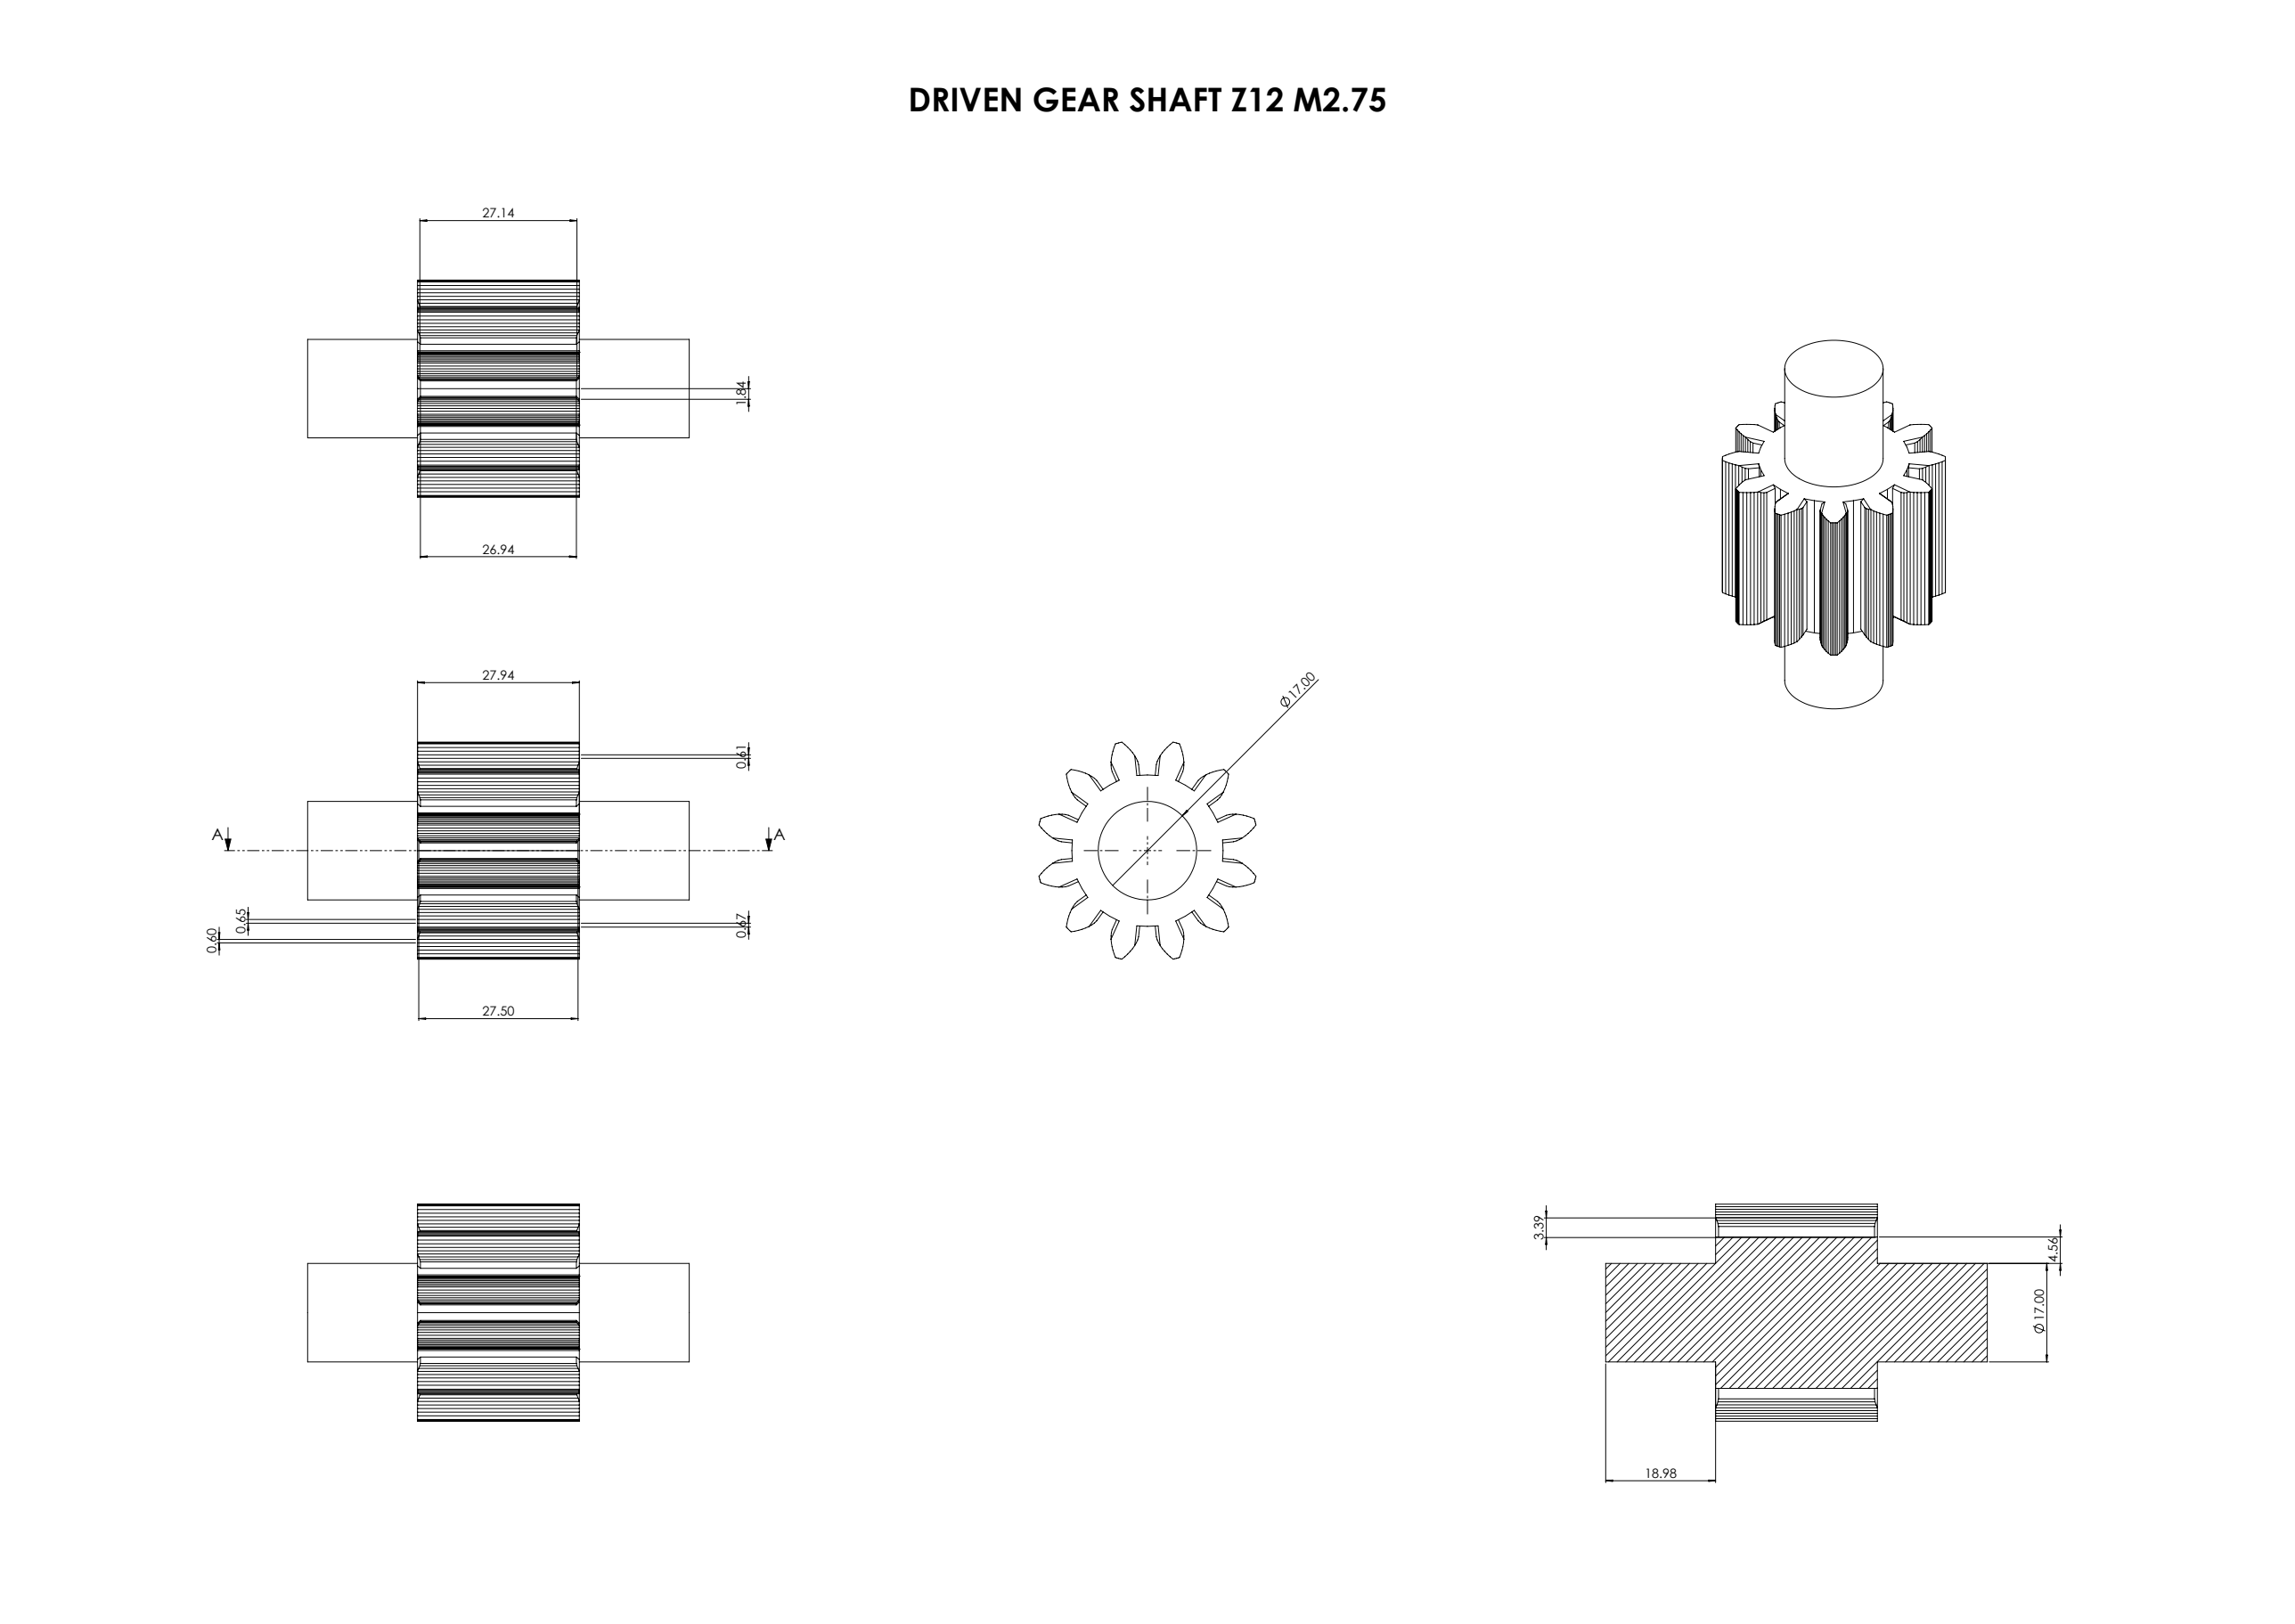
ISO-10303-21;
HEADER;
/* Generated by software containing ST-Developer
 * from STEP Tools, Inc. (www.steptools.com) 
 */

FILE_DESCRIPTION(
/* description */ (''),
/* implementation_level */ '2;1');

FILE_NAME(
/* name */ '05_Driven_Gear_Shaft_z12_m2.75.step',
/* time_stamp */ '2026-10-26T06:59:52-07:00',
/* author */ (''),
/* organization */ (''),
/* preprocessor_version */ 'ST-DEVELOPER v20.2',
/* originating_system */ 'Autodesk Translation Framework v15.15.0.0',
/* authorisation */ '');

FILE_SCHEMA (('AUTOMOTIVE_DESIGN { 1 0 10303 214 3 1 1 }'));
ENDSEC;

DATA;
#10=MECHANICAL_DESIGN_GEOMETRIC_PRESENTATION_REPRESENTATION('',(#168),#46395);
#140=SHAPE_REPRESENTATION_RELATIONSHIP('SRR','None',#46460,#154);
#154=ADVANCED_BREP_SHAPE_REPRESENTATION('',(#182),#46385);
#168=STYLED_ITEM('',(#46596),#182);
#182=MANIFOLD_SOLID_BREP('Body1',#24941);
#517=CYLINDRICAL_SURFACE('',#26404,8.5);
#518=CYLINDRICAL_SURFACE('',#26407,8.5);
#649=FACE_BOUND('',#3798,.T.);
#650=FACE_BOUND('',#3872,.T.);
#1160=PLANE('',#26064);
#1161=PLANE('',#26065);
#1162=PLANE('',#26067);
#1163=PLANE('',#26068);
#1164=PLANE('',#26069);
#1165=PLANE('',#26070);
#1166=PLANE('',#26071);
#1167=PLANE('',#26072);
#1168=PLANE('',#26073);
#1169=PLANE('',#26074);
#1170=PLANE('',#26075);
#1171=PLANE('',#26076);
#1172=PLANE('',#26077);
#1173=PLANE('',#26078);
#1174=PLANE('',#26079);
#1175=PLANE('',#26080);
#1176=PLANE('',#26081);
#1177=PLANE('',#26082);
#1178=PLANE('',#26083);
#1179=PLANE('',#26084);
#1180=PLANE('',#26085);
#1181=PLANE('',#26086);
#1182=PLANE('',#26087);
#1183=PLANE('',#26088);
#1184=PLANE('',#26089);
#1185=PLANE('',#26090);
#1186=PLANE('',#26091);
#1187=PLANE('',#26092);
#1188=PLANE('',#26093);
#1189=PLANE('',#26094);
#1190=PLANE('',#26095);
#1191=PLANE('',#26096);
#1192=PLANE('',#26097);
#1193=PLANE('',#26098);
#1194=PLANE('',#26099);
#1195=PLANE('',#26100);
#1196=PLANE('',#26101);
#1197=PLANE('',#26102);
#1198=PLANE('',#26103);
#1199=PLANE('',#26104);
#1200=PLANE('',#26105);
#1201=PLANE('',#26106);
#1202=PLANE('',#26107);
#1203=PLANE('',#26108);
#1204=PLANE('',#26109);
#1205=PLANE('',#26110);
#1206=PLANE('',#26111);
#1207=PLANE('',#26112);
#1208=PLANE('',#26113);
#1209=PLANE('',#26114);
#1210=PLANE('',#26115);
#1211=PLANE('',#26116);
#1212=PLANE('',#26117);
#1213=PLANE('',#26118);
#1214=PLANE('',#26119);
#1215=PLANE('',#26120);
#1216=PLANE('',#26121);
#1217=PLANE('',#26122);
#1218=PLANE('',#26123);
#1219=PLANE('',#26124);
#1220=PLANE('',#26125);
#1221=PLANE('',#26126);
#1222=PLANE('',#26127);
#1223=PLANE('',#26128);
#1224=PLANE('',#26129);
#1225=PLANE('',#26130);
#1226=PLANE('',#26131);
#1227=PLANE('',#26132);
#1228=PLANE('',#26133);
#1229=PLANE('',#26134);
#1230=PLANE('',#26135);
#1231=PLANE('',#26136);
#1232=PLANE('',#26137);
#1233=PLANE('',#26138);
#1234=PLANE('',#26139);
#1235=PLANE('',#26141);
#1236=PLANE('',#26142);
#1237=PLANE('',#26143);
#1238=PLANE('',#26144);
#1239=PLANE('',#26145);
#1240=PLANE('',#26146);
#1241=PLANE('',#26147);
#1242=PLANE('',#26148);
#1243=PLANE('',#26149);
#1244=PLANE('',#26150);
#1245=PLANE('',#26151);
#1246=PLANE('',#26152);
#1247=PLANE('',#26153);
#1248=PLANE('',#26154);
#1249=PLANE('',#26155);
#1250=PLANE('',#26156);
#1251=PLANE('',#26157);
#1252=PLANE('',#26158);
#1253=PLANE('',#26159);
#1254=PLANE('',#26160);
#1255=PLANE('',#26161);
#1256=PLANE('',#26162);
#1257=PLANE('',#26163);
#1258=PLANE('',#26164);
#1259=PLANE('',#26165);
#1260=PLANE('',#26166);
#1261=PLANE('',#26167);
#1262=PLANE('',#26168);
#1263=PLANE('',#26169);
#1264=PLANE('',#26170);
#1265=PLANE('',#26171);
#1266=PLANE('',#26172);
#1267=PLANE('',#26173);
#1268=PLANE('',#26174);
#1269=PLANE('',#26175);
#1270=PLANE('',#26176);
#1271=PLANE('',#26177);
#1272=PLANE('',#26178);
#1273=PLANE('',#26179);
#1274=PLANE('',#26180);
#1275=PLANE('',#26181);
#1276=PLANE('',#26182);
#1277=PLANE('',#26183);
#1278=PLANE('',#26184);
#1279=PLANE('',#26185);
#1280=PLANE('',#26186);
#1281=PLANE('',#26187);
#1282=PLANE('',#26188);
#1283=PLANE('',#26189);
#1284=PLANE('',#26190);
#1285=PLANE('',#26191);
#1286=PLANE('',#26192);
#1287=PLANE('',#26193);
#1288=PLANE('',#26194);
#1289=PLANE('',#26195);
#1290=PLANE('',#26196);
#1291=PLANE('',#26197);
#1292=PLANE('',#26198);
#1293=PLANE('',#26199);
#1294=PLANE('',#26200);
#1295=PLANE('',#26201);
#1296=PLANE('',#26202);
#1297=PLANE('',#26203);
#1298=PLANE('',#26204);
#1299=PLANE('',#26205);
#1300=PLANE('',#26206);
#1301=PLANE('',#26207);
#1302=PLANE('',#26208);
#1303=PLANE('',#26209);
#1304=PLANE('',#26210);
#1305=PLANE('',#26211);
#1306=PLANE('',#26212);
#1307=PLANE('',#26213);
#1308=PLANE('',#26214);
#1309=PLANE('',#26215);
#1310=PLANE('',#26216);
#1311=PLANE('',#26217);
#1312=PLANE('',#26218);
#1313=PLANE('',#26219);
#1314=PLANE('',#26220);
#1315=PLANE('',#26221);
#1316=PLANE('',#26222);
#1317=PLANE('',#26223);
#1318=PLANE('',#26224);
#1319=PLANE('',#26225);
#1320=PLANE('',#26226);
#1321=PLANE('',#26227);
#1322=PLANE('',#26228);
#1323=PLANE('',#26229);
#1324=PLANE('',#26230);
#1325=PLANE('',#26231);
#1326=PLANE('',#26232);
#1327=PLANE('',#26233);
#1328=PLANE('',#26234);
#1329=PLANE('',#26235);
#1330=PLANE('',#26236);
#1331=PLANE('',#26237);
#1332=PLANE('',#26238);
#1333=PLANE('',#26239);
#1334=PLANE('',#26240);
#1335=PLANE('',#26241);
#1336=PLANE('',#26242);
#1337=PLANE('',#26243);
#1338=PLANE('',#26244);
#1339=PLANE('',#26245);
#1340=PLANE('',#26246);
#1341=PLANE('',#26247);
#1342=PLANE('',#26248);
#1343=PLANE('',#26249);
#1344=PLANE('',#26250);
#1345=PLANE('',#26251);
#1346=PLANE('',#26252);
#1347=PLANE('',#26253);
#1348=PLANE('',#26254);
#1349=PLANE('',#26255);
#1350=PLANE('',#26256);
#1351=PLANE('',#26257);
#1352=PLANE('',#26258);
#1353=PLANE('',#26259);
#1354=PLANE('',#26260);
#1355=PLANE('',#26261);
#1356=PLANE('',#26262);
#1357=PLANE('',#26263);
#1358=PLANE('',#26264);
#1359=PLANE('',#26265);
#1360=PLANE('',#26266);
#1361=PLANE('',#26267);
#1362=PLANE('',#26268);
#1363=PLANE('',#26269);
#1364=PLANE('',#26270);
#1365=PLANE('',#26271);
#1366=PLANE('',#26272);
#1367=PLANE('',#26273);
#1368=PLANE('',#26274);
#1369=PLANE('',#26275);
#1370=PLANE('',#26276);
#1371=PLANE('',#26277);
#1372=PLANE('',#26278);
#1373=PLANE('',#26279);
#1374=PLANE('',#26280);
#1375=PLANE('',#26281);
#1376=PLANE('',#26282);
#1377=PLANE('',#26283);
#1378=PLANE('',#26284);
#1379=PLANE('',#26285);
#1380=PLANE('',#26286);
#1381=PLANE('',#26287);
#1382=PLANE('',#26288);
#1383=PLANE('',#26289);
#1384=PLANE('',#26290);
#1385=PLANE('',#26291);
#1386=PLANE('',#26292);
#1387=PLANE('',#26293);
#1388=PLANE('',#26294);
#1389=PLANE('',#26295);
#1390=PLANE('',#26296);
#1391=PLANE('',#26297);
#1392=PLANE('',#26298);
#1393=PLANE('',#26299);
#1394=PLANE('',#26300);
#1395=PLANE('',#26301);
#1396=PLANE('',#26302);
#1397=PLANE('',#26303);
#1398=PLANE('',#26304);
#1399=PLANE('',#26305);
#1400=PLANE('',#26306);
#1401=PLANE('',#26307);
#1402=PLANE('',#26308);
#1403=PLANE('',#26309);
#1404=PLANE('',#26310);
#1405=PLANE('',#26311);
#1406=PLANE('',#26312);
#1407=PLANE('',#26313);
#1408=PLANE('',#26314);
#1409=PLANE('',#26315);
#1410=PLANE('',#26316);
#1411=PLANE('',#26317);
#1412=PLANE('',#26318);
#1413=PLANE('',#26319);
#1414=PLANE('',#26320);
#1415=PLANE('',#26321);
#1416=PLANE('',#26322);
#1417=PLANE('',#26323);
#1418=PLANE('',#26324);
#1419=PLANE('',#26325);
#1420=PLANE('',#26326);
#1421=PLANE('',#26327);
#1422=PLANE('',#26328);
#1423=PLANE('',#26329);
#1424=PLANE('',#26330);
#1425=PLANE('',#26331);
#1426=PLANE('',#26332);
#1427=PLANE('',#26333);
#1428=PLANE('',#26334);
#1429=PLANE('',#26335);
#1430=PLANE('',#26336);
#1431=PLANE('',#26337);
#1432=PLANE('',#26338);
#1433=PLANE('',#26339);
#1434=PLANE('',#26340);
#1435=PLANE('',#26341);
#1436=PLANE('',#26342);
#1437=PLANE('',#26343);
#1438=PLANE('',#26344);
#1439=PLANE('',#26345);
#1440=PLANE('',#26346);
#1441=PLANE('',#26347);
#1442=PLANE('',#26348);
#1443=PLANE('',#26349);
#1444=PLANE('',#26350);
#1445=PLANE('',#26351);
#1446=PLANE('',#26352);
#1447=PLANE('',#26353);
#1448=PLANE('',#26354);
#1449=PLANE('',#26355);
#1450=PLANE('',#26356);
#1451=PLANE('',#26357);
#1452=PLANE('',#26358);
#1453=PLANE('',#26359);
#1454=PLANE('',#26360);
#1455=PLANE('',#26361);
#1456=PLANE('',#26362);
#1457=PLANE('',#26363);
#1458=PLANE('',#26364);
#1459=PLANE('',#26365);
#1460=PLANE('',#26366);
#1461=PLANE('',#26367);
#1462=PLANE('',#26368);
#1463=PLANE('',#26369);
#1464=PLANE('',#26370);
#1465=PLANE('',#26371);
#1466=PLANE('',#26372);
#1467=PLANE('',#26373);
#1468=PLANE('',#26374);
#1469=PLANE('',#26375);
#1470=PLANE('',#26376);
#1471=PLANE('',#26377);
#1472=PLANE('',#26378);
#1473=PLANE('',#26379);
#1474=PLANE('',#26380);
#1475=PLANE('',#26381);
#1476=PLANE('',#26382);
#1477=PLANE('',#26383);
#1478=PLANE('',#26384);
#1479=PLANE('',#26385);
#1480=PLANE('',#26386);
#1481=PLANE('',#26387);
#1482=PLANE('',#26388);
#1483=PLANE('',#26389);
#1484=PLANE('',#26390);
#1485=PLANE('',#26391);
#1486=PLANE('',#26392);
#1487=PLANE('',#26393);
#1488=PLANE('',#26394);
#1489=PLANE('',#26395);
#1490=PLANE('',#26396);
#1491=PLANE('',#26397);
#1492=PLANE('',#26398);
#1493=PLANE('',#26399);
#1494=PLANE('',#26400);
#1495=PLANE('',#26401);
#1496=PLANE('',#26402);
#1497=PLANE('',#26403);
#1498=PLANE('',#26406);
#1499=PLANE('',#26409);
#2402=FACE_OUTER_BOUND('',#3796,.T.);
#2403=FACE_OUTER_BOUND('',#3797,.T.);
#2404=FACE_OUTER_BOUND('',#3799,.T.);
#2405=FACE_OUTER_BOUND('',#3800,.T.);
#2406=FACE_OUTER_BOUND('',#3801,.T.);
#2407=FACE_OUTER_BOUND('',#3802,.T.);
#2408=FACE_OUTER_BOUND('',#3803,.T.);
#2409=FACE_OUTER_BOUND('',#3804,.T.);
#2410=FACE_OUTER_BOUND('',#3805,.T.);
#2411=FACE_OUTER_BOUND('',#3806,.T.);
#2412=FACE_OUTER_BOUND('',#3807,.T.);
#2413=FACE_OUTER_BOUND('',#3808,.T.);
#2414=FACE_OUTER_BOUND('',#3809,.T.);
#2415=FACE_OUTER_BOUND('',#3810,.T.);
#2416=FACE_OUTER_BOUND('',#3811,.T.);
#2417=FACE_OUTER_BOUND('',#3812,.T.);
#2418=FACE_OUTER_BOUND('',#3813,.T.);
#2419=FACE_OUTER_BOUND('',#3814,.T.);
#2420=FACE_OUTER_BOUND('',#3815,.T.);
#2421=FACE_OUTER_BOUND('',#3816,.T.);
#2422=FACE_OUTER_BOUND('',#3817,.T.);
#2423=FACE_OUTER_BOUND('',#3818,.T.);
#2424=FACE_OUTER_BOUND('',#3819,.T.);
#2425=FACE_OUTER_BOUND('',#3820,.T.);
#2426=FACE_OUTER_BOUND('',#3821,.T.);
#2427=FACE_OUTER_BOUND('',#3822,.T.);
#2428=FACE_OUTER_BOUND('',#3823,.T.);
#2429=FACE_OUTER_BOUND('',#3824,.T.);
#2430=FACE_OUTER_BOUND('',#3825,.T.);
#2431=FACE_OUTER_BOUND('',#3826,.T.);
#2432=FACE_OUTER_BOUND('',#3827,.T.);
#2433=FACE_OUTER_BOUND('',#3828,.T.);
#2434=FACE_OUTER_BOUND('',#3829,.T.);
#2435=FACE_OUTER_BOUND('',#3830,.T.);
#2436=FACE_OUTER_BOUND('',#3831,.T.);
#2437=FACE_OUTER_BOUND('',#3832,.T.);
#2438=FACE_OUTER_BOUND('',#3833,.T.);
#2439=FACE_OUTER_BOUND('',#3834,.T.);
#2440=FACE_OUTER_BOUND('',#3835,.T.);
#2441=FACE_OUTER_BOUND('',#3836,.T.);
#2442=FACE_OUTER_BOUND('',#3837,.T.);
#2443=FACE_OUTER_BOUND('',#3838,.T.);
#2444=FACE_OUTER_BOUND('',#3839,.T.);
#2445=FACE_OUTER_BOUND('',#3840,.T.);
#2446=FACE_OUTER_BOUND('',#3841,.T.);
#2447=FACE_OUTER_BOUND('',#3842,.T.);
#2448=FACE_OUTER_BOUND('',#3843,.T.);
#2449=FACE_OUTER_BOUND('',#3844,.T.);
#2450=FACE_OUTER_BOUND('',#3845,.T.);
#2451=FACE_OUTER_BOUND('',#3846,.T.);
#2452=FACE_OUTER_BOUND('',#3847,.T.);
#2453=FACE_OUTER_BOUND('',#3848,.T.);
#2454=FACE_OUTER_BOUND('',#3849,.T.);
#2455=FACE_OUTER_BOUND('',#3850,.T.);
#2456=FACE_OUTER_BOUND('',#3851,.T.);
#2457=FACE_OUTER_BOUND('',#3852,.T.);
#2458=FACE_OUTER_BOUND('',#3853,.T.);
#2459=FACE_OUTER_BOUND('',#3854,.T.);
#2460=FACE_OUTER_BOUND('',#3855,.T.);
#2461=FACE_OUTER_BOUND('',#3856,.T.);
#2462=FACE_OUTER_BOUND('',#3857,.T.);
#2463=FACE_OUTER_BOUND('',#3858,.T.);
#2464=FACE_OUTER_BOUND('',#3859,.T.);
#2465=FACE_OUTER_BOUND('',#3860,.T.);
#2466=FACE_OUTER_BOUND('',#3861,.T.);
#2467=FACE_OUTER_BOUND('',#3862,.T.);
#2468=FACE_OUTER_BOUND('',#3863,.T.);
#2469=FACE_OUTER_BOUND('',#3864,.T.);
#2470=FACE_OUTER_BOUND('',#3865,.T.);
#2471=FACE_OUTER_BOUND('',#3866,.T.);
#2472=FACE_OUTER_BOUND('',#3867,.T.);
#2473=FACE_OUTER_BOUND('',#3868,.T.);
#2474=FACE_OUTER_BOUND('',#3869,.T.);
#2475=FACE_OUTER_BOUND('',#3870,.T.);
#2476=FACE_OUTER_BOUND('',#3871,.T.);
#2477=FACE_OUTER_BOUND('',#3873,.T.);
#2478=FACE_OUTER_BOUND('',#3874,.T.);
#2479=FACE_OUTER_BOUND('',#3875,.T.);
#2480=FACE_OUTER_BOUND('',#3876,.T.);
#2481=FACE_OUTER_BOUND('',#3877,.T.);
#2482=FACE_OUTER_BOUND('',#3878,.T.);
#2483=FACE_OUTER_BOUND('',#3879,.T.);
#2484=FACE_OUTER_BOUND('',#3880,.T.);
#2485=FACE_OUTER_BOUND('',#3881,.T.);
#2486=FACE_OUTER_BOUND('',#3882,.T.);
#2487=FACE_OUTER_BOUND('',#3883,.T.);
#2488=FACE_OUTER_BOUND('',#3884,.T.);
#2489=FACE_OUTER_BOUND('',#3885,.T.);
#2490=FACE_OUTER_BOUND('',#3886,.T.);
#2491=FACE_OUTER_BOUND('',#3887,.T.);
#2492=FACE_OUTER_BOUND('',#3888,.T.);
#2493=FACE_OUTER_BOUND('',#3889,.T.);
#2494=FACE_OUTER_BOUND('',#3890,.T.);
#2495=FACE_OUTER_BOUND('',#3891,.T.);
#2496=FACE_OUTER_BOUND('',#3892,.T.);
#2497=FACE_OUTER_BOUND('',#3893,.T.);
#2498=FACE_OUTER_BOUND('',#3894,.T.);
#2499=FACE_OUTER_BOUND('',#3895,.T.);
#2500=FACE_OUTER_BOUND('',#3896,.T.);
#2501=FACE_OUTER_BOUND('',#3897,.T.);
#2502=FACE_OUTER_BOUND('',#3898,.T.);
#2503=FACE_OUTER_BOUND('',#3899,.T.);
#2504=FACE_OUTER_BOUND('',#3900,.T.);
#2505=FACE_OUTER_BOUND('',#3901,.T.);
#2506=FACE_OUTER_BOUND('',#3902,.T.);
#2507=FACE_OUTER_BOUND('',#3903,.T.);
#2508=FACE_OUTER_BOUND('',#3904,.T.);
#2509=FACE_OUTER_BOUND('',#3905,.T.);
#2510=FACE_OUTER_BOUND('',#3906,.T.);
#2511=FACE_OUTER_BOUND('',#3907,.T.);
#2512=FACE_OUTER_BOUND('',#3908,.T.);
#2513=FACE_OUTER_BOUND('',#3909,.T.);
#2514=FACE_OUTER_BOUND('',#3910,.T.);
#2515=FACE_OUTER_BOUND('',#3911,.T.);
#2516=FACE_OUTER_BOUND('',#3912,.T.);
#2517=FACE_OUTER_BOUND('',#3913,.T.);
#2518=FACE_OUTER_BOUND('',#3914,.T.);
#2519=FACE_OUTER_BOUND('',#3915,.T.);
#2520=FACE_OUTER_BOUND('',#3916,.T.);
#2521=FACE_OUTER_BOUND('',#3917,.T.);
#2522=FACE_OUTER_BOUND('',#3918,.T.);
#2523=FACE_OUTER_BOUND('',#3919,.T.);
#2524=FACE_OUTER_BOUND('',#3920,.T.);
#2525=FACE_OUTER_BOUND('',#3921,.T.);
#2526=FACE_OUTER_BOUND('',#3922,.T.);
#2527=FACE_OUTER_BOUND('',#3923,.T.);
#2528=FACE_OUTER_BOUND('',#3924,.T.);
#2529=FACE_OUTER_BOUND('',#3925,.T.);
#2530=FACE_OUTER_BOUND('',#3926,.T.);
#2531=FACE_OUTER_BOUND('',#3927,.T.);
#2532=FACE_OUTER_BOUND('',#3928,.T.);
#2533=FACE_OUTER_BOUND('',#3929,.T.);
#2534=FACE_OUTER_BOUND('',#3930,.T.);
#2535=FACE_OUTER_BOUND('',#3931,.T.);
#2536=FACE_OUTER_BOUND('',#3932,.T.);
#2537=FACE_OUTER_BOUND('',#3933,.T.);
#2538=FACE_OUTER_BOUND('',#3934,.T.);
#2539=FACE_OUTER_BOUND('',#3935,.T.);
#2540=FACE_OUTER_BOUND('',#3936,.T.);
#2541=FACE_OUTER_BOUND('',#3937,.T.);
#2542=FACE_OUTER_BOUND('',#3938,.T.);
#2543=FACE_OUTER_BOUND('',#3939,.T.);
#2544=FACE_OUTER_BOUND('',#3940,.T.);
#2545=FACE_OUTER_BOUND('',#3941,.T.);
#2546=FACE_OUTER_BOUND('',#3942,.T.);
#2547=FACE_OUTER_BOUND('',#3943,.T.);
#2548=FACE_OUTER_BOUND('',#3944,.T.);
#2549=FACE_OUTER_BOUND('',#3945,.T.);
#2550=FACE_OUTER_BOUND('',#3946,.T.);
#2551=FACE_OUTER_BOUND('',#3947,.T.);
#2552=FACE_OUTER_BOUND('',#3948,.T.);
#2553=FACE_OUTER_BOUND('',#3949,.T.);
#2554=FACE_OUTER_BOUND('',#3950,.T.);
#2555=FACE_OUTER_BOUND('',#3951,.T.);
#2556=FACE_OUTER_BOUND('',#3952,.T.);
#2557=FACE_OUTER_BOUND('',#3953,.T.);
#2558=FACE_OUTER_BOUND('',#3954,.T.);
#2559=FACE_OUTER_BOUND('',#3955,.T.);
#2560=FACE_OUTER_BOUND('',#3956,.T.);
#2561=FACE_OUTER_BOUND('',#3957,.T.);
#2562=FACE_OUTER_BOUND('',#3958,.T.);
#2563=FACE_OUTER_BOUND('',#3959,.T.);
#2564=FACE_OUTER_BOUND('',#3960,.T.);
#2565=FACE_OUTER_BOUND('',#3961,.T.);
#2566=FACE_OUTER_BOUND('',#3962,.T.);
#2567=FACE_OUTER_BOUND('',#3963,.T.);
#2568=FACE_OUTER_BOUND('',#3964,.T.);
#2569=FACE_OUTER_BOUND('',#3965,.T.);
#2570=FACE_OUTER_BOUND('',#3966,.T.);
#2571=FACE_OUTER_BOUND('',#3967,.T.);
#2572=FACE_OUTER_BOUND('',#3968,.T.);
#2573=FACE_OUTER_BOUND('',#3969,.T.);
#2574=FACE_OUTER_BOUND('',#3970,.T.);
#2575=FACE_OUTER_BOUND('',#3971,.T.);
#2576=FACE_OUTER_BOUND('',#3972,.T.);
#2577=FACE_OUTER_BOUND('',#3973,.T.);
#2578=FACE_OUTER_BOUND('',#3974,.T.);
#2579=FACE_OUTER_BOUND('',#3975,.T.);
#2580=FACE_OUTER_BOUND('',#3976,.T.);
#2581=FACE_OUTER_BOUND('',#3977,.T.);
#2582=FACE_OUTER_BOUND('',#3978,.T.);
#2583=FACE_OUTER_BOUND('',#3979,.T.);
#2584=FACE_OUTER_BOUND('',#3980,.T.);
#2585=FACE_OUTER_BOUND('',#3981,.T.);
#2586=FACE_OUTER_BOUND('',#3982,.T.);
#2587=FACE_OUTER_BOUND('',#3983,.T.);
#2588=FACE_OUTER_BOUND('',#3984,.T.);
#2589=FACE_OUTER_BOUND('',#3985,.T.);
#2590=FACE_OUTER_BOUND('',#3986,.T.);
#2591=FACE_OUTER_BOUND('',#3987,.T.);
#2592=FACE_OUTER_BOUND('',#3988,.T.);
#2593=FACE_OUTER_BOUND('',#3989,.T.);
#2594=FACE_OUTER_BOUND('',#3990,.T.);
#2595=FACE_OUTER_BOUND('',#3991,.T.);
#2596=FACE_OUTER_BOUND('',#3992,.T.);
#2597=FACE_OUTER_BOUND('',#3993,.T.);
#2598=FACE_OUTER_BOUND('',#3994,.T.);
#2599=FACE_OUTER_BOUND('',#3995,.T.);
#2600=FACE_OUTER_BOUND('',#3996,.T.);
#2601=FACE_OUTER_BOUND('',#3997,.T.);
#2602=FACE_OUTER_BOUND('',#3998,.T.);
#2603=FACE_OUTER_BOUND('',#3999,.T.);
#2604=FACE_OUTER_BOUND('',#4000,.T.);
#2605=FACE_OUTER_BOUND('',#4001,.T.);
#2606=FACE_OUTER_BOUND('',#4002,.T.);
#2607=FACE_OUTER_BOUND('',#4003,.T.);
#2608=FACE_OUTER_BOUND('',#4004,.T.);
#2609=FACE_OUTER_BOUND('',#4005,.T.);
#2610=FACE_OUTER_BOUND('',#4006,.T.);
#2611=FACE_OUTER_BOUND('',#4007,.T.);
#2612=FACE_OUTER_BOUND('',#4008,.T.);
#2613=FACE_OUTER_BOUND('',#4009,.T.);
#2614=FACE_OUTER_BOUND('',#4010,.T.);
#2615=FACE_OUTER_BOUND('',#4011,.T.);
#2616=FACE_OUTER_BOUND('',#4012,.T.);
#2617=FACE_OUTER_BOUND('',#4013,.T.);
#2618=FACE_OUTER_BOUND('',#4014,.T.);
#2619=FACE_OUTER_BOUND('',#4015,.T.);
#2620=FACE_OUTER_BOUND('',#4016,.T.);
#2621=FACE_OUTER_BOUND('',#4017,.T.);
#2622=FACE_OUTER_BOUND('',#4018,.T.);
#2623=FACE_OUTER_BOUND('',#4019,.T.);
#2624=FACE_OUTER_BOUND('',#4020,.T.);
#2625=FACE_OUTER_BOUND('',#4021,.T.);
#2626=FACE_OUTER_BOUND('',#4022,.T.);
#2627=FACE_OUTER_BOUND('',#4023,.T.);
#2628=FACE_OUTER_BOUND('',#4024,.T.);
#2629=FACE_OUTER_BOUND('',#4025,.T.);
#2630=FACE_OUTER_BOUND('',#4026,.T.);
#2631=FACE_OUTER_BOUND('',#4027,.T.);
#2632=FACE_OUTER_BOUND('',#4028,.T.);
#2633=FACE_OUTER_BOUND('',#4029,.T.);
#2634=FACE_OUTER_BOUND('',#4030,.T.);
#2635=FACE_OUTER_BOUND('',#4031,.T.);
#2636=FACE_OUTER_BOUND('',#4032,.T.);
#2637=FACE_OUTER_BOUND('',#4033,.T.);
#2638=FACE_OUTER_BOUND('',#4034,.T.);
#2639=FACE_OUTER_BOUND('',#4035,.T.);
#2640=FACE_OUTER_BOUND('',#4036,.T.);
#2641=FACE_OUTER_BOUND('',#4037,.T.);
#2642=FACE_OUTER_BOUND('',#4038,.T.);
#2643=FACE_OUTER_BOUND('',#4039,.T.);
#2644=FACE_OUTER_BOUND('',#4040,.T.);
#2645=FACE_OUTER_BOUND('',#4041,.T.);
#2646=FACE_OUTER_BOUND('',#4042,.T.);
#2647=FACE_OUTER_BOUND('',#4043,.T.);
#2648=FACE_OUTER_BOUND('',#4044,.T.);
#2649=FACE_OUTER_BOUND('',#4045,.T.);
#2650=FACE_OUTER_BOUND('',#4046,.T.);
#2651=FACE_OUTER_BOUND('',#4047,.T.);
#2652=FACE_OUTER_BOUND('',#4048,.T.);
#2653=FACE_OUTER_BOUND('',#4049,.T.);
#2654=FACE_OUTER_BOUND('',#4050,.T.);
#2655=FACE_OUTER_BOUND('',#4051,.T.);
#2656=FACE_OUTER_BOUND('',#4052,.T.);
#2657=FACE_OUTER_BOUND('',#4053,.T.);
#2658=FACE_OUTER_BOUND('',#4054,.T.);
#2659=FACE_OUTER_BOUND('',#4055,.T.);
#2660=FACE_OUTER_BOUND('',#4056,.T.);
#2661=FACE_OUTER_BOUND('',#4057,.T.);
#2662=FACE_OUTER_BOUND('',#4058,.T.);
#2663=FACE_OUTER_BOUND('',#4059,.T.);
#2664=FACE_OUTER_BOUND('',#4060,.T.);
#2665=FACE_OUTER_BOUND('',#4061,.T.);
#2666=FACE_OUTER_BOUND('',#4062,.T.);
#2667=FACE_OUTER_BOUND('',#4063,.T.);
#2668=FACE_OUTER_BOUND('',#4064,.T.);
#2669=FACE_OUTER_BOUND('',#4065,.T.);
#2670=FACE_OUTER_BOUND('',#4066,.T.);
#2671=FACE_OUTER_BOUND('',#4067,.T.);
#2672=FACE_OUTER_BOUND('',#4068,.T.);
#2673=FACE_OUTER_BOUND('',#4069,.T.);
#2674=FACE_OUTER_BOUND('',#4070,.T.);
#2675=FACE_OUTER_BOUND('',#4071,.T.);
#2676=FACE_OUTER_BOUND('',#4072,.T.);
#2677=FACE_OUTER_BOUND('',#4073,.T.);
#2678=FACE_OUTER_BOUND('',#4074,.T.);
#2679=FACE_OUTER_BOUND('',#4075,.T.);
#2680=FACE_OUTER_BOUND('',#4076,.T.);
#2681=FACE_OUTER_BOUND('',#4077,.T.);
#2682=FACE_OUTER_BOUND('',#4078,.T.);
#2683=FACE_OUTER_BOUND('',#4079,.T.);
#2684=FACE_OUTER_BOUND('',#4080,.T.);
#2685=FACE_OUTER_BOUND('',#4081,.T.);
#2686=FACE_OUTER_BOUND('',#4082,.T.);
#2687=FACE_OUTER_BOUND('',#4083,.T.);
#2688=FACE_OUTER_BOUND('',#4084,.T.);
#2689=FACE_OUTER_BOUND('',#4085,.T.);
#2690=FACE_OUTER_BOUND('',#4086,.T.);
#2691=FACE_OUTER_BOUND('',#4087,.T.);
#2692=FACE_OUTER_BOUND('',#4088,.T.);
#2693=FACE_OUTER_BOUND('',#4089,.T.);
#2694=FACE_OUTER_BOUND('',#4090,.T.);
#2695=FACE_OUTER_BOUND('',#4091,.T.);
#2696=FACE_OUTER_BOUND('',#4092,.T.);
#2697=FACE_OUTER_BOUND('',#4093,.T.);
#2698=FACE_OUTER_BOUND('',#4094,.T.);
#2699=FACE_OUTER_BOUND('',#4095,.T.);
#2700=FACE_OUTER_BOUND('',#4096,.T.);
#2701=FACE_OUTER_BOUND('',#4097,.T.);
#2702=FACE_OUTER_BOUND('',#4098,.T.);
#2703=FACE_OUTER_BOUND('',#4099,.T.);
#2704=FACE_OUTER_BOUND('',#4100,.T.);
#2705=FACE_OUTER_BOUND('',#4101,.T.);
#2706=FACE_OUTER_BOUND('',#4102,.T.);
#2707=FACE_OUTER_BOUND('',#4103,.T.);
#2708=FACE_OUTER_BOUND('',#4104,.T.);
#2709=FACE_OUTER_BOUND('',#4105,.T.);
#2710=FACE_OUTER_BOUND('',#4106,.T.);
#2711=FACE_OUTER_BOUND('',#4107,.T.);
#2712=FACE_OUTER_BOUND('',#4108,.T.);
#2713=FACE_OUTER_BOUND('',#4109,.T.);
#2714=FACE_OUTER_BOUND('',#4110,.T.);
#2715=FACE_OUTER_BOUND('',#4111,.T.);
#2716=FACE_OUTER_BOUND('',#4112,.T.);
#2717=FACE_OUTER_BOUND('',#4113,.T.);
#2718=FACE_OUTER_BOUND('',#4114,.T.);
#2719=FACE_OUTER_BOUND('',#4115,.T.);
#2720=FACE_OUTER_BOUND('',#4116,.T.);
#2721=FACE_OUTER_BOUND('',#4117,.T.);
#2722=FACE_OUTER_BOUND('',#4118,.T.);
#2723=FACE_OUTER_BOUND('',#4119,.T.);
#2724=FACE_OUTER_BOUND('',#4120,.T.);
#2725=FACE_OUTER_BOUND('',#4121,.T.);
#2726=FACE_OUTER_BOUND('',#4122,.T.);
#2727=FACE_OUTER_BOUND('',#4123,.T.);
#2728=FACE_OUTER_BOUND('',#4124,.T.);
#2729=FACE_OUTER_BOUND('',#4125,.T.);
#2730=FACE_OUTER_BOUND('',#4126,.T.);
#2731=FACE_OUTER_BOUND('',#4127,.T.);
#2732=FACE_OUTER_BOUND('',#4128,.T.);
#2733=FACE_OUTER_BOUND('',#4129,.T.);
#2734=FACE_OUTER_BOUND('',#4130,.T.);
#2735=FACE_OUTER_BOUND('',#4131,.T.);
#2736=FACE_OUTER_BOUND('',#4132,.T.);
#2737=FACE_OUTER_BOUND('',#4133,.T.);
#2738=FACE_OUTER_BOUND('',#4134,.T.);
#2739=FACE_OUTER_BOUND('',#4135,.T.);
#2740=FACE_OUTER_BOUND('',#4136,.T.);
#2741=FACE_OUTER_BOUND('',#4137,.T.);
#2742=FACE_OUTER_BOUND('',#4138,.T.);
#2743=FACE_OUTER_BOUND('',#4139,.T.);
#3796=EDGE_LOOP('',(#19988,#19989,#19990,#19991,#19992,#19993));
#3797=EDGE_LOOP('',(#19994,#19995,#19996,#19997,#19998,#19999,#20000,#20001,
#20002,#20003,#20004,#20005,#20006,#20007,#20008,#20009,#20010,#20011,#20012,
#20013,#20014,#20015,#20016,#20017,#20018,#20019,#20020,#20021,#20022,#20023,
#20024,#20025,#20026,#20027,#20028,#20029,#20030,#20031,#20032,#20033,#20034,
#20035,#20036,#20037,#20038,#20039,#20040,#20041,#20042,#20043,#20044,#20045,
#20046,#20047,#20048,#20049,#20050,#20051,#20052,#20053,#20054,#20055,#20056,
#20057,#20058,#20059,#20060,#20061,#20062,#20063,#20064,#20065,#20066,#20067,
#20068,#20069,#20070,#20071,#20072,#20073,#20074,#20075,#20076,#20077,#20078,
#20079,#20080,#20081,#20082,#20083,#20084,#20085,#20086,#20087,#20088,#20089,
#20090,#20091,#20092,#20093,#20094,#20095,#20096,#20097,#20098,#20099,#20100,
#20101,#20102,#20103,#20104,#20105,#20106,#20107,#20108,#20109,#20110,#20111,
#20112,#20113,#20114,#20115,#20116,#20117,#20118,#20119,#20120,#20121,#20122,
#20123,#20124,#20125,#20126,#20127,#20128,#20129,#20130,#20131,#20132,#20133,
#20134,#20135,#20136,#20137,#20138,#20139,#20140,#20141,#20142,#20143,#20144,
#20145,#20146,#20147,#20148,#20149,#20150,#20151,#20152,#20153,#20154,#20155,
#20156,#20157,#20158,#20159,#20160,#20161,#20162,#20163,#20164,#20165,#20166,
#20167,#20168,#20169,#20170,#20171,#20172,#20173,#20174,#20175,#20176,#20177,
#20178,#20179,#20180,#20181,#20182,#20183,#20184,#20185,#20186,#20187,#20188,
#20189,#20190,#20191,#20192,#20193,#20194,#20195,#20196,#20197,#20198,#20199,
#20200,#20201,#20202,#20203,#20204,#20205,#20206,#20207,#20208,#20209,#20210,
#20211,#20212,#20213,#20214,#20215,#20216,#20217,#20218,#20219,#20220,#20221,
#20222,#20223,#20224,#20225,#20226,#20227,#20228,#20229,#20230,#20231,#20232,
#20233));
#3798=EDGE_LOOP('',(#20234));
#3799=EDGE_LOOP('',(#20235,#20236,#20237,#20238,#20239,#20240));
#3800=EDGE_LOOP('',(#20241,#20242,#20243,#20244));
#3801=EDGE_LOOP('',(#20245,#20246,#20247,#20248,#20249,#20250));
#3802=EDGE_LOOP('',(#20251,#20252,#20253,#20254,#20255,#20256));
#3803=EDGE_LOOP('',(#20257,#20258,#20259,#20260));
#3804=EDGE_LOOP('',(#20261,#20262,#20263,#20264,#20265,#20266));
#3805=EDGE_LOOP('',(#20267,#20268,#20269,#20270,#20271,#20272));
#3806=EDGE_LOOP('',(#20273,#20274,#20275,#20276));
#3807=EDGE_LOOP('',(#20277,#20278,#20279,#20280,#20281,#20282));
#3808=EDGE_LOOP('',(#20283,#20284,#20285,#20286,#20287,#20288));
#3809=EDGE_LOOP('',(#20289,#20290,#20291,#20292));
#3810=EDGE_LOOP('',(#20293,#20294,#20295,#20296,#20297,#20298));
#3811=EDGE_LOOP('',(#20299,#20300,#20301,#20302,#20303,#20304));
#3812=EDGE_LOOP('',(#20305,#20306,#20307,#20308));
#3813=EDGE_LOOP('',(#20309,#20310,#20311,#20312,#20313,#20314));
#3814=EDGE_LOOP('',(#20315,#20316,#20317,#20318,#20319,#20320));
#3815=EDGE_LOOP('',(#20321,#20322,#20323,#20324));
#3816=EDGE_LOOP('',(#20325,#20326,#20327,#20328,#20329,#20330));
#3817=EDGE_LOOP('',(#20331,#20332,#20333,#20334,#20335,#20336));
#3818=EDGE_LOOP('',(#20337,#20338,#20339,#20340));
#3819=EDGE_LOOP('',(#20341,#20342,#20343,#20344,#20345,#20346));
#3820=EDGE_LOOP('',(#20347,#20348,#20349,#20350,#20351,#20352));
#3821=EDGE_LOOP('',(#20353,#20354,#20355,#20356));
#3822=EDGE_LOOP('',(#20357,#20358,#20359,#20360,#20361,#20362));
#3823=EDGE_LOOP('',(#20363,#20364,#20365,#20366,#20367,#20368));
#3824=EDGE_LOOP('',(#20369,#20370,#20371,#20372));
#3825=EDGE_LOOP('',(#20373,#20374,#20375,#20376,#20377,#20378));
#3826=EDGE_LOOP('',(#20379,#20380,#20381,#20382,#20383,#20384));
#3827=EDGE_LOOP('',(#20385,#20386,#20387,#20388));
#3828=EDGE_LOOP('',(#20389,#20390,#20391,#20392,#20393,#20394));
#3829=EDGE_LOOP('',(#20395,#20396,#20397,#20398,#20399,#20400));
#3830=EDGE_LOOP('',(#20401,#20402,#20403,#20404));
#3831=EDGE_LOOP('',(#20405,#20406,#20407,#20408,#20409,#20410));
#3832=EDGE_LOOP('',(#20411,#20412,#20413,#20414,#20415,#20416));
#3833=EDGE_LOOP('',(#20417,#20418,#20419,#20420));
#3834=EDGE_LOOP('',(#20421,#20422,#20423,#20424,#20425,#20426));
#3835=EDGE_LOOP('',(#20427,#20428,#20429,#20430));
#3836=EDGE_LOOP('',(#20431,#20432,#20433,#20434));
#3837=EDGE_LOOP('',(#20435,#20436,#20437,#20438,#20439,#20440));
#3838=EDGE_LOOP('',(#20441,#20442,#20443,#20444));
#3839=EDGE_LOOP('',(#20445,#20446,#20447,#20448));
#3840=EDGE_LOOP('',(#20449,#20450,#20451,#20452,#20453,#20454));
#3841=EDGE_LOOP('',(#20455,#20456,#20457,#20458));
#3842=EDGE_LOOP('',(#20459,#20460,#20461,#20462));
#3843=EDGE_LOOP('',(#20463,#20464,#20465,#20466,#20467,#20468));
#3844=EDGE_LOOP('',(#20469,#20470,#20471,#20472));
#3845=EDGE_LOOP('',(#20473,#20474,#20475,#20476));
#3846=EDGE_LOOP('',(#20477,#20478,#20479,#20480,#20481,#20482));
#3847=EDGE_LOOP('',(#20483,#20484,#20485,#20486));
#3848=EDGE_LOOP('',(#20487,#20488,#20489,#20490));
#3849=EDGE_LOOP('',(#20491,#20492,#20493,#20494,#20495,#20496));
#3850=EDGE_LOOP('',(#20497,#20498,#20499,#20500));
#3851=EDGE_LOOP('',(#20501,#20502,#20503,#20504));
#3852=EDGE_LOOP('',(#20505,#20506,#20507,#20508,#20509,#20510));
#3853=EDGE_LOOP('',(#20511,#20512,#20513,#20514));
#3854=EDGE_LOOP('',(#20515,#20516,#20517,#20518));
#3855=EDGE_LOOP('',(#20519,#20520,#20521,#20522,#20523,#20524));
#3856=EDGE_LOOP('',(#20525,#20526,#20527,#20528));
#3857=EDGE_LOOP('',(#20529,#20530,#20531,#20532));
#3858=EDGE_LOOP('',(#20533,#20534,#20535,#20536,#20537,#20538));
#3859=EDGE_LOOP('',(#20539,#20540,#20541,#20542));
#3860=EDGE_LOOP('',(#20543,#20544,#20545,#20546));
#3861=EDGE_LOOP('',(#20547,#20548,#20549,#20550,#20551,#20552));
#3862=EDGE_LOOP('',(#20553,#20554,#20555,#20556));
#3863=EDGE_LOOP('',(#20557,#20558,#20559,#20560));
#3864=EDGE_LOOP('',(#20561,#20562,#20563,#20564,#20565,#20566));
#3865=EDGE_LOOP('',(#20567,#20568,#20569,#20570));
#3866=EDGE_LOOP('',(#20571,#20572,#20573,#20574));
#3867=EDGE_LOOP('',(#20575,#20576,#20577,#20578,#20579,#20580));
#3868=EDGE_LOOP('',(#20581,#20582,#20583,#20584));
#3869=EDGE_LOOP('',(#20585,#20586,#20587,#20588));
#3870=EDGE_LOOP('',(#20589,#20590,#20591,#20592,#20593,#20594));
#3871=EDGE_LOOP('',(#20595,#20596,#20597,#20598,#20599,#20600,#20601,#20602,
#20603,#20604,#20605,#20606,#20607,#20608,#20609,#20610,#20611,#20612,#20613,
#20614,#20615,#20616,#20617,#20618,#20619,#20620,#20621,#20622,#20623,#20624,
#20625,#20626,#20627,#20628,#20629,#20630,#20631,#20632,#20633,#20634,#20635,
#20636,#20637,#20638,#20639,#20640,#20641,#20642,#20643,#20644,#20645,#20646,
#20647,#20648,#20649,#20650,#20651,#20652,#20653,#20654,#20655,#20656,#20657,
#20658,#20659,#20660,#20661,#20662,#20663,#20664,#20665,#20666,#20667,#20668,
#20669,#20670,#20671,#20672,#20673,#20674,#20675,#20676,#20677,#20678,#20679,
#20680,#20681,#20682,#20683,#20684,#20685,#20686,#20687,#20688,#20689,#20690,
#20691,#20692,#20693,#20694,#20695,#20696,#20697,#20698,#20699,#20700,#20701,
#20702,#20703,#20704,#20705,#20706,#20707,#20708,#20709,#20710,#20711,#20712,
#20713,#20714,#20715,#20716,#20717,#20718,#20719,#20720,#20721,#20722,#20723,
#20724,#20725,#20726,#20727,#20728,#20729,#20730,#20731,#20732,#20733,#20734,
#20735,#20736,#20737,#20738,#20739,#20740,#20741,#20742,#20743,#20744,#20745,
#20746,#20747,#20748,#20749,#20750,#20751,#20752,#20753,#20754,#20755,#20756,
#20757,#20758,#20759,#20760,#20761,#20762,#20763,#20764,#20765,#20766,#20767,
#20768,#20769,#20770,#20771,#20772,#20773,#20774,#20775,#20776,#20777,#20778,
#20779,#20780,#20781,#20782,#20783,#20784,#20785,#20786,#20787,#20788,#20789,
#20790,#20791,#20792,#20793,#20794,#20795,#20796,#20797,#20798,#20799,#20800,
#20801,#20802,#20803,#20804,#20805,#20806,#20807,#20808,#20809,#20810,#20811,
#20812,#20813,#20814,#20815,#20816,#20817,#20818,#20819,#20820,#20821,#20822,
#20823,#20824,#20825,#20826,#20827,#20828,#20829,#20830,#20831,#20832,#20833,
#20834));
#3872=EDGE_LOOP('',(#20835));
#3873=EDGE_LOOP('',(#20836,#20837,#20838,#20839,#20840,#20841));
#3874=EDGE_LOOP('',(#20842,#20843,#20844,#20845,#20846,#20847));
#3875=EDGE_LOOP('',(#20848,#20849,#20850,#20851,#20852,#20853));
#3876=EDGE_LOOP('',(#20854,#20855,#20856,#20857,#20858,#20859));
#3877=EDGE_LOOP('',(#20860,#20861,#20862,#20863,#20864,#20865));
#3878=EDGE_LOOP('',(#20866,#20867,#20868,#20869,#20870,#20871));
#3879=EDGE_LOOP('',(#20872,#20873,#20874,#20875,#20876,#20877));
#3880=EDGE_LOOP('',(#20878,#20879,#20880,#20881,#20882,#20883));
#3881=EDGE_LOOP('',(#20884,#20885,#20886,#20887,#20888,#20889));
#3882=EDGE_LOOP('',(#20890,#20891,#20892,#20893,#20894,#20895));
#3883=EDGE_LOOP('',(#20896,#20897,#20898,#20899,#20900,#20901));
#3884=EDGE_LOOP('',(#20902,#20903,#20904,#20905,#20906,#20907));
#3885=EDGE_LOOP('',(#20908,#20909,#20910,#20911,#20912,#20913));
#3886=EDGE_LOOP('',(#20914,#20915,#20916,#20917,#20918,#20919));
#3887=EDGE_LOOP('',(#20920,#20921,#20922,#20923,#20924,#20925));
#3888=EDGE_LOOP('',(#20926,#20927,#20928,#20929,#20930,#20931));
#3889=EDGE_LOOP('',(#20932,#20933,#20934,#20935,#20936,#20937));
#3890=EDGE_LOOP('',(#20938,#20939,#20940,#20941,#20942,#20943));
#3891=EDGE_LOOP('',(#20944,#20945,#20946,#20947,#20948,#20949));
#3892=EDGE_LOOP('',(#20950,#20951,#20952,#20953,#20954,#20955));
#3893=EDGE_LOOP('',(#20956,#20957,#20958,#20959,#20960,#20961));
#3894=EDGE_LOOP('',(#20962,#20963,#20964,#20965,#20966,#20967));
#3895=EDGE_LOOP('',(#20968,#20969,#20970,#20971,#20972,#20973));
#3896=EDGE_LOOP('',(#20974,#20975,#20976,#20977,#20978,#20979));
#3897=EDGE_LOOP('',(#20980,#20981,#20982,#20983));
#3898=EDGE_LOOP('',(#20984,#20985,#20986,#20987));
#3899=EDGE_LOOP('',(#20988,#20989,#20990,#20991));
#3900=EDGE_LOOP('',(#20992,#20993,#20994,#20995));
#3901=EDGE_LOOP('',(#20996,#20997,#20998,#20999));
#3902=EDGE_LOOP('',(#21000,#21001,#21002,#21003));
#3903=EDGE_LOOP('',(#21004,#21005,#21006,#21007));
#3904=EDGE_LOOP('',(#21008,#21009,#21010,#21011));
#3905=EDGE_LOOP('',(#21012,#21013,#21014,#21015));
#3906=EDGE_LOOP('',(#21016,#21017,#21018,#21019));
#3907=EDGE_LOOP('',(#21020,#21021,#21022,#21023));
#3908=EDGE_LOOP('',(#21024,#21025,#21026,#21027));
#3909=EDGE_LOOP('',(#21028,#21029,#21030,#21031));
#3910=EDGE_LOOP('',(#21032,#21033,#21034,#21035));
#3911=EDGE_LOOP('',(#21036,#21037,#21038,#21039));
#3912=EDGE_LOOP('',(#21040,#21041,#21042,#21043));
#3913=EDGE_LOOP('',(#21044,#21045,#21046,#21047,#21048,#21049));
#3914=EDGE_LOOP('',(#21050,#21051,#21052,#21053));
#3915=EDGE_LOOP('',(#21054,#21055,#21056,#21057,#21058,#21059));
#3916=EDGE_LOOP('',(#21060,#21061,#21062,#21063,#21064,#21065));
#3917=EDGE_LOOP('',(#21066,#21067,#21068,#21069));
#3918=EDGE_LOOP('',(#21070,#21071,#21072,#21073));
#3919=EDGE_LOOP('',(#21074,#21075,#21076,#21077));
#3920=EDGE_LOOP('',(#21078,#21079,#21080,#21081));
#3921=EDGE_LOOP('',(#21082,#21083,#21084,#21085));
#3922=EDGE_LOOP('',(#21086,#21087,#21088,#21089));
#3923=EDGE_LOOP('',(#21090,#21091,#21092,#21093));
#3924=EDGE_LOOP('',(#21094,#21095,#21096,#21097));
#3925=EDGE_LOOP('',(#21098,#21099,#21100,#21101));
#3926=EDGE_LOOP('',(#21102,#21103,#21104,#21105));
#3927=EDGE_LOOP('',(#21106,#21107,#21108,#21109));
#3928=EDGE_LOOP('',(#21110,#21111,#21112,#21113));
#3929=EDGE_LOOP('',(#21114,#21115,#21116,#21117));
#3930=EDGE_LOOP('',(#21118,#21119,#21120,#21121));
#3931=EDGE_LOOP('',(#21122,#21123,#21124,#21125));
#3932=EDGE_LOOP('',(#21126,#21127,#21128,#21129));
#3933=EDGE_LOOP('',(#21130,#21131,#21132,#21133,#21134,#21135));
#3934=EDGE_LOOP('',(#21136,#21137,#21138,#21139));
#3935=EDGE_LOOP('',(#21140,#21141,#21142,#21143,#21144,#21145));
#3936=EDGE_LOOP('',(#21146,#21147,#21148,#21149,#21150,#21151));
#3937=EDGE_LOOP('',(#21152,#21153,#21154,#21155));
#3938=EDGE_LOOP('',(#21156,#21157,#21158,#21159));
#3939=EDGE_LOOP('',(#21160,#21161,#21162,#21163));
#3940=EDGE_LOOP('',(#21164,#21165,#21166,#21167));
#3941=EDGE_LOOP('',(#21168,#21169,#21170,#21171));
#3942=EDGE_LOOP('',(#21172,#21173,#21174,#21175));
#3943=EDGE_LOOP('',(#21176,#21177,#21178,#21179));
#3944=EDGE_LOOP('',(#21180,#21181,#21182,#21183));
#3945=EDGE_LOOP('',(#21184,#21185,#21186,#21187));
#3946=EDGE_LOOP('',(#21188,#21189,#21190,#21191));
#3947=EDGE_LOOP('',(#21192,#21193,#21194,#21195));
#3948=EDGE_LOOP('',(#21196,#21197,#21198,#21199));
#3949=EDGE_LOOP('',(#21200,#21201,#21202,#21203));
#3950=EDGE_LOOP('',(#21204,#21205,#21206,#21207));
#3951=EDGE_LOOP('',(#21208,#21209,#21210,#21211));
#3952=EDGE_LOOP('',(#21212,#21213,#21214,#21215));
#3953=EDGE_LOOP('',(#21216,#21217,#21218,#21219,#21220,#21221));
#3954=EDGE_LOOP('',(#21222,#21223,#21224,#21225));
#3955=EDGE_LOOP('',(#21226,#21227,#21228,#21229,#21230,#21231));
#3956=EDGE_LOOP('',(#21232,#21233,#21234,#21235,#21236,#21237));
#3957=EDGE_LOOP('',(#21238,#21239,#21240,#21241));
#3958=EDGE_LOOP('',(#21242,#21243,#21244,#21245));
#3959=EDGE_LOOP('',(#21246,#21247,#21248,#21249));
#3960=EDGE_LOOP('',(#21250,#21251,#21252,#21253));
#3961=EDGE_LOOP('',(#21254,#21255,#21256,#21257));
#3962=EDGE_LOOP('',(#21258,#21259,#21260,#21261));
#3963=EDGE_LOOP('',(#21262,#21263,#21264,#21265));
#3964=EDGE_LOOP('',(#21266,#21267,#21268,#21269));
#3965=EDGE_LOOP('',(#21270,#21271,#21272,#21273));
#3966=EDGE_LOOP('',(#21274,#21275,#21276,#21277));
#3967=EDGE_LOOP('',(#21278,#21279,#21280,#21281));
#3968=EDGE_LOOP('',(#21282,#21283,#21284,#21285));
#3969=EDGE_LOOP('',(#21286,#21287,#21288,#21289));
#3970=EDGE_LOOP('',(#21290,#21291,#21292,#21293));
#3971=EDGE_LOOP('',(#21294,#21295,#21296,#21297));
#3972=EDGE_LOOP('',(#21298,#21299,#21300,#21301));
#3973=EDGE_LOOP('',(#21302,#21303,#21304,#21305,#21306,#21307));
#3974=EDGE_LOOP('',(#21308,#21309,#21310,#21311));
#3975=EDGE_LOOP('',(#21312,#21313,#21314,#21315,#21316,#21317));
#3976=EDGE_LOOP('',(#21318,#21319,#21320,#21321,#21322,#21323));
#3977=EDGE_LOOP('',(#21324,#21325,#21326,#21327));
#3978=EDGE_LOOP('',(#21328,#21329,#21330,#21331));
#3979=EDGE_LOOP('',(#21332,#21333,#21334,#21335));
#3980=EDGE_LOOP('',(#21336,#21337,#21338,#21339));
#3981=EDGE_LOOP('',(#21340,#21341,#21342,#21343));
#3982=EDGE_LOOP('',(#21344,#21345,#21346,#21347));
#3983=EDGE_LOOP('',(#21348,#21349,#21350,#21351));
#3984=EDGE_LOOP('',(#21352,#21353,#21354,#21355));
#3985=EDGE_LOOP('',(#21356,#21357,#21358,#21359));
#3986=EDGE_LOOP('',(#21360,#21361,#21362,#21363));
#3987=EDGE_LOOP('',(#21364,#21365,#21366,#21367));
#3988=EDGE_LOOP('',(#21368,#21369,#21370,#21371));
#3989=EDGE_LOOP('',(#21372,#21373,#21374,#21375));
#3990=EDGE_LOOP('',(#21376,#21377,#21378,#21379));
#3991=EDGE_LOOP('',(#21380,#21381,#21382,#21383));
#3992=EDGE_LOOP('',(#21384,#21385,#21386,#21387));
#3993=EDGE_LOOP('',(#21388,#21389,#21390,#21391,#21392,#21393));
#3994=EDGE_LOOP('',(#21394,#21395,#21396,#21397));
#3995=EDGE_LOOP('',(#21398,#21399,#21400,#21401,#21402,#21403));
#3996=EDGE_LOOP('',(#21404,#21405,#21406,#21407,#21408,#21409));
#3997=EDGE_LOOP('',(#21410,#21411,#21412,#21413));
#3998=EDGE_LOOP('',(#21414,#21415,#21416,#21417));
#3999=EDGE_LOOP('',(#21418,#21419,#21420,#21421));
#4000=EDGE_LOOP('',(#21422,#21423,#21424,#21425));
#4001=EDGE_LOOP('',(#21426,#21427,#21428,#21429));
#4002=EDGE_LOOP('',(#21430,#21431,#21432,#21433));
#4003=EDGE_LOOP('',(#21434,#21435,#21436,#21437));
#4004=EDGE_LOOP('',(#21438,#21439,#21440,#21441));
#4005=EDGE_LOOP('',(#21442,#21443,#21444,#21445));
#4006=EDGE_LOOP('',(#21446,#21447,#21448,#21449));
#4007=EDGE_LOOP('',(#21450,#21451,#21452,#21453));
#4008=EDGE_LOOP('',(#21454,#21455,#21456,#21457));
#4009=EDGE_LOOP('',(#21458,#21459,#21460,#21461));
#4010=EDGE_LOOP('',(#21462,#21463,#21464,#21465));
#4011=EDGE_LOOP('',(#21466,#21467,#21468,#21469));
#4012=EDGE_LOOP('',(#21470,#21471,#21472,#21473));
#4013=EDGE_LOOP('',(#21474,#21475,#21476,#21477,#21478,#21479));
#4014=EDGE_LOOP('',(#21480,#21481,#21482,#21483));
#4015=EDGE_LOOP('',(#21484,#21485,#21486,#21487,#21488,#21489));
#4016=EDGE_LOOP('',(#21490,#21491,#21492,#21493,#21494,#21495));
#4017=EDGE_LOOP('',(#21496,#21497,#21498,#21499));
#4018=EDGE_LOOP('',(#21500,#21501,#21502,#21503));
#4019=EDGE_LOOP('',(#21504,#21505,#21506,#21507));
#4020=EDGE_LOOP('',(#21508,#21509,#21510,#21511));
#4021=EDGE_LOOP('',(#21512,#21513,#21514,#21515));
#4022=EDGE_LOOP('',(#21516,#21517,#21518,#21519));
#4023=EDGE_LOOP('',(#21520,#21521,#21522,#21523));
#4024=EDGE_LOOP('',(#21524,#21525,#21526,#21527));
#4025=EDGE_LOOP('',(#21528,#21529,#21530,#21531));
#4026=EDGE_LOOP('',(#21532,#21533,#21534,#21535));
#4027=EDGE_LOOP('',(#21536,#21537,#21538,#21539));
#4028=EDGE_LOOP('',(#21540,#21541,#21542,#21543));
#4029=EDGE_LOOP('',(#21544,#21545,#21546,#21547));
#4030=EDGE_LOOP('',(#21548,#21549,#21550,#21551));
#4031=EDGE_LOOP('',(#21552,#21553,#21554,#21555));
#4032=EDGE_LOOP('',(#21556,#21557,#21558,#21559));
#4033=EDGE_LOOP('',(#21560,#21561,#21562,#21563,#21564,#21565));
#4034=EDGE_LOOP('',(#21566,#21567,#21568,#21569));
#4035=EDGE_LOOP('',(#21570,#21571,#21572,#21573,#21574,#21575));
#4036=EDGE_LOOP('',(#21576,#21577,#21578,#21579,#21580,#21581));
#4037=EDGE_LOOP('',(#21582,#21583,#21584,#21585));
#4038=EDGE_LOOP('',(#21586,#21587,#21588,#21589));
#4039=EDGE_LOOP('',(#21590,#21591,#21592,#21593));
#4040=EDGE_LOOP('',(#21594,#21595,#21596,#21597));
#4041=EDGE_LOOP('',(#21598,#21599,#21600,#21601));
#4042=EDGE_LOOP('',(#21602,#21603,#21604,#21605));
#4043=EDGE_LOOP('',(#21606,#21607,#21608,#21609));
#4044=EDGE_LOOP('',(#21610,#21611,#21612,#21613));
#4045=EDGE_LOOP('',(#21614,#21615,#21616,#21617));
#4046=EDGE_LOOP('',(#21618,#21619,#21620,#21621));
#4047=EDGE_LOOP('',(#21622,#21623,#21624,#21625));
#4048=EDGE_LOOP('',(#21626,#21627,#21628,#21629));
#4049=EDGE_LOOP('',(#21630,#21631,#21632,#21633));
#4050=EDGE_LOOP('',(#21634,#21635,#21636,#21637));
#4051=EDGE_LOOP('',(#21638,#21639,#21640,#21641));
#4052=EDGE_LOOP('',(#21642,#21643,#21644,#21645));
#4053=EDGE_LOOP('',(#21646,#21647,#21648,#21649,#21650,#21651));
#4054=EDGE_LOOP('',(#21652,#21653,#21654,#21655));
#4055=EDGE_LOOP('',(#21656,#21657,#21658,#21659,#21660,#21661));
#4056=EDGE_LOOP('',(#21662,#21663,#21664,#21665,#21666,#21667));
#4057=EDGE_LOOP('',(#21668,#21669,#21670,#21671));
#4058=EDGE_LOOP('',(#21672,#21673,#21674,#21675));
#4059=EDGE_LOOP('',(#21676,#21677,#21678,#21679));
#4060=EDGE_LOOP('',(#21680,#21681,#21682,#21683));
#4061=EDGE_LOOP('',(#21684,#21685,#21686,#21687));
#4062=EDGE_LOOP('',(#21688,#21689,#21690,#21691));
#4063=EDGE_LOOP('',(#21692,#21693,#21694,#21695));
#4064=EDGE_LOOP('',(#21696,#21697,#21698,#21699));
#4065=EDGE_LOOP('',(#21700,#21701,#21702,#21703));
#4066=EDGE_LOOP('',(#21704,#21705,#21706,#21707));
#4067=EDGE_LOOP('',(#21708,#21709,#21710,#21711));
#4068=EDGE_LOOP('',(#21712,#21713,#21714,#21715));
#4069=EDGE_LOOP('',(#21716,#21717,#21718,#21719));
#4070=EDGE_LOOP('',(#21720,#21721,#21722,#21723));
#4071=EDGE_LOOP('',(#21724,#21725,#21726,#21727));
#4072=EDGE_LOOP('',(#21728,#21729,#21730,#21731));
#4073=EDGE_LOOP('',(#21732,#21733,#21734,#21735,#21736,#21737));
#4074=EDGE_LOOP('',(#21738,#21739,#21740,#21741));
#4075=EDGE_LOOP('',(#21742,#21743,#21744,#21745,#21746,#21747));
#4076=EDGE_LOOP('',(#21748,#21749,#21750,#21751,#21752,#21753));
#4077=EDGE_LOOP('',(#21754,#21755,#21756,#21757));
#4078=EDGE_LOOP('',(#21758,#21759,#21760,#21761));
#4079=EDGE_LOOP('',(#21762,#21763,#21764,#21765));
#4080=EDGE_LOOP('',(#21766,#21767,#21768,#21769));
#4081=EDGE_LOOP('',(#21770,#21771,#21772,#21773));
#4082=EDGE_LOOP('',(#21774,#21775,#21776,#21777));
#4083=EDGE_LOOP('',(#21778,#21779,#21780,#21781));
#4084=EDGE_LOOP('',(#21782,#21783,#21784,#21785));
#4085=EDGE_LOOP('',(#21786,#21787,#21788,#21789));
#4086=EDGE_LOOP('',(#21790,#21791,#21792,#21793));
#4087=EDGE_LOOP('',(#21794,#21795,#21796,#21797));
#4088=EDGE_LOOP('',(#21798,#21799,#21800,#21801));
#4089=EDGE_LOOP('',(#21802,#21803,#21804,#21805));
#4090=EDGE_LOOP('',(#21806,#21807,#21808,#21809));
#4091=EDGE_LOOP('',(#21810,#21811,#21812,#21813));
#4092=EDGE_LOOP('',(#21814,#21815,#21816,#21817));
#4093=EDGE_LOOP('',(#21818,#21819,#21820,#21821,#21822,#21823));
#4094=EDGE_LOOP('',(#21824,#21825,#21826,#21827));
#4095=EDGE_LOOP('',(#21828,#21829,#21830,#21831,#21832,#21833));
#4096=EDGE_LOOP('',(#21834,#21835,#21836,#21837,#21838,#21839));
#4097=EDGE_LOOP('',(#21840,#21841,#21842,#21843));
#4098=EDGE_LOOP('',(#21844,#21845,#21846,#21847));
#4099=EDGE_LOOP('',(#21848,#21849,#21850,#21851));
#4100=EDGE_LOOP('',(#21852,#21853,#21854,#21855));
#4101=EDGE_LOOP('',(#21856,#21857,#21858,#21859));
#4102=EDGE_LOOP('',(#21860,#21861,#21862,#21863));
#4103=EDGE_LOOP('',(#21864,#21865,#21866,#21867));
#4104=EDGE_LOOP('',(#21868,#21869,#21870,#21871));
#4105=EDGE_LOOP('',(#21872,#21873,#21874,#21875));
#4106=EDGE_LOOP('',(#21876,#21877,#21878,#21879));
#4107=EDGE_LOOP('',(#21880,#21881,#21882,#21883));
#4108=EDGE_LOOP('',(#21884,#21885,#21886,#21887));
#4109=EDGE_LOOP('',(#21888,#21889,#21890,#21891));
#4110=EDGE_LOOP('',(#21892,#21893,#21894,#21895));
#4111=EDGE_LOOP('',(#21896,#21897,#21898,#21899));
#4112=EDGE_LOOP('',(#21900,#21901,#21902,#21903));
#4113=EDGE_LOOP('',(#21904,#21905,#21906,#21907,#21908,#21909));
#4114=EDGE_LOOP('',(#21910,#21911,#21912,#21913));
#4115=EDGE_LOOP('',(#21914,#21915,#21916,#21917,#21918,#21919));
#4116=EDGE_LOOP('',(#21920,#21921,#21922,#21923,#21924,#21925));
#4117=EDGE_LOOP('',(#21926,#21927,#21928,#21929));
#4118=EDGE_LOOP('',(#21930,#21931,#21932,#21933));
#4119=EDGE_LOOP('',(#21934,#21935,#21936,#21937));
#4120=EDGE_LOOP('',(#21938,#21939,#21940,#21941));
#4121=EDGE_LOOP('',(#21942,#21943,#21944,#21945));
#4122=EDGE_LOOP('',(#21946,#21947,#21948,#21949));
#4123=EDGE_LOOP('',(#21950,#21951,#21952,#21953));
#4124=EDGE_LOOP('',(#21954,#21955,#21956,#21957));
#4125=EDGE_LOOP('',(#21958,#21959,#21960,#21961));
#4126=EDGE_LOOP('',(#21962,#21963,#21964,#21965));
#4127=EDGE_LOOP('',(#21966,#21967,#21968,#21969));
#4128=EDGE_LOOP('',(#21970,#21971,#21972,#21973));
#4129=EDGE_LOOP('',(#21974,#21975,#21976,#21977));
#4130=EDGE_LOOP('',(#21978,#21979,#21980,#21981));
#4131=EDGE_LOOP('',(#21982,#21983,#21984,#21985));
#4132=EDGE_LOOP('',(#21986,#21987,#21988,#21989));
#4133=EDGE_LOOP('',(#21990,#21991,#21992,#21993,#21994,#21995));
#4134=EDGE_LOOP('',(#21996,#21997,#21998,#21999));
#4135=EDGE_LOOP('',(#22000,#22001,#22002,#22003,#22004,#22005));
#4136=EDGE_LOOP('',(#22006,#22007,#22008,#22009));
#4137=EDGE_LOOP('',(#22010));
#4138=EDGE_LOOP('',(#22011,#22012,#22013,#22014));
#4139=EDGE_LOOP('',(#22015));
#5889=LINE('',#38100,#8758);
#5890=LINE('',#38102,#8759);
#5891=LINE('',#38104,#8760);
#5892=LINE('',#38106,#8761);
#5893=LINE('',#38108,#8762);
#5894=LINE('',#38109,#8763);
#5895=LINE('',#38112,#8764);
#5896=LINE('',#38114,#8765);
#5897=LINE('',#38116,#8766);
#5898=LINE('',#38118,#8767);
#5899=LINE('',#38120,#8768);
#5900=LINE('',#38122,#8769);
#5901=LINE('',#38124,#8770);
#5902=LINE('',#38126,#8771);
#5903=LINE('',#38128,#8772);
#5904=LINE('',#38130,#8773);
#5905=LINE('',#38132,#8774);
#5906=LINE('',#38134,#8775);
#5907=LINE('',#38136,#8776);
#5908=LINE('',#38138,#8777);
#5909=LINE('',#38140,#8778);
#5910=LINE('',#38142,#8779);
#5911=LINE('',#38144,#8780);
#5912=LINE('',#38146,#8781);
#5913=LINE('',#38148,#8782);
#5914=LINE('',#38150,#8783);
#5915=LINE('',#38152,#8784);
#5916=LINE('',#38154,#8785);
#5917=LINE('',#38156,#8786);
#5918=LINE('',#38158,#8787);
#5919=LINE('',#38160,#8788);
#5920=LINE('',#38162,#8789);
#5921=LINE('',#38164,#8790);
#5922=LINE('',#38166,#8791);
#5923=LINE('',#38168,#8792);
#5924=LINE('',#38170,#8793);
#5925=LINE('',#38172,#8794);
#5926=LINE('',#38174,#8795);
#5927=LINE('',#38176,#8796);
#5928=LINE('',#38178,#8797);
#5929=LINE('',#38180,#8798);
#5930=LINE('',#38182,#8799);
#5931=LINE('',#38184,#8800);
#5932=LINE('',#38186,#8801);
#5933=LINE('',#38188,#8802);
#5934=LINE('',#38190,#8803);
#5935=LINE('',#38192,#8804);
#5936=LINE('',#38194,#8805);
#5937=LINE('',#38196,#8806);
#5938=LINE('',#38198,#8807);
#5939=LINE('',#38200,#8808);
#5940=LINE('',#38202,#8809);
#5941=LINE('',#38204,#8810);
#5942=LINE('',#38206,#8811);
#5943=LINE('',#38208,#8812);
#5944=LINE('',#38210,#8813);
#5945=LINE('',#38212,#8814);
#5946=LINE('',#38214,#8815);
#5947=LINE('',#38216,#8816);
#5948=LINE('',#38218,#8817);
#5949=LINE('',#38220,#8818);
#5950=LINE('',#38222,#8819);
#5951=LINE('',#38224,#8820);
#5952=LINE('',#38226,#8821);
#5953=LINE('',#38228,#8822);
#5954=LINE('',#38230,#8823);
#5955=LINE('',#38232,#8824);
#5956=LINE('',#38234,#8825);
#5957=LINE('',#38236,#8826);
#5958=LINE('',#38238,#8827);
#5959=LINE('',#38240,#8828);
#5960=LINE('',#38242,#8829);
#5961=LINE('',#38244,#8830);
#5962=LINE('',#38246,#8831);
#5963=LINE('',#38248,#8832);
#5964=LINE('',#38250,#8833);
#5965=LINE('',#38252,#8834);
#5966=LINE('',#38254,#8835);
#5967=LINE('',#38256,#8836);
#5968=LINE('',#38258,#8837);
#5969=LINE('',#38260,#8838);
#5970=LINE('',#38262,#8839);
#5971=LINE('',#38264,#8840);
#5972=LINE('',#38266,#8841);
#5973=LINE('',#38268,#8842);
#5974=LINE('',#38270,#8843);
#5975=LINE('',#38272,#8844);
#5976=LINE('',#38274,#8845);
#5977=LINE('',#38276,#8846);
#5978=LINE('',#38278,#8847);
#5979=LINE('',#38280,#8848);
#5980=LINE('',#38282,#8849);
#5981=LINE('',#38284,#8850);
#5982=LINE('',#38286,#8851);
#5983=LINE('',#38288,#8852);
#5984=LINE('',#38290,#8853);
#5985=LINE('',#38292,#8854);
#5986=LINE('',#38294,#8855);
#5987=LINE('',#38296,#8856);
#5988=LINE('',#38298,#8857);
#5989=LINE('',#38300,#8858);
#5990=LINE('',#38302,#8859);
#5991=LINE('',#38304,#8860);
#5992=LINE('',#38306,#8861);
#5993=LINE('',#38308,#8862);
#5994=LINE('',#38310,#8863);
#5995=LINE('',#38312,#8864);
#5996=LINE('',#38314,#8865);
#5997=LINE('',#38316,#8866);
#5998=LINE('',#38318,#8867);
#5999=LINE('',#38320,#8868);
#6000=LINE('',#38322,#8869);
#6001=LINE('',#38324,#8870);
#6002=LINE('',#38326,#8871);
#6003=LINE('',#38328,#8872);
#6004=LINE('',#38330,#8873);
#6005=LINE('',#38332,#8874);
#6006=LINE('',#38334,#8875);
#6007=LINE('',#38336,#8876);
#6008=LINE('',#38338,#8877);
#6009=LINE('',#38340,#8878);
#6010=LINE('',#38342,#8879);
#6011=LINE('',#38344,#8880);
#6012=LINE('',#38346,#8881);
#6013=LINE('',#38348,#8882);
#6014=LINE('',#38350,#8883);
#6015=LINE('',#38352,#8884);
#6016=LINE('',#38354,#8885);
#6017=LINE('',#38356,#8886);
#6018=LINE('',#38358,#8887);
#6019=LINE('',#38360,#8888);
#6020=LINE('',#38362,#8889);
#6021=LINE('',#38364,#8890);
#6022=LINE('',#38366,#8891);
#6023=LINE('',#38368,#8892);
#6024=LINE('',#38370,#8893);
#6025=LINE('',#38372,#8894);
#6026=LINE('',#38374,#8895);
#6027=LINE('',#38376,#8896);
#6028=LINE('',#38378,#8897);
#6029=LINE('',#38380,#8898);
#6030=LINE('',#38382,#8899);
#6031=LINE('',#38384,#8900);
#6032=LINE('',#38386,#8901);
#6033=LINE('',#38388,#8902);
#6034=LINE('',#38390,#8903);
#6035=LINE('',#38392,#8904);
#6036=LINE('',#38394,#8905);
#6037=LINE('',#38396,#8906);
#6038=LINE('',#38398,#8907);
#6039=LINE('',#38400,#8908);
#6040=LINE('',#38402,#8909);
#6041=LINE('',#38404,#8910);
#6042=LINE('',#38406,#8911);
#6043=LINE('',#38408,#8912);
#6044=LINE('',#38410,#8913);
#6045=LINE('',#38412,#8914);
#6046=LINE('',#38414,#8915);
#6047=LINE('',#38416,#8916);
#6048=LINE('',#38418,#8917);
#6049=LINE('',#38420,#8918);
#6050=LINE('',#38422,#8919);
#6051=LINE('',#38424,#8920);
#6052=LINE('',#38426,#8921);
#6053=LINE('',#38428,#8922);
#6054=LINE('',#38430,#8923);
#6055=LINE('',#38432,#8924);
#6056=LINE('',#38434,#8925);
#6057=LINE('',#38436,#8926);
#6058=LINE('',#38438,#8927);
#6059=LINE('',#38440,#8928);
#6060=LINE('',#38442,#8929);
#6061=LINE('',#38444,#8930);
#6062=LINE('',#38446,#8931);
#6063=LINE('',#38448,#8932);
#6064=LINE('',#38450,#8933);
#6065=LINE('',#38452,#8934);
#6066=LINE('',#38454,#8935);
#6067=LINE('',#38456,#8936);
#6068=LINE('',#38458,#8937);
#6069=LINE('',#38460,#8938);
#6070=LINE('',#38462,#8939);
#6071=LINE('',#38464,#8940);
#6072=LINE('',#38466,#8941);
#6073=LINE('',#38468,#8942);
#6074=LINE('',#38470,#8943);
#6075=LINE('',#38472,#8944);
#6076=LINE('',#38474,#8945);
#6077=LINE('',#38476,#8946);
#6078=LINE('',#38478,#8947);
#6079=LINE('',#38480,#8948);
#6080=LINE('',#38482,#8949);
#6081=LINE('',#38484,#8950);
#6082=LINE('',#38486,#8951);
#6083=LINE('',#38488,#8952);
#6084=LINE('',#38490,#8953);
#6085=LINE('',#38492,#8954);
#6086=LINE('',#38494,#8955);
#6087=LINE('',#38496,#8956);
#6088=LINE('',#38498,#8957);
#6089=LINE('',#38500,#8958);
#6090=LINE('',#38502,#8959);
#6091=LINE('',#38504,#8960);
#6092=LINE('',#38506,#8961);
#6093=LINE('',#38508,#8962);
#6094=LINE('',#38510,#8963);
#6095=LINE('',#38512,#8964);
#6096=LINE('',#38514,#8965);
#6097=LINE('',#38516,#8966);
#6098=LINE('',#38518,#8967);
#6099=LINE('',#38520,#8968);
#6100=LINE('',#38522,#8969);
#6101=LINE('',#38524,#8970);
#6102=LINE('',#38526,#8971);
#6103=LINE('',#38528,#8972);
#6104=LINE('',#38530,#8973);
#6105=LINE('',#38532,#8974);
#6106=LINE('',#38534,#8975);
#6107=LINE('',#38536,#8976);
#6108=LINE('',#38538,#8977);
#6109=LINE('',#38540,#8978);
#6110=LINE('',#38542,#8979);
#6111=LINE('',#38544,#8980);
#6112=LINE('',#38546,#8981);
#6113=LINE('',#38548,#8982);
#6114=LINE('',#38550,#8983);
#6115=LINE('',#38552,#8984);
#6116=LINE('',#38554,#8985);
#6117=LINE('',#38556,#8986);
#6118=LINE('',#38558,#8987);
#6119=LINE('',#38560,#8988);
#6120=LINE('',#38562,#8989);
#6121=LINE('',#38564,#8990);
#6122=LINE('',#38566,#8991);
#6123=LINE('',#38568,#8992);
#6124=LINE('',#38570,#8993);
#6125=LINE('',#38572,#8994);
#6126=LINE('',#38574,#8995);
#6127=LINE('',#38576,#8996);
#6128=LINE('',#38578,#8997);
#6129=LINE('',#38580,#8998);
#6130=LINE('',#38582,#8999);
#6131=LINE('',#38584,#9000);
#6132=LINE('',#38586,#9001);
#6133=LINE('',#38587,#9002);
#6134=LINE('',#38592,#9003);
#6135=LINE('',#38594,#9004);
#6136=LINE('',#38596,#9005);
#6137=LINE('',#38597,#9006);
#6138=LINE('',#38600,#9007);
#6139=LINE('',#38601,#9008);
#6140=LINE('',#38604,#9009);
#6141=LINE('',#38606,#9010);
#6142=LINE('',#38608,#9011);
#6143=LINE('',#38610,#9012);
#6144=LINE('',#38611,#9013);
#6145=LINE('',#38614,#9014);
#6146=LINE('',#38616,#9015);
#6147=LINE('',#38618,#9016);
#6148=LINE('',#38619,#9017);
#6149=LINE('',#38622,#9018);
#6150=LINE('',#38623,#9019);
#6151=LINE('',#38626,#9020);
#6152=LINE('',#38628,#9021);
#6153=LINE('',#38630,#9022);
#6154=LINE('',#38632,#9023);
#6155=LINE('',#38633,#9024);
#6156=LINE('',#38636,#9025);
#6157=LINE('',#38638,#9026);
#6158=LINE('',#38640,#9027);
#6159=LINE('',#38641,#9028);
#6160=LINE('',#38644,#9029);
#6161=LINE('',#38645,#9030);
#6162=LINE('',#38648,#9031);
#6163=LINE('',#38650,#9032);
#6164=LINE('',#38652,#9033);
#6165=LINE('',#38654,#9034);
#6166=LINE('',#38655,#9035);
#6167=LINE('',#38658,#9036);
#6168=LINE('',#38660,#9037);
#6169=LINE('',#38662,#9038);
#6170=LINE('',#38663,#9039);
#6171=LINE('',#38666,#9040);
#6172=LINE('',#38667,#9041);
#6173=LINE('',#38670,#9042);
#6174=LINE('',#38672,#9043);
#6175=LINE('',#38674,#9044);
#6176=LINE('',#38676,#9045);
#6177=LINE('',#38677,#9046);
#6178=LINE('',#38680,#9047);
#6179=LINE('',#38682,#9048);
#6180=LINE('',#38684,#9049);
#6181=LINE('',#38685,#9050);
#6182=LINE('',#38688,#9051);
#6183=LINE('',#38689,#9052);
#6184=LINE('',#38692,#9053);
#6185=LINE('',#38694,#9054);
#6186=LINE('',#38696,#9055);
#6187=LINE('',#38698,#9056);
#6188=LINE('',#38699,#9057);
#6189=LINE('',#38702,#9058);
#6190=LINE('',#38704,#9059);
#6191=LINE('',#38706,#9060);
#6192=LINE('',#38707,#9061);
#6193=LINE('',#38710,#9062);
#6194=LINE('',#38711,#9063);
#6195=LINE('',#38714,#9064);
#6196=LINE('',#38716,#9065);
#6197=LINE('',#38718,#9066);
#6198=LINE('',#38720,#9067);
#6199=LINE('',#38721,#9068);
#6200=LINE('',#38724,#9069);
#6201=LINE('',#38726,#9070);
#6202=LINE('',#38728,#9071);
#6203=LINE('',#38729,#9072);
#6204=LINE('',#38732,#9073);
#6205=LINE('',#38733,#9074);
#6206=LINE('',#38736,#9075);
#6207=LINE('',#38738,#9076);
#6208=LINE('',#38740,#9077);
#6209=LINE('',#38742,#9078);
#6210=LINE('',#38743,#9079);
#6211=LINE('',#38746,#9080);
#6212=LINE('',#38748,#9081);
#6213=LINE('',#38750,#9082);
#6214=LINE('',#38751,#9083);
#6215=LINE('',#38754,#9084);
#6216=LINE('',#38755,#9085);
#6217=LINE('',#38758,#9086);
#6218=LINE('',#38760,#9087);
#6219=LINE('',#38762,#9088);
#6220=LINE('',#38764,#9089);
#6221=LINE('',#38765,#9090);
#6222=LINE('',#38768,#9091);
#6223=LINE('',#38770,#9092);
#6224=LINE('',#38772,#9093);
#6225=LINE('',#38773,#9094);
#6226=LINE('',#38776,#9095);
#6227=LINE('',#38777,#9096);
#6228=LINE('',#38780,#9097);
#6229=LINE('',#38782,#9098);
#6230=LINE('',#38784,#9099);
#6231=LINE('',#38786,#9100);
#6232=LINE('',#38787,#9101);
#6233=LINE('',#38790,#9102);
#6234=LINE('',#38792,#9103);
#6235=LINE('',#38794,#9104);
#6236=LINE('',#38795,#9105);
#6237=LINE('',#38798,#9106);
#6238=LINE('',#38799,#9107);
#6239=LINE('',#38802,#9108);
#6240=LINE('',#38804,#9109);
#6241=LINE('',#38806,#9110);
#6242=LINE('',#38808,#9111);
#6243=LINE('',#38809,#9112);
#6244=LINE('',#38812,#9113);
#6245=LINE('',#38814,#9114);
#6246=LINE('',#38816,#9115);
#6247=LINE('',#38817,#9116);
#6248=LINE('',#38820,#9117);
#6249=LINE('',#38821,#9118);
#6250=LINE('',#38824,#9119);
#6251=LINE('',#38826,#9120);
#6252=LINE('',#38828,#9121);
#6253=LINE('',#38830,#9122);
#6254=LINE('',#38831,#9123);
#6255=LINE('',#38834,#9124);
#6256=LINE('',#38836,#9125);
#6257=LINE('',#38838,#9126);
#6258=LINE('',#38839,#9127);
#6259=LINE('',#38842,#9128);
#6260=LINE('',#38843,#9129);
#6261=LINE('',#38847,#9130);
#6262=LINE('',#38849,#9131);
#6263=LINE('',#38850,#9132);
#6264=LINE('',#38852,#9133);
#6265=LINE('',#38853,#9134);
#6266=LINE('',#38856,#9135);
#6267=LINE('',#38858,#9136);
#6268=LINE('',#38859,#9137);
#6269=LINE('',#38862,#9138);
#6270=LINE('',#38863,#9139);
#6271=LINE('',#38867,#9140);
#6272=LINE('',#38869,#9141);
#6273=LINE('',#38870,#9142);
#6274=LINE('',#38872,#9143);
#6275=LINE('',#38873,#9144);
#6276=LINE('',#38876,#9145);
#6277=LINE('',#38878,#9146);
#6278=LINE('',#38879,#9147);
#6279=LINE('',#38882,#9148);
#6280=LINE('',#38883,#9149);
#6281=LINE('',#38887,#9150);
#6282=LINE('',#38889,#9151);
#6283=LINE('',#38890,#9152);
#6284=LINE('',#38892,#9153);
#6285=LINE('',#38893,#9154);
#6286=LINE('',#38896,#9155);
#6287=LINE('',#38898,#9156);
#6288=LINE('',#38899,#9157);
#6289=LINE('',#38902,#9158);
#6290=LINE('',#38903,#9159);
#6291=LINE('',#38907,#9160);
#6292=LINE('',#38909,#9161);
#6293=LINE('',#38910,#9162);
#6294=LINE('',#38912,#9163);
#6295=LINE('',#38913,#9164);
#6296=LINE('',#38916,#9165);
#6297=LINE('',#38918,#9166);
#6298=LINE('',#38919,#9167);
#6299=LINE('',#38922,#9168);
#6300=LINE('',#38923,#9169);
#6301=LINE('',#38927,#9170);
#6302=LINE('',#38929,#9171);
#6303=LINE('',#38930,#9172);
#6304=LINE('',#38932,#9173);
#6305=LINE('',#38933,#9174);
#6306=LINE('',#38936,#9175);
#6307=LINE('',#38938,#9176);
#6308=LINE('',#38939,#9177);
#6309=LINE('',#38942,#9178);
#6310=LINE('',#38943,#9179);
#6311=LINE('',#38947,#9180);
#6312=LINE('',#38949,#9181);
#6313=LINE('',#38950,#9182);
#6314=LINE('',#38952,#9183);
#6315=LINE('',#38953,#9184);
#6316=LINE('',#38956,#9185);
#6317=LINE('',#38958,#9186);
#6318=LINE('',#38959,#9187);
#6319=LINE('',#38962,#9188);
#6320=LINE('',#38963,#9189);
#6321=LINE('',#38967,#9190);
#6322=LINE('',#38969,#9191);
#6323=LINE('',#38970,#9192);
#6324=LINE('',#38972,#9193);
#6325=LINE('',#38973,#9194);
#6326=LINE('',#38976,#9195);
#6327=LINE('',#38978,#9196);
#6328=LINE('',#38979,#9197);
#6329=LINE('',#38982,#9198);
#6330=LINE('',#38983,#9199);
#6331=LINE('',#38987,#9200);
#6332=LINE('',#38989,#9201);
#6333=LINE('',#38990,#9202);
#6334=LINE('',#38992,#9203);
#6335=LINE('',#38993,#9204);
#6336=LINE('',#38996,#9205);
#6337=LINE('',#38998,#9206);
#6338=LINE('',#38999,#9207);
#6339=LINE('',#39002,#9208);
#6340=LINE('',#39003,#9209);
#6341=LINE('',#39007,#9210);
#6342=LINE('',#39009,#9211);
#6343=LINE('',#39010,#9212);
#6344=LINE('',#39012,#9213);
#6345=LINE('',#39013,#9214);
#6346=LINE('',#39016,#9215);
#6347=LINE('',#39018,#9216);
#6348=LINE('',#39019,#9217);
#6349=LINE('',#39022,#9218);
#6350=LINE('',#39023,#9219);
#6351=LINE('',#39027,#9220);
#6352=LINE('',#39029,#9221);
#6353=LINE('',#39030,#9222);
#6354=LINE('',#39032,#9223);
#6355=LINE('',#39033,#9224);
#6356=LINE('',#39036,#9225);
#6357=LINE('',#39038,#9226);
#6358=LINE('',#39039,#9227);
#6359=LINE('',#39042,#9228);
#6360=LINE('',#39043,#9229);
#6361=LINE('',#39047,#9230);
#6362=LINE('',#39049,#9231);
#6363=LINE('',#39050,#9232);
#6364=LINE('',#39052,#9233);
#6365=LINE('',#39053,#9234);
#6366=LINE('',#39056,#9235);
#6367=LINE('',#39058,#9236);
#6368=LINE('',#39059,#9237);
#6369=LINE('',#39062,#9238);
#6370=LINE('',#39063,#9239);
#6371=LINE('',#39067,#9240);
#6372=LINE('',#39069,#9241);
#6373=LINE('',#39070,#9242);
#6374=LINE('',#39072,#9243);
#6375=LINE('',#39073,#9244);
#6376=LINE('',#39076,#9245);
#6377=LINE('',#39078,#9246);
#6378=LINE('',#39079,#9247);
#6379=LINE('',#39082,#9248);
#6380=LINE('',#39083,#9249);
#6381=LINE('',#39086,#9250);
#6382=LINE('',#39088,#9251);
#6383=LINE('',#39090,#9252);
#6384=LINE('',#39091,#9253);
#6385=LINE('',#39094,#9254);
#6386=LINE('',#39096,#9255);
#6387=LINE('',#39098,#9256);
#6388=LINE('',#39100,#9257);
#6389=LINE('',#39102,#9258);
#6390=LINE('',#39104,#9259);
#6391=LINE('',#39106,#9260);
#6392=LINE('',#39108,#9261);
#6393=LINE('',#39110,#9262);
#6394=LINE('',#39112,#9263);
#6395=LINE('',#39114,#9264);
#6396=LINE('',#39116,#9265);
#6397=LINE('',#39118,#9266);
#6398=LINE('',#39120,#9267);
#6399=LINE('',#39122,#9268);
#6400=LINE('',#39124,#9269);
#6401=LINE('',#39126,#9270);
#6402=LINE('',#39127,#9271);
#6403=LINE('',#39129,#9272);
#6404=LINE('',#39131,#9273);
#6405=LINE('',#39133,#9274);
#6406=LINE('',#39135,#9275);
#6407=LINE('',#39137,#9276);
#6408=LINE('',#39139,#9277);
#6409=LINE('',#39141,#9278);
#6410=LINE('',#39143,#9279);
#6411=LINE('',#39145,#9280);
#6412=LINE('',#39147,#9281);
#6413=LINE('',#39149,#9282);
#6414=LINE('',#39151,#9283);
#6415=LINE('',#39153,#9284);
#6416=LINE('',#39155,#9285);
#6417=LINE('',#39157,#9286);
#6418=LINE('',#39159,#9287);
#6419=LINE('',#39161,#9288);
#6420=LINE('',#39163,#9289);
#6421=LINE('',#39164,#9290);
#6422=LINE('',#39166,#9291);
#6423=LINE('',#39168,#9292);
#6424=LINE('',#39170,#9293);
#6425=LINE('',#39172,#9294);
#6426=LINE('',#39174,#9295);
#6427=LINE('',#39176,#9296);
#6428=LINE('',#39178,#9297);
#6429=LINE('',#39180,#9298);
#6430=LINE('',#39182,#9299);
#6431=LINE('',#39184,#9300);
#6432=LINE('',#39186,#9301);
#6433=LINE('',#39188,#9302);
#6434=LINE('',#39190,#9303);
#6435=LINE('',#39192,#9304);
#6436=LINE('',#39194,#9305);
#6437=LINE('',#39196,#9306);
#6438=LINE('',#39198,#9307);
#6439=LINE('',#39200,#9308);
#6440=LINE('',#39201,#9309);
#6441=LINE('',#39203,#9310);
#6442=LINE('',#39205,#9311);
#6443=LINE('',#39207,#9312);
#6444=LINE('',#39209,#9313);
#6445=LINE('',#39211,#9314);
#6446=LINE('',#39213,#9315);
#6447=LINE('',#39215,#9316);
#6448=LINE('',#39217,#9317);
#6449=LINE('',#39219,#9318);
#6450=LINE('',#39221,#9319);
#6451=LINE('',#39223,#9320);
#6452=LINE('',#39225,#9321);
#6453=LINE('',#39227,#9322);
#6454=LINE('',#39229,#9323);
#6455=LINE('',#39231,#9324);
#6456=LINE('',#39233,#9325);
#6457=LINE('',#39235,#9326);
#6458=LINE('',#39237,#9327);
#6459=LINE('',#39238,#9328);
#6460=LINE('',#39240,#9329);
#6461=LINE('',#39242,#9330);
#6462=LINE('',#39244,#9331);
#6463=LINE('',#39246,#9332);
#6464=LINE('',#39248,#9333);
#6465=LINE('',#39250,#9334);
#6466=LINE('',#39252,#9335);
#6467=LINE('',#39254,#9336);
#6468=LINE('',#39256,#9337);
#6469=LINE('',#39258,#9338);
#6470=LINE('',#39260,#9339);
#6471=LINE('',#39262,#9340);
#6472=LINE('',#39264,#9341);
#6473=LINE('',#39266,#9342);
#6474=LINE('',#39268,#9343);
#6475=LINE('',#39270,#9344);
#6476=LINE('',#39272,#9345);
#6477=LINE('',#39274,#9346);
#6478=LINE('',#39275,#9347);
#6479=LINE('',#39277,#9348);
#6480=LINE('',#39279,#9349);
#6481=LINE('',#39281,#9350);
#6482=LINE('',#39283,#9351);
#6483=LINE('',#39285,#9352);
#6484=LINE('',#39287,#9353);
#6485=LINE('',#39289,#9354);
#6486=LINE('',#39291,#9355);
#6487=LINE('',#39293,#9356);
#6488=LINE('',#39295,#9357);
#6489=LINE('',#39297,#9358);
#6490=LINE('',#39299,#9359);
#6491=LINE('',#39301,#9360);
#6492=LINE('',#39303,#9361);
#6493=LINE('',#39305,#9362);
#6494=LINE('',#39307,#9363);
#6495=LINE('',#39309,#9364);
#6496=LINE('',#39311,#9365);
#6497=LINE('',#39312,#9366);
#6498=LINE('',#39314,#9367);
#6499=LINE('',#39316,#9368);
#6500=LINE('',#39318,#9369);
#6501=LINE('',#39320,#9370);
#6502=LINE('',#39322,#9371);
#6503=LINE('',#39324,#9372);
#6504=LINE('',#39326,#9373);
#6505=LINE('',#39328,#9374);
#6506=LINE('',#39330,#9375);
#6507=LINE('',#39332,#9376);
#6508=LINE('',#39334,#9377);
#6509=LINE('',#39336,#9378);
#6510=LINE('',#39338,#9379);
#6511=LINE('',#39340,#9380);
#6512=LINE('',#39342,#9381);
#6513=LINE('',#39344,#9382);
#6514=LINE('',#39346,#9383);
#6515=LINE('',#39348,#9384);
#6516=LINE('',#39349,#9385);
#6517=LINE('',#39351,#9386);
#6518=LINE('',#39353,#9387);
#6519=LINE('',#39355,#9388);
#6520=LINE('',#39357,#9389);
#6521=LINE('',#39359,#9390);
#6522=LINE('',#39361,#9391);
#6523=LINE('',#39363,#9392);
#6524=LINE('',#39365,#9393);
#6525=LINE('',#39367,#9394);
#6526=LINE('',#39369,#9395);
#6527=LINE('',#39371,#9396);
#6528=LINE('',#39373,#9397);
#6529=LINE('',#39375,#9398);
#6530=LINE('',#39377,#9399);
#6531=LINE('',#39379,#9400);
#6532=LINE('',#39381,#9401);
#6533=LINE('',#39383,#9402);
#6534=LINE('',#39385,#9403);
#6535=LINE('',#39386,#9404);
#6536=LINE('',#39388,#9405);
#6537=LINE('',#39390,#9406);
#6538=LINE('',#39392,#9407);
#6539=LINE('',#39394,#9408);
#6540=LINE('',#39396,#9409);
#6541=LINE('',#39398,#9410);
#6542=LINE('',#39400,#9411);
#6543=LINE('',#39402,#9412);
#6544=LINE('',#39404,#9413);
#6545=LINE('',#39406,#9414);
#6546=LINE('',#39408,#9415);
#6547=LINE('',#39410,#9416);
#6548=LINE('',#39412,#9417);
#6549=LINE('',#39414,#9418);
#6550=LINE('',#39416,#9419);
#6551=LINE('',#39418,#9420);
#6552=LINE('',#39420,#9421);
#6553=LINE('',#39422,#9422);
#6554=LINE('',#39423,#9423);
#6555=LINE('',#39425,#9424);
#6556=LINE('',#39427,#9425);
#6557=LINE('',#39429,#9426);
#6558=LINE('',#39431,#9427);
#6559=LINE('',#39433,#9428);
#6560=LINE('',#39435,#9429);
#6561=LINE('',#39437,#9430);
#6562=LINE('',#39439,#9431);
#6563=LINE('',#39441,#9432);
#6564=LINE('',#39443,#9433);
#6565=LINE('',#39445,#9434);
#6566=LINE('',#39447,#9435);
#6567=LINE('',#39449,#9436);
#6568=LINE('',#39451,#9437);
#6569=LINE('',#39453,#9438);
#6570=LINE('',#39455,#9439);
#6571=LINE('',#39457,#9440);
#6572=LINE('',#39459,#9441);
#6573=LINE('',#39460,#9442);
#6574=LINE('',#39462,#9443);
#6575=LINE('',#39464,#9444);
#6576=LINE('',#39466,#9445);
#6577=LINE('',#39468,#9446);
#6578=LINE('',#39470,#9447);
#6579=LINE('',#39472,#9448);
#6580=LINE('',#39474,#9449);
#6581=LINE('',#39476,#9450);
#6582=LINE('',#39478,#9451);
#6583=LINE('',#39480,#9452);
#6584=LINE('',#39482,#9453);
#6585=LINE('',#39484,#9454);
#6586=LINE('',#39486,#9455);
#6587=LINE('',#39488,#9456);
#6588=LINE('',#39490,#9457);
#6589=LINE('',#39492,#9458);
#6590=LINE('',#39494,#9459);
#6591=LINE('',#39496,#9460);
#6592=LINE('',#39497,#9461);
#6593=LINE('',#39499,#9462);
#6594=LINE('',#39501,#9463);
#6595=LINE('',#39503,#9464);
#6596=LINE('',#39505,#9465);
#6597=LINE('',#39507,#9466);
#6598=LINE('',#39509,#9467);
#6599=LINE('',#39511,#9468);
#6600=LINE('',#39513,#9469);
#6601=LINE('',#39515,#9470);
#6602=LINE('',#39517,#9471);
#6603=LINE('',#39519,#9472);
#6604=LINE('',#39521,#9473);
#6605=LINE('',#39523,#9474);
#6606=LINE('',#39525,#9475);
#6607=LINE('',#39527,#9476);
#6608=LINE('',#39529,#9477);
#6609=LINE('',#39531,#9478);
#6610=LINE('',#39533,#9479);
#6611=LINE('',#39534,#9480);
#6612=LINE('',#39539,#9481);
#6613=LINE('',#39540,#9482);
#6614=LINE('',#39541,#9483);
#6615=LINE('',#39544,#9484);
#6616=LINE('',#39546,#9485);
#6617=LINE('',#39547,#9486);
#6618=LINE('',#39550,#9487);
#6619=LINE('',#39551,#9488);
#6620=LINE('',#39552,#9489);
#6621=LINE('',#39555,#9490);
#6622=LINE('',#39557,#9491);
#6623=LINE('',#39558,#9492);
#6624=LINE('',#39561,#9493);
#6625=LINE('',#39562,#9494);
#6626=LINE('',#39563,#9495);
#6627=LINE('',#39566,#9496);
#6628=LINE('',#39568,#9497);
#6629=LINE('',#39569,#9498);
#6630=LINE('',#39572,#9499);
#6631=LINE('',#39573,#9500);
#6632=LINE('',#39574,#9501);
#6633=LINE('',#39577,#9502);
#6634=LINE('',#39579,#9503);
#6635=LINE('',#39580,#9504);
#6636=LINE('',#39583,#9505);
#6637=LINE('',#39584,#9506);
#6638=LINE('',#39585,#9507);
#6639=LINE('',#39588,#9508);
#6640=LINE('',#39590,#9509);
#6641=LINE('',#39591,#9510);
#6642=LINE('',#39594,#9511);
#6643=LINE('',#39595,#9512);
#6644=LINE('',#39596,#9513);
#6645=LINE('',#39599,#9514);
#6646=LINE('',#39601,#9515);
#6647=LINE('',#39602,#9516);
#6648=LINE('',#39605,#9517);
#6649=LINE('',#39606,#9518);
#6650=LINE('',#39607,#9519);
#6651=LINE('',#39610,#9520);
#6652=LINE('',#39612,#9521);
#6653=LINE('',#39613,#9522);
#6654=LINE('',#39616,#9523);
#6655=LINE('',#39617,#9524);
#6656=LINE('',#39618,#9525);
#6657=LINE('',#39621,#9526);
#6658=LINE('',#39623,#9527);
#6659=LINE('',#39624,#9528);
#6660=LINE('',#39627,#9529);
#6661=LINE('',#39628,#9530);
#6662=LINE('',#39629,#9531);
#6663=LINE('',#39632,#9532);
#6664=LINE('',#39634,#9533);
#6665=LINE('',#39635,#9534);
#6666=LINE('',#39638,#9535);
#6667=LINE('',#39639,#9536);
#6668=LINE('',#39640,#9537);
#6669=LINE('',#39643,#9538);
#6670=LINE('',#39645,#9539);
#6671=LINE('',#39646,#9540);
#6672=LINE('',#39649,#9541);
#6673=LINE('',#39650,#9542);
#6674=LINE('',#39651,#9543);
#6675=LINE('',#39654,#9544);
#6676=LINE('',#39656,#9545);
#6677=LINE('',#39657,#9546);
#6678=LINE('',#39660,#9547);
#6679=LINE('',#39661,#9548);
#6680=LINE('',#39662,#9549);
#6681=LINE('',#39664,#9550);
#6682=LINE('',#39665,#9551);
#6683=LINE('',#39667,#9552);
#6684=LINE('',#39670,#9553);
#6685=LINE('',#39672,#9554);
#6686=LINE('',#39674,#9555);
#6687=LINE('',#39676,#9556);
#6688=LINE('',#39678,#9557);
#6689=LINE('',#39680,#9558);
#6690=LINE('',#39682,#9559);
#6691=LINE('',#39684,#9560);
#6692=LINE('',#39686,#9561);
#6693=LINE('',#39688,#9562);
#6694=LINE('',#39690,#9563);
#6695=LINE('',#39692,#9564);
#6696=LINE('',#39694,#9565);
#6697=LINE('',#39696,#9566);
#6698=LINE('',#39698,#9567);
#6699=LINE('',#39701,#9568);
#6700=LINE('',#39703,#9569);
#6701=LINE('',#39705,#9570);
#6702=LINE('',#39708,#9571);
#6703=LINE('',#39710,#9572);
#6704=LINE('',#39712,#9573);
#6705=LINE('',#39714,#9574);
#6706=LINE('',#39716,#9575);
#6707=LINE('',#39718,#9576);
#6708=LINE('',#39720,#9577);
#6709=LINE('',#39722,#9578);
#6710=LINE('',#39724,#9579);
#6711=LINE('',#39726,#9580);
#6712=LINE('',#39728,#9581);
#6713=LINE('',#39730,#9582);
#6714=LINE('',#39732,#9583);
#6715=LINE('',#39734,#9584);
#6716=LINE('',#39736,#9585);
#6717=LINE('',#39739,#9586);
#6718=LINE('',#39741,#9587);
#6719=LINE('',#39743,#9588);
#6720=LINE('',#39746,#9589);
#6721=LINE('',#39748,#9590);
#6722=LINE('',#39750,#9591);
#6723=LINE('',#39752,#9592);
#6724=LINE('',#39754,#9593);
#6725=LINE('',#39756,#9594);
#6726=LINE('',#39758,#9595);
#6727=LINE('',#39760,#9596);
#6728=LINE('',#39762,#9597);
#6729=LINE('',#39764,#9598);
#6730=LINE('',#39766,#9599);
#6731=LINE('',#39768,#9600);
#6732=LINE('',#39770,#9601);
#6733=LINE('',#39772,#9602);
#6734=LINE('',#39774,#9603);
#6735=LINE('',#39777,#9604);
#6736=LINE('',#39779,#9605);
#6737=LINE('',#39781,#9606);
#6738=LINE('',#39784,#9607);
#6739=LINE('',#39786,#9608);
#6740=LINE('',#39788,#9609);
#6741=LINE('',#39790,#9610);
#6742=LINE('',#39792,#9611);
#6743=LINE('',#39794,#9612);
#6744=LINE('',#39796,#9613);
#6745=LINE('',#39798,#9614);
#6746=LINE('',#39800,#9615);
#6747=LINE('',#39802,#9616);
#6748=LINE('',#39804,#9617);
#6749=LINE('',#39806,#9618);
#6750=LINE('',#39808,#9619);
#6751=LINE('',#39810,#9620);
#6752=LINE('',#39812,#9621);
#6753=LINE('',#39815,#9622);
#6754=LINE('',#39817,#9623);
#6755=LINE('',#39819,#9624);
#6756=LINE('',#39822,#9625);
#6757=LINE('',#39824,#9626);
#6758=LINE('',#39826,#9627);
#6759=LINE('',#39828,#9628);
#6760=LINE('',#39830,#9629);
#6761=LINE('',#39832,#9630);
#6762=LINE('',#39834,#9631);
#6763=LINE('',#39836,#9632);
#6764=LINE('',#39838,#9633);
#6765=LINE('',#39840,#9634);
#6766=LINE('',#39842,#9635);
#6767=LINE('',#39844,#9636);
#6768=LINE('',#39846,#9637);
#6769=LINE('',#39848,#9638);
#6770=LINE('',#39850,#9639);
#6771=LINE('',#39853,#9640);
#6772=LINE('',#39855,#9641);
#6773=LINE('',#39857,#9642);
#6774=LINE('',#39860,#9643);
#6775=LINE('',#39862,#9644);
#6776=LINE('',#39864,#9645);
#6777=LINE('',#39866,#9646);
#6778=LINE('',#39868,#9647);
#6779=LINE('',#39870,#9648);
#6780=LINE('',#39872,#9649);
#6781=LINE('',#39874,#9650);
#6782=LINE('',#39876,#9651);
#6783=LINE('',#39878,#9652);
#6784=LINE('',#39880,#9653);
#6785=LINE('',#39882,#9654);
#6786=LINE('',#39884,#9655);
#6787=LINE('',#39886,#9656);
#6788=LINE('',#39888,#9657);
#6789=LINE('',#39891,#9658);
#6790=LINE('',#39893,#9659);
#6791=LINE('',#39895,#9660);
#6792=LINE('',#39898,#9661);
#6793=LINE('',#39900,#9662);
#6794=LINE('',#39902,#9663);
#6795=LINE('',#39904,#9664);
#6796=LINE('',#39906,#9665);
#6797=LINE('',#39908,#9666);
#6798=LINE('',#39910,#9667);
#6799=LINE('',#39912,#9668);
#6800=LINE('',#39914,#9669);
#6801=LINE('',#39916,#9670);
#6802=LINE('',#39918,#9671);
#6803=LINE('',#39920,#9672);
#6804=LINE('',#39922,#9673);
#6805=LINE('',#39924,#9674);
#6806=LINE('',#39926,#9675);
#6807=LINE('',#39929,#9676);
#6808=LINE('',#39931,#9677);
#6809=LINE('',#39933,#9678);
#6810=LINE('',#39936,#9679);
#6811=LINE('',#39938,#9680);
#6812=LINE('',#39940,#9681);
#6813=LINE('',#39942,#9682);
#6814=LINE('',#39944,#9683);
#6815=LINE('',#39946,#9684);
#6816=LINE('',#39948,#9685);
#6817=LINE('',#39950,#9686);
#6818=LINE('',#39952,#9687);
#6819=LINE('',#39954,#9688);
#6820=LINE('',#39956,#9689);
#6821=LINE('',#39958,#9690);
#6822=LINE('',#39960,#9691);
#6823=LINE('',#39962,#9692);
#6824=LINE('',#39964,#9693);
#6825=LINE('',#39967,#9694);
#6826=LINE('',#39969,#9695);
#6827=LINE('',#39971,#9696);
#6828=LINE('',#39974,#9697);
#6829=LINE('',#39976,#9698);
#6830=LINE('',#39978,#9699);
#6831=LINE('',#39980,#9700);
#6832=LINE('',#39982,#9701);
#6833=LINE('',#39984,#9702);
#6834=LINE('',#39986,#9703);
#6835=LINE('',#39988,#9704);
#6836=LINE('',#39990,#9705);
#6837=LINE('',#39992,#9706);
#6838=LINE('',#39994,#9707);
#6839=LINE('',#39996,#9708);
#6840=LINE('',#39998,#9709);
#6841=LINE('',#40000,#9710);
#6842=LINE('',#40002,#9711);
#6843=LINE('',#40005,#9712);
#6844=LINE('',#40007,#9713);
#6845=LINE('',#40009,#9714);
#6846=LINE('',#40012,#9715);
#6847=LINE('',#40014,#9716);
#6848=LINE('',#40016,#9717);
#6849=LINE('',#40018,#9718);
#6850=LINE('',#40020,#9719);
#6851=LINE('',#40022,#9720);
#6852=LINE('',#40024,#9721);
#6853=LINE('',#40026,#9722);
#6854=LINE('',#40028,#9723);
#6855=LINE('',#40030,#9724);
#6856=LINE('',#40032,#9725);
#6857=LINE('',#40034,#9726);
#6858=LINE('',#40036,#9727);
#6859=LINE('',#40038,#9728);
#6860=LINE('',#40040,#9729);
#6861=LINE('',#40043,#9730);
#6862=LINE('',#40045,#9731);
#6863=LINE('',#40047,#9732);
#6864=LINE('',#40050,#9733);
#6865=LINE('',#40052,#9734);
#6866=LINE('',#40054,#9735);
#6867=LINE('',#40056,#9736);
#6868=LINE('',#40058,#9737);
#6869=LINE('',#40060,#9738);
#6870=LINE('',#40062,#9739);
#6871=LINE('',#40064,#9740);
#6872=LINE('',#40066,#9741);
#6873=LINE('',#40068,#9742);
#6874=LINE('',#40070,#9743);
#6875=LINE('',#40072,#9744);
#6876=LINE('',#40074,#9745);
#6877=LINE('',#40076,#9746);
#6878=LINE('',#40078,#9747);
#6879=LINE('',#40081,#9748);
#6880=LINE('',#40083,#9749);
#6881=LINE('',#40085,#9750);
#6882=LINE('',#40088,#9751);
#6883=LINE('',#40090,#9752);
#6884=LINE('',#40092,#9753);
#6885=LINE('',#40094,#9754);
#6886=LINE('',#40096,#9755);
#6887=LINE('',#40098,#9756);
#6888=LINE('',#40100,#9757);
#6889=LINE('',#40102,#9758);
#6890=LINE('',#40104,#9759);
#6891=LINE('',#40106,#9760);
#6892=LINE('',#40108,#9761);
#6893=LINE('',#40110,#9762);
#6894=LINE('',#40112,#9763);
#6895=LINE('',#40114,#9764);
#6896=LINE('',#40116,#9765);
#6897=LINE('',#40121,#9766);
#6898=LINE('',#40127,#9767);
#8758=VECTOR('',#30206,10.);
#8759=VECTOR('',#30207,10.);
#8760=VECTOR('',#30208,10.);
#8761=VECTOR('',#30209,10.);
#8762=VECTOR('',#30210,10.);
#8763=VECTOR('',#30211,10.);
#8764=VECTOR('',#30214,10.);
#8765=VECTOR('',#30215,10.);
#8766=VECTOR('',#30216,10.);
#8767=VECTOR('',#30217,10.);
#8768=VECTOR('',#30218,10.);
#8769=VECTOR('',#30219,10.);
#8770=VECTOR('',#30220,10.);
#8771=VECTOR('',#30221,10.);
#8772=VECTOR('',#30222,10.);
#8773=VECTOR('',#30223,10.);
#8774=VECTOR('',#30224,10.);
#8775=VECTOR('',#30225,10.);
#8776=VECTOR('',#30226,10.);
#8777=VECTOR('',#30227,10.);
#8778=VECTOR('',#30228,10.);
#8779=VECTOR('',#30229,10.);
#8780=VECTOR('',#30230,10.);
#8781=VECTOR('',#30231,10.);
#8782=VECTOR('',#30232,10.);
#8783=VECTOR('',#30233,10.);
#8784=VECTOR('',#30234,10.);
#8785=VECTOR('',#30235,10.);
#8786=VECTOR('',#30236,10.);
#8787=VECTOR('',#30237,10.);
#8788=VECTOR('',#30238,10.);
#8789=VECTOR('',#30239,10.);
#8790=VECTOR('',#30240,10.);
#8791=VECTOR('',#30241,10.);
#8792=VECTOR('',#30242,10.);
#8793=VECTOR('',#30243,10.);
#8794=VECTOR('',#30244,10.);
#8795=VECTOR('',#30245,10.);
#8796=VECTOR('',#30246,10.);
#8797=VECTOR('',#30247,10.);
#8798=VECTOR('',#30248,10.);
#8799=VECTOR('',#30249,10.);
#8800=VECTOR('',#30250,10.);
#8801=VECTOR('',#30251,10.);
#8802=VECTOR('',#30252,10.);
#8803=VECTOR('',#30253,10.);
#8804=VECTOR('',#30254,10.);
#8805=VECTOR('',#30255,10.);
#8806=VECTOR('',#30256,10.);
#8807=VECTOR('',#30257,10.);
#8808=VECTOR('',#30258,10.);
#8809=VECTOR('',#30259,10.);
#8810=VECTOR('',#30260,10.);
#8811=VECTOR('',#30261,10.);
#8812=VECTOR('',#30262,10.);
#8813=VECTOR('',#30263,10.);
#8814=VECTOR('',#30264,10.);
#8815=VECTOR('',#30265,10.);
#8816=VECTOR('',#30266,10.);
#8817=VECTOR('',#30267,10.);
#8818=VECTOR('',#30268,10.);
#8819=VECTOR('',#30269,10.);
#8820=VECTOR('',#30270,10.);
#8821=VECTOR('',#30271,10.);
#8822=VECTOR('',#30272,10.);
#8823=VECTOR('',#30273,10.);
#8824=VECTOR('',#30274,10.);
#8825=VECTOR('',#30275,10.);
#8826=VECTOR('',#30276,10.);
#8827=VECTOR('',#30277,10.);
#8828=VECTOR('',#30278,10.);
#8829=VECTOR('',#30279,10.);
#8830=VECTOR('',#30280,10.);
#8831=VECTOR('',#30281,10.);
#8832=VECTOR('',#30282,10.);
#8833=VECTOR('',#30283,10.);
#8834=VECTOR('',#30284,10.);
#8835=VECTOR('',#30285,10.);
#8836=VECTOR('',#30286,10.);
#8837=VECTOR('',#30287,10.);
#8838=VECTOR('',#30288,10.);
#8839=VECTOR('',#30289,10.);
#8840=VECTOR('',#30290,10.);
#8841=VECTOR('',#30291,10.);
#8842=VECTOR('',#30292,10.);
#8843=VECTOR('',#30293,10.);
#8844=VECTOR('',#30294,10.);
#8845=VECTOR('',#30295,10.);
#8846=VECTOR('',#30296,10.);
#8847=VECTOR('',#30297,10.);
#8848=VECTOR('',#30298,10.);
#8849=VECTOR('',#30299,10.);
#8850=VECTOR('',#30300,10.);
#8851=VECTOR('',#30301,10.);
#8852=VECTOR('',#30302,10.);
#8853=VECTOR('',#30303,10.);
#8854=VECTOR('',#30304,10.);
#8855=VECTOR('',#30305,10.);
#8856=VECTOR('',#30306,10.);
#8857=VECTOR('',#30307,10.);
#8858=VECTOR('',#30308,10.);
#8859=VECTOR('',#30309,10.);
#8860=VECTOR('',#30310,10.);
#8861=VECTOR('',#30311,10.);
#8862=VECTOR('',#30312,10.);
#8863=VECTOR('',#30313,10.);
#8864=VECTOR('',#30314,10.);
#8865=VECTOR('',#30315,10.);
#8866=VECTOR('',#30316,10.);
#8867=VECTOR('',#30317,10.);
#8868=VECTOR('',#30318,10.);
#8869=VECTOR('',#30319,10.);
#8870=VECTOR('',#30320,10.);
#8871=VECTOR('',#30321,10.);
#8872=VECTOR('',#30322,10.);
#8873=VECTOR('',#30323,10.);
#8874=VECTOR('',#30324,10.);
#8875=VECTOR('',#30325,10.);
#8876=VECTOR('',#30326,10.);
#8877=VECTOR('',#30327,10.);
#8878=VECTOR('',#30328,10.);
#8879=VECTOR('',#30329,10.);
#8880=VECTOR('',#30330,10.);
#8881=VECTOR('',#30331,10.);
#8882=VECTOR('',#30332,10.);
#8883=VECTOR('',#30333,10.);
#8884=VECTOR('',#30334,10.);
#8885=VECTOR('',#30335,10.);
#8886=VECTOR('',#30336,10.);
#8887=VECTOR('',#30337,10.);
#8888=VECTOR('',#30338,10.);
#8889=VECTOR('',#30339,10.);
#8890=VECTOR('',#30340,10.);
#8891=VECTOR('',#30341,10.);
#8892=VECTOR('',#30342,10.);
#8893=VECTOR('',#30343,10.);
#8894=VECTOR('',#30344,10.);
#8895=VECTOR('',#30345,10.);
#8896=VECTOR('',#30346,10.);
#8897=VECTOR('',#30347,10.);
#8898=VECTOR('',#30348,10.);
#8899=VECTOR('',#30349,10.);
#8900=VECTOR('',#30350,10.);
#8901=VECTOR('',#30351,10.);
#8902=VECTOR('',#30352,10.);
#8903=VECTOR('',#30353,10.);
#8904=VECTOR('',#30354,10.);
#8905=VECTOR('',#30355,10.);
#8906=VECTOR('',#30356,10.);
#8907=VECTOR('',#30357,10.);
#8908=VECTOR('',#30358,10.);
#8909=VECTOR('',#30359,10.);
#8910=VECTOR('',#30360,10.);
#8911=VECTOR('',#30361,10.);
#8912=VECTOR('',#30362,10.);
#8913=VECTOR('',#30363,10.);
#8914=VECTOR('',#30364,10.);
#8915=VECTOR('',#30365,10.);
#8916=VECTOR('',#30366,10.);
#8917=VECTOR('',#30367,10.);
#8918=VECTOR('',#30368,10.);
#8919=VECTOR('',#30369,10.);
#8920=VECTOR('',#30370,10.);
#8921=VECTOR('',#30371,10.);
#8922=VECTOR('',#30372,10.);
#8923=VECTOR('',#30373,10.);
#8924=VECTOR('',#30374,10.);
#8925=VECTOR('',#30375,10.);
#8926=VECTOR('',#30376,10.);
#8927=VECTOR('',#30377,10.);
#8928=VECTOR('',#30378,10.);
#8929=VECTOR('',#30379,10.);
#8930=VECTOR('',#30380,10.);
#8931=VECTOR('',#30381,10.);
#8932=VECTOR('',#30382,10.);
#8933=VECTOR('',#30383,10.);
#8934=VECTOR('',#30384,10.);
#8935=VECTOR('',#30385,10.);
#8936=VECTOR('',#30386,10.);
#8937=VECTOR('',#30387,10.);
#8938=VECTOR('',#30388,10.);
#8939=VECTOR('',#30389,10.);
#8940=VECTOR('',#30390,10.);
#8941=VECTOR('',#30391,10.);
#8942=VECTOR('',#30392,10.);
#8943=VECTOR('',#30393,10.);
#8944=VECTOR('',#30394,10.);
#8945=VECTOR('',#30395,10.);
#8946=VECTOR('',#30396,10.);
#8947=VECTOR('',#30397,10.);
#8948=VECTOR('',#30398,10.);
#8949=VECTOR('',#30399,10.);
#8950=VECTOR('',#30400,10.);
#8951=VECTOR('',#30401,10.);
#8952=VECTOR('',#30402,10.);
#8953=VECTOR('',#30403,10.);
#8954=VECTOR('',#30404,10.);
#8955=VECTOR('',#30405,10.);
#8956=VECTOR('',#30406,10.);
#8957=VECTOR('',#30407,10.);
#8958=VECTOR('',#30408,10.);
#8959=VECTOR('',#30409,10.);
#8960=VECTOR('',#30410,10.);
#8961=VECTOR('',#30411,10.);
#8962=VECTOR('',#30412,10.);
#8963=VECTOR('',#30413,10.);
#8964=VECTOR('',#30414,10.);
#8965=VECTOR('',#30415,10.);
#8966=VECTOR('',#30416,10.);
#8967=VECTOR('',#30417,10.);
#8968=VECTOR('',#30418,10.);
#8969=VECTOR('',#30419,10.);
#8970=VECTOR('',#30420,10.);
#8971=VECTOR('',#30421,10.);
#8972=VECTOR('',#30422,10.);
#8973=VECTOR('',#30423,10.);
#8974=VECTOR('',#30424,10.);
#8975=VECTOR('',#30425,10.);
#8976=VECTOR('',#30426,10.);
#8977=VECTOR('',#30427,10.);
#8978=VECTOR('',#30428,10.);
#8979=VECTOR('',#30429,10.);
#8980=VECTOR('',#30430,10.);
#8981=VECTOR('',#30431,10.);
#8982=VECTOR('',#30432,10.);
#8983=VECTOR('',#30433,10.);
#8984=VECTOR('',#30434,10.);
#8985=VECTOR('',#30435,10.);
#8986=VECTOR('',#30436,10.);
#8987=VECTOR('',#30437,10.);
#8988=VECTOR('',#30438,10.);
#8989=VECTOR('',#30439,10.);
#8990=VECTOR('',#30440,10.);
#8991=VECTOR('',#30441,10.);
#8992=VECTOR('',#30442,10.);
#8993=VECTOR('',#30443,10.);
#8994=VECTOR('',#30444,10.);
#8995=VECTOR('',#30445,10.);
#8996=VECTOR('',#30446,10.);
#8997=VECTOR('',#30447,10.);
#8998=VECTOR('',#30448,10.);
#8999=VECTOR('',#30449,10.);
#9000=VECTOR('',#30450,10.);
#9001=VECTOR('',#30451,10.);
#9002=VECTOR('',#30452,10.);
#9003=VECTOR('',#30457,10.);
#9004=VECTOR('',#30458,10.);
#9005=VECTOR('',#30459,10.);
#9006=VECTOR('',#30460,10.);
#9007=VECTOR('',#30463,10.);
#9008=VECTOR('',#30464,10.);
#9009=VECTOR('',#30467,10.);
#9010=VECTOR('',#30468,10.);
#9011=VECTOR('',#30469,10.);
#9012=VECTOR('',#30470,10.);
#9013=VECTOR('',#30471,10.);
#9014=VECTOR('',#30474,10.);
#9015=VECTOR('',#30475,10.);
#9016=VECTOR('',#30476,10.);
#9017=VECTOR('',#30477,10.);
#9018=VECTOR('',#30480,10.);
#9019=VECTOR('',#30481,10.);
#9020=VECTOR('',#30484,10.);
#9021=VECTOR('',#30485,10.);
#9022=VECTOR('',#30486,10.);
#9023=VECTOR('',#30487,10.);
#9024=VECTOR('',#30488,10.);
#9025=VECTOR('',#30491,10.);
#9026=VECTOR('',#30492,10.);
#9027=VECTOR('',#30493,10.);
#9028=VECTOR('',#30494,10.);
#9029=VECTOR('',#30497,10.);
#9030=VECTOR('',#30498,10.);
#9031=VECTOR('',#30501,10.);
#9032=VECTOR('',#30502,10.);
#9033=VECTOR('',#30503,10.);
#9034=VECTOR('',#30504,10.);
#9035=VECTOR('',#30505,10.);
#9036=VECTOR('',#30508,10.);
#9037=VECTOR('',#30509,10.);
#9038=VECTOR('',#30510,10.);
#9039=VECTOR('',#30511,10.);
#9040=VECTOR('',#30514,10.);
#9041=VECTOR('',#30515,10.);
#9042=VECTOR('',#30518,10.);
#9043=VECTOR('',#30519,10.);
#9044=VECTOR('',#30520,10.);
#9045=VECTOR('',#30521,10.);
#9046=VECTOR('',#30522,10.);
#9047=VECTOR('',#30525,10.);
#9048=VECTOR('',#30526,10.);
#9049=VECTOR('',#30527,10.);
#9050=VECTOR('',#30528,10.);
#9051=VECTOR('',#30531,10.);
#9052=VECTOR('',#30532,10.);
#9053=VECTOR('',#30535,10.);
#9054=VECTOR('',#30536,10.);
#9055=VECTOR('',#30537,10.);
#9056=VECTOR('',#30538,10.);
#9057=VECTOR('',#30539,10.);
#9058=VECTOR('',#30542,10.);
#9059=VECTOR('',#30543,10.);
#9060=VECTOR('',#30544,10.);
#9061=VECTOR('',#30545,10.);
#9062=VECTOR('',#30548,10.);
#9063=VECTOR('',#30549,10.);
#9064=VECTOR('',#30552,10.);
#9065=VECTOR('',#30553,10.);
#9066=VECTOR('',#30554,10.);
#9067=VECTOR('',#30555,10.);
#9068=VECTOR('',#30556,10.);
#9069=VECTOR('',#30559,10.);
#9070=VECTOR('',#30560,10.);
#9071=VECTOR('',#30561,10.);
#9072=VECTOR('',#30562,10.);
#9073=VECTOR('',#30565,10.);
#9074=VECTOR('',#30566,10.);
#9075=VECTOR('',#30569,10.);
#9076=VECTOR('',#30570,10.);
#9077=VECTOR('',#30571,10.);
#9078=VECTOR('',#30572,10.);
#9079=VECTOR('',#30573,10.);
#9080=VECTOR('',#30576,10.);
#9081=VECTOR('',#30577,10.);
#9082=VECTOR('',#30578,10.);
#9083=VECTOR('',#30579,10.);
#9084=VECTOR('',#30582,10.);
#9085=VECTOR('',#30583,10.);
#9086=VECTOR('',#30586,10.);
#9087=VECTOR('',#30587,10.);
#9088=VECTOR('',#30588,10.);
#9089=VECTOR('',#30589,10.);
#9090=VECTOR('',#30590,10.);
#9091=VECTOR('',#30593,10.);
#9092=VECTOR('',#30594,10.);
#9093=VECTOR('',#30595,10.);
#9094=VECTOR('',#30596,10.);
#9095=VECTOR('',#30599,10.);
#9096=VECTOR('',#30600,10.);
#9097=VECTOR('',#30603,10.);
#9098=VECTOR('',#30604,10.);
#9099=VECTOR('',#30605,10.);
#9100=VECTOR('',#30606,10.);
#9101=VECTOR('',#30607,10.);
#9102=VECTOR('',#30610,10.);
#9103=VECTOR('',#30611,10.);
#9104=VECTOR('',#30612,10.);
#9105=VECTOR('',#30613,10.);
#9106=VECTOR('',#30616,10.);
#9107=VECTOR('',#30617,10.);
#9108=VECTOR('',#30620,10.);
#9109=VECTOR('',#30621,10.);
#9110=VECTOR('',#30622,10.);
#9111=VECTOR('',#30623,10.);
#9112=VECTOR('',#30624,10.);
#9113=VECTOR('',#30627,10.);
#9114=VECTOR('',#30628,10.);
#9115=VECTOR('',#30629,10.);
#9116=VECTOR('',#30630,10.);
#9117=VECTOR('',#30633,10.);
#9118=VECTOR('',#30634,10.);
#9119=VECTOR('',#30637,10.);
#9120=VECTOR('',#30638,10.);
#9121=VECTOR('',#30639,10.);
#9122=VECTOR('',#30640,10.);
#9123=VECTOR('',#30641,10.);
#9124=VECTOR('',#30644,10.);
#9125=VECTOR('',#30645,10.);
#9126=VECTOR('',#30646,10.);
#9127=VECTOR('',#30647,10.);
#9128=VECTOR('',#30650,10.);
#9129=VECTOR('',#30651,10.);
#9130=VECTOR('',#30654,10.);
#9131=VECTOR('',#30655,10.);
#9132=VECTOR('',#30656,10.);
#9133=VECTOR('',#30657,10.);
#9134=VECTOR('',#30658,10.);
#9135=VECTOR('',#30661,10.);
#9136=VECTOR('',#30662,10.);
#9137=VECTOR('',#30663,10.);
#9138=VECTOR('',#30666,10.);
#9139=VECTOR('',#30667,10.);
#9140=VECTOR('',#30670,10.);
#9141=VECTOR('',#30671,10.);
#9142=VECTOR('',#30672,10.);
#9143=VECTOR('',#30673,10.);
#9144=VECTOR('',#30674,10.);
#9145=VECTOR('',#30677,10.);
#9146=VECTOR('',#30678,10.);
#9147=VECTOR('',#30679,10.);
#9148=VECTOR('',#30682,10.);
#9149=VECTOR('',#30683,10.);
#9150=VECTOR('',#30686,10.);
#9151=VECTOR('',#30687,10.);
#9152=VECTOR('',#30688,10.);
#9153=VECTOR('',#30689,10.);
#9154=VECTOR('',#30690,10.);
#9155=VECTOR('',#30693,10.);
#9156=VECTOR('',#30694,10.);
#9157=VECTOR('',#30695,10.);
#9158=VECTOR('',#30698,10.);
#9159=VECTOR('',#30699,10.);
#9160=VECTOR('',#30702,10.);
#9161=VECTOR('',#30703,10.);
#9162=VECTOR('',#30704,10.);
#9163=VECTOR('',#30705,10.);
#9164=VECTOR('',#30706,10.);
#9165=VECTOR('',#30709,10.);
#9166=VECTOR('',#30710,10.);
#9167=VECTOR('',#30711,10.);
#9168=VECTOR('',#30714,10.);
#9169=VECTOR('',#30715,10.);
#9170=VECTOR('',#30718,10.);
#9171=VECTOR('',#30719,10.);
#9172=VECTOR('',#30720,10.);
#9173=VECTOR('',#30721,10.);
#9174=VECTOR('',#30722,10.);
#9175=VECTOR('',#30725,10.);
#9176=VECTOR('',#30726,10.);
#9177=VECTOR('',#30727,10.);
#9178=VECTOR('',#30730,10.);
#9179=VECTOR('',#30731,10.);
#9180=VECTOR('',#30734,10.);
#9181=VECTOR('',#30735,10.);
#9182=VECTOR('',#30736,10.);
#9183=VECTOR('',#30737,10.);
#9184=VECTOR('',#30738,10.);
#9185=VECTOR('',#30741,10.);
#9186=VECTOR('',#30742,10.);
#9187=VECTOR('',#30743,10.);
#9188=VECTOR('',#30746,10.);
#9189=VECTOR('',#30747,10.);
#9190=VECTOR('',#30750,10.);
#9191=VECTOR('',#30751,10.);
#9192=VECTOR('',#30752,10.);
#9193=VECTOR('',#30753,10.);
#9194=VECTOR('',#30754,10.);
#9195=VECTOR('',#30757,10.);
#9196=VECTOR('',#30758,10.);
#9197=VECTOR('',#30759,10.);
#9198=VECTOR('',#30762,10.);
#9199=VECTOR('',#30763,10.);
#9200=VECTOR('',#30766,10.);
#9201=VECTOR('',#30767,10.);
#9202=VECTOR('',#30768,10.);
#9203=VECTOR('',#30769,10.);
#9204=VECTOR('',#30770,10.);
#9205=VECTOR('',#30773,10.);
#9206=VECTOR('',#30774,10.);
#9207=VECTOR('',#30775,10.);
#9208=VECTOR('',#30778,10.);
#9209=VECTOR('',#30779,10.);
#9210=VECTOR('',#30782,10.);
#9211=VECTOR('',#30783,10.);
#9212=VECTOR('',#30784,10.);
#9213=VECTOR('',#30785,10.);
#9214=VECTOR('',#30786,10.);
#9215=VECTOR('',#30789,10.);
#9216=VECTOR('',#30790,10.);
#9217=VECTOR('',#30791,10.);
#9218=VECTOR('',#30794,10.);
#9219=VECTOR('',#30795,10.);
#9220=VECTOR('',#30798,10.);
#9221=VECTOR('',#30799,10.);
#9222=VECTOR('',#30800,10.);
#9223=VECTOR('',#30801,10.);
#9224=VECTOR('',#30802,10.);
#9225=VECTOR('',#30805,10.);
#9226=VECTOR('',#30806,10.);
#9227=VECTOR('',#30807,10.);
#9228=VECTOR('',#30810,10.);
#9229=VECTOR('',#30811,10.);
#9230=VECTOR('',#30814,10.);
#9231=VECTOR('',#30815,10.);
#9232=VECTOR('',#30816,10.);
#9233=VECTOR('',#30817,10.);
#9234=VECTOR('',#30818,10.);
#9235=VECTOR('',#30821,10.);
#9236=VECTOR('',#30822,10.);
#9237=VECTOR('',#30823,10.);
#9238=VECTOR('',#30826,10.);
#9239=VECTOR('',#30827,10.);
#9240=VECTOR('',#30830,10.);
#9241=VECTOR('',#30831,10.);
#9242=VECTOR('',#30832,10.);
#9243=VECTOR('',#30833,10.);
#9244=VECTOR('',#30834,10.);
#9245=VECTOR('',#30837,10.);
#9246=VECTOR('',#30838,10.);
#9247=VECTOR('',#30839,10.);
#9248=VECTOR('',#30842,10.);
#9249=VECTOR('',#30843,10.);
#9250=VECTOR('',#30846,10.);
#9251=VECTOR('',#30847,10.);
#9252=VECTOR('',#30848,10.);
#9253=VECTOR('',#30849,10.);
#9254=VECTOR('',#30852,10.);
#9255=VECTOR('',#30853,10.);
#9256=VECTOR('',#30854,10.);
#9257=VECTOR('',#30855,10.);
#9258=VECTOR('',#30856,10.);
#9259=VECTOR('',#30857,10.);
#9260=VECTOR('',#30858,10.);
#9261=VECTOR('',#30859,10.);
#9262=VECTOR('',#30860,10.);
#9263=VECTOR('',#30861,10.);
#9264=VECTOR('',#30862,10.);
#9265=VECTOR('',#30863,10.);
#9266=VECTOR('',#30864,10.);
#9267=VECTOR('',#30865,10.);
#9268=VECTOR('',#30866,10.);
#9269=VECTOR('',#30867,10.);
#9270=VECTOR('',#30868,10.);
#9271=VECTOR('',#30869,10.);
#9272=VECTOR('',#30870,10.);
#9273=VECTOR('',#30871,10.);
#9274=VECTOR('',#30872,10.);
#9275=VECTOR('',#30873,10.);
#9276=VECTOR('',#30874,10.);
#9277=VECTOR('',#30875,10.);
#9278=VECTOR('',#30876,10.);
#9279=VECTOR('',#30877,10.);
#9280=VECTOR('',#30878,10.);
#9281=VECTOR('',#30879,10.);
#9282=VECTOR('',#30880,10.);
#9283=VECTOR('',#30881,10.);
#9284=VECTOR('',#30882,10.);
#9285=VECTOR('',#30883,10.);
#9286=VECTOR('',#30884,10.);
#9287=VECTOR('',#30885,10.);
#9288=VECTOR('',#30886,10.);
#9289=VECTOR('',#30887,10.);
#9290=VECTOR('',#30888,10.);
#9291=VECTOR('',#30889,10.);
#9292=VECTOR('',#30890,10.);
#9293=VECTOR('',#30891,10.);
#9294=VECTOR('',#30892,10.);
#9295=VECTOR('',#30893,10.);
#9296=VECTOR('',#30894,10.);
#9297=VECTOR('',#30895,10.);
#9298=VECTOR('',#30896,10.);
#9299=VECTOR('',#30897,10.);
#9300=VECTOR('',#30898,10.);
#9301=VECTOR('',#30899,10.);
#9302=VECTOR('',#30900,10.);
#9303=VECTOR('',#30901,10.);
#9304=VECTOR('',#30902,10.);
#9305=VECTOR('',#30903,10.);
#9306=VECTOR('',#30904,10.);
#9307=VECTOR('',#30905,10.);
#9308=VECTOR('',#30906,10.);
#9309=VECTOR('',#30907,10.);
#9310=VECTOR('',#30908,10.);
#9311=VECTOR('',#30909,10.);
#9312=VECTOR('',#30910,10.);
#9313=VECTOR('',#30911,10.);
#9314=VECTOR('',#30912,10.);
#9315=VECTOR('',#30913,10.);
#9316=VECTOR('',#30914,10.);
#9317=VECTOR('',#30915,10.);
#9318=VECTOR('',#30916,10.);
#9319=VECTOR('',#30917,10.);
#9320=VECTOR('',#30918,10.);
#9321=VECTOR('',#30919,10.);
#9322=VECTOR('',#30920,10.);
#9323=VECTOR('',#30921,10.);
#9324=VECTOR('',#30922,10.);
#9325=VECTOR('',#30923,10.);
#9326=VECTOR('',#30924,10.);
#9327=VECTOR('',#30925,10.);
#9328=VECTOR('',#30926,10.);
#9329=VECTOR('',#30927,10.);
#9330=VECTOR('',#30928,10.);
#9331=VECTOR('',#30929,10.);
#9332=VECTOR('',#30930,10.);
#9333=VECTOR('',#30931,10.);
#9334=VECTOR('',#30932,10.);
#9335=VECTOR('',#30933,10.);
#9336=VECTOR('',#30934,10.);
#9337=VECTOR('',#30935,10.);
#9338=VECTOR('',#30936,10.);
#9339=VECTOR('',#30937,10.);
#9340=VECTOR('',#30938,10.);
#9341=VECTOR('',#30939,10.);
#9342=VECTOR('',#30940,10.);
#9343=VECTOR('',#30941,10.);
#9344=VECTOR('',#30942,10.);
#9345=VECTOR('',#30943,10.);
#9346=VECTOR('',#30944,10.);
#9347=VECTOR('',#30945,10.);
#9348=VECTOR('',#30946,10.);
#9349=VECTOR('',#30947,10.);
#9350=VECTOR('',#30948,10.);
#9351=VECTOR('',#30949,10.);
#9352=VECTOR('',#30950,10.);
#9353=VECTOR('',#30951,10.);
#9354=VECTOR('',#30952,10.);
#9355=VECTOR('',#30953,10.);
#9356=VECTOR('',#30954,10.);
#9357=VECTOR('',#30955,10.);
#9358=VECTOR('',#30956,10.);
#9359=VECTOR('',#30957,10.);
#9360=VECTOR('',#30958,10.);
#9361=VECTOR('',#30959,10.);
#9362=VECTOR('',#30960,10.);
#9363=VECTOR('',#30961,10.);
#9364=VECTOR('',#30962,10.);
#9365=VECTOR('',#30963,10.);
#9366=VECTOR('',#30964,10.);
#9367=VECTOR('',#30965,10.);
#9368=VECTOR('',#30966,10.);
#9369=VECTOR('',#30967,10.);
#9370=VECTOR('',#30968,10.);
#9371=VECTOR('',#30969,10.);
#9372=VECTOR('',#30970,10.);
#9373=VECTOR('',#30971,10.);
#9374=VECTOR('',#30972,10.);
#9375=VECTOR('',#30973,10.);
#9376=VECTOR('',#30974,10.);
#9377=VECTOR('',#30975,10.);
#9378=VECTOR('',#30976,10.);
#9379=VECTOR('',#30977,10.);
#9380=VECTOR('',#30978,10.);
#9381=VECTOR('',#30979,10.);
#9382=VECTOR('',#30980,10.);
#9383=VECTOR('',#30981,10.);
#9384=VECTOR('',#30982,10.);
#9385=VECTOR('',#30983,10.);
#9386=VECTOR('',#30984,10.);
#9387=VECTOR('',#30985,10.);
#9388=VECTOR('',#30986,10.);
#9389=VECTOR('',#30987,10.);
#9390=VECTOR('',#30988,10.);
#9391=VECTOR('',#30989,10.);
#9392=VECTOR('',#30990,10.);
#9393=VECTOR('',#30991,10.);
#9394=VECTOR('',#30992,10.);
#9395=VECTOR('',#30993,10.);
#9396=VECTOR('',#30994,10.);
#9397=VECTOR('',#30995,10.);
#9398=VECTOR('',#30996,10.);
#9399=VECTOR('',#30997,10.);
#9400=VECTOR('',#30998,10.);
#9401=VECTOR('',#30999,10.);
#9402=VECTOR('',#31000,10.);
#9403=VECTOR('',#31001,10.);
#9404=VECTOR('',#31002,10.);
#9405=VECTOR('',#31003,10.);
#9406=VECTOR('',#31004,10.);
#9407=VECTOR('',#31005,10.);
#9408=VECTOR('',#31006,10.);
#9409=VECTOR('',#31007,10.);
#9410=VECTOR('',#31008,10.);
#9411=VECTOR('',#31009,10.);
#9412=VECTOR('',#31010,10.);
#9413=VECTOR('',#31011,10.);
#9414=VECTOR('',#31012,10.);
#9415=VECTOR('',#31013,10.);
#9416=VECTOR('',#31014,10.);
#9417=VECTOR('',#31015,10.);
#9418=VECTOR('',#31016,10.);
#9419=VECTOR('',#31017,10.);
#9420=VECTOR('',#31018,10.);
#9421=VECTOR('',#31019,10.);
#9422=VECTOR('',#31020,10.);
#9423=VECTOR('',#31021,10.);
#9424=VECTOR('',#31022,10.);
#9425=VECTOR('',#31023,10.);
#9426=VECTOR('',#31024,10.);
#9427=VECTOR('',#31025,10.);
#9428=VECTOR('',#31026,10.);
#9429=VECTOR('',#31027,10.);
#9430=VECTOR('',#31028,10.);
#9431=VECTOR('',#31029,10.);
#9432=VECTOR('',#31030,10.);
#9433=VECTOR('',#31031,10.);
#9434=VECTOR('',#31032,10.);
#9435=VECTOR('',#31033,10.);
#9436=VECTOR('',#31034,10.);
#9437=VECTOR('',#31035,10.);
#9438=VECTOR('',#31036,10.);
#9439=VECTOR('',#31037,10.);
#9440=VECTOR('',#31038,10.);
#9441=VECTOR('',#31039,10.);
#9442=VECTOR('',#31040,10.);
#9443=VECTOR('',#31041,10.);
#9444=VECTOR('',#31042,10.);
#9445=VECTOR('',#31043,10.);
#9446=VECTOR('',#31044,10.);
#9447=VECTOR('',#31045,10.);
#9448=VECTOR('',#31046,10.);
#9449=VECTOR('',#31047,10.);
#9450=VECTOR('',#31048,10.);
#9451=VECTOR('',#31049,10.);
#9452=VECTOR('',#31050,10.);
#9453=VECTOR('',#31051,10.);
#9454=VECTOR('',#31052,10.);
#9455=VECTOR('',#31053,10.);
#9456=VECTOR('',#31054,10.);
#9457=VECTOR('',#31055,10.);
#9458=VECTOR('',#31056,10.);
#9459=VECTOR('',#31057,10.);
#9460=VECTOR('',#31058,10.);
#9461=VECTOR('',#31059,10.);
#9462=VECTOR('',#31060,10.);
#9463=VECTOR('',#31061,10.);
#9464=VECTOR('',#31062,10.);
#9465=VECTOR('',#31063,10.);
#9466=VECTOR('',#31064,10.);
#9467=VECTOR('',#31065,10.);
#9468=VECTOR('',#31066,10.);
#9469=VECTOR('',#31067,10.);
#9470=VECTOR('',#31068,10.);
#9471=VECTOR('',#31069,10.);
#9472=VECTOR('',#31070,10.);
#9473=VECTOR('',#31071,10.);
#9474=VECTOR('',#31072,10.);
#9475=VECTOR('',#31073,10.);
#9476=VECTOR('',#31074,10.);
#9477=VECTOR('',#31075,10.);
#9478=VECTOR('',#31076,10.);
#9479=VECTOR('',#31077,10.);
#9480=VECTOR('',#31078,10.);
#9481=VECTOR('',#31083,10.);
#9482=VECTOR('',#31084,10.);
#9483=VECTOR('',#31085,10.);
#9484=VECTOR('',#31088,10.);
#9485=VECTOR('',#31089,10.);
#9486=VECTOR('',#31090,10.);
#9487=VECTOR('',#31093,10.);
#9488=VECTOR('',#31094,10.);
#9489=VECTOR('',#31095,10.);
#9490=VECTOR('',#31098,10.);
#9491=VECTOR('',#31099,10.);
#9492=VECTOR('',#31100,10.);
#9493=VECTOR('',#31103,10.);
#9494=VECTOR('',#31104,10.);
#9495=VECTOR('',#31105,10.);
#9496=VECTOR('',#31108,10.);
#9497=VECTOR('',#31109,10.);
#9498=VECTOR('',#31110,10.);
#9499=VECTOR('',#31113,10.);
#9500=VECTOR('',#31114,10.);
#9501=VECTOR('',#31115,10.);
#9502=VECTOR('',#31118,10.);
#9503=VECTOR('',#31119,10.);
#9504=VECTOR('',#31120,10.);
#9505=VECTOR('',#31123,10.);
#9506=VECTOR('',#31124,10.);
#9507=VECTOR('',#31125,10.);
#9508=VECTOR('',#31128,10.);
#9509=VECTOR('',#31129,10.);
#9510=VECTOR('',#31130,10.);
#9511=VECTOR('',#31133,10.);
#9512=VECTOR('',#31134,10.);
#9513=VECTOR('',#31135,10.);
#9514=VECTOR('',#31138,10.);
#9515=VECTOR('',#31139,10.);
#9516=VECTOR('',#31140,10.);
#9517=VECTOR('',#31143,10.);
#9518=VECTOR('',#31144,10.);
#9519=VECTOR('',#31145,10.);
#9520=VECTOR('',#31148,10.);
#9521=VECTOR('',#31149,10.);
#9522=VECTOR('',#31150,10.);
#9523=VECTOR('',#31153,10.);
#9524=VECTOR('',#31154,10.);
#9525=VECTOR('',#31155,10.);
#9526=VECTOR('',#31158,10.);
#9527=VECTOR('',#31159,10.);
#9528=VECTOR('',#31160,10.);
#9529=VECTOR('',#31163,10.);
#9530=VECTOR('',#31164,10.);
#9531=VECTOR('',#31165,10.);
#9532=VECTOR('',#31168,10.);
#9533=VECTOR('',#31169,10.);
#9534=VECTOR('',#31170,10.);
#9535=VECTOR('',#31173,10.);
#9536=VECTOR('',#31174,10.);
#9537=VECTOR('',#31175,10.);
#9538=VECTOR('',#31178,10.);
#9539=VECTOR('',#31179,10.);
#9540=VECTOR('',#31180,10.);
#9541=VECTOR('',#31183,10.);
#9542=VECTOR('',#31184,10.);
#9543=VECTOR('',#31185,10.);
#9544=VECTOR('',#31188,10.);
#9545=VECTOR('',#31189,10.);
#9546=VECTOR('',#31190,10.);
#9547=VECTOR('',#31193,10.);
#9548=VECTOR('',#31194,10.);
#9549=VECTOR('',#31195,10.);
#9550=VECTOR('',#31198,10.);
#9551=VECTOR('',#31199,10.);
#9552=VECTOR('',#31202,10.);
#9553=VECTOR('',#31207,10.);
#9554=VECTOR('',#31210,10.);
#9555=VECTOR('',#31213,10.);
#9556=VECTOR('',#31216,10.);
#9557=VECTOR('',#31219,10.);
#9558=VECTOR('',#31222,10.);
#9559=VECTOR('',#31225,10.);
#9560=VECTOR('',#31228,10.);
#9561=VECTOR('',#31231,10.);
#9562=VECTOR('',#31234,10.);
#9563=VECTOR('',#31237,10.);
#9564=VECTOR('',#31240,10.);
#9565=VECTOR('',#31243,10.);
#9566=VECTOR('',#31246,10.);
#9567=VECTOR('',#31249,10.);
#9568=VECTOR('',#31254,10.);
#9569=VECTOR('',#31257,10.);
#9570=VECTOR('',#31260,10.);
#9571=VECTOR('',#31265,10.);
#9572=VECTOR('',#31268,10.);
#9573=VECTOR('',#31271,10.);
#9574=VECTOR('',#31274,10.);
#9575=VECTOR('',#31277,10.);
#9576=VECTOR('',#31280,10.);
#9577=VECTOR('',#31283,10.);
#9578=VECTOR('',#31286,10.);
#9579=VECTOR('',#31289,10.);
#9580=VECTOR('',#31292,10.);
#9581=VECTOR('',#31295,10.);
#9582=VECTOR('',#31298,10.);
#9583=VECTOR('',#31301,10.);
#9584=VECTOR('',#31304,10.);
#9585=VECTOR('',#31307,10.);
#9586=VECTOR('',#31312,10.);
#9587=VECTOR('',#31315,10.);
#9588=VECTOR('',#31318,10.);
#9589=VECTOR('',#31323,10.);
#9590=VECTOR('',#31326,10.);
#9591=VECTOR('',#31329,10.);
#9592=VECTOR('',#31332,10.);
#9593=VECTOR('',#31335,10.);
#9594=VECTOR('',#31338,10.);
#9595=VECTOR('',#31341,10.);
#9596=VECTOR('',#31344,10.);
#9597=VECTOR('',#31347,10.);
#9598=VECTOR('',#31350,10.);
#9599=VECTOR('',#31353,10.);
#9600=VECTOR('',#31356,10.);
#9601=VECTOR('',#31359,10.);
#9602=VECTOR('',#31362,10.);
#9603=VECTOR('',#31365,10.);
#9604=VECTOR('',#31370,10.);
#9605=VECTOR('',#31373,10.);
#9606=VECTOR('',#31376,10.);
#9607=VECTOR('',#31381,10.);
#9608=VECTOR('',#31384,10.);
#9609=VECTOR('',#31387,10.);
#9610=VECTOR('',#31390,10.);
#9611=VECTOR('',#31393,10.);
#9612=VECTOR('',#31396,10.);
#9613=VECTOR('',#31399,10.);
#9614=VECTOR('',#31402,10.);
#9615=VECTOR('',#31405,10.);
#9616=VECTOR('',#31408,10.);
#9617=VECTOR('',#31411,10.);
#9618=VECTOR('',#31414,10.);
#9619=VECTOR('',#31417,10.);
#9620=VECTOR('',#31420,10.);
#9621=VECTOR('',#31423,10.);
#9622=VECTOR('',#31428,10.);
#9623=VECTOR('',#31431,10.);
#9624=VECTOR('',#31434,10.);
#9625=VECTOR('',#31439,10.);
#9626=VECTOR('',#31442,10.);
#9627=VECTOR('',#31445,10.);
#9628=VECTOR('',#31448,10.);
#9629=VECTOR('',#31451,10.);
#9630=VECTOR('',#31454,10.);
#9631=VECTOR('',#31457,10.);
#9632=VECTOR('',#31460,10.);
#9633=VECTOR('',#31463,10.);
#9634=VECTOR('',#31466,10.);
#9635=VECTOR('',#31469,10.);
#9636=VECTOR('',#31472,10.);
#9637=VECTOR('',#31475,10.);
#9638=VECTOR('',#31478,10.);
#9639=VECTOR('',#31481,10.);
#9640=VECTOR('',#31486,10.);
#9641=VECTOR('',#31489,10.);
#9642=VECTOR('',#31492,10.);
#9643=VECTOR('',#31497,10.);
#9644=VECTOR('',#31500,10.);
#9645=VECTOR('',#31503,10.);
#9646=VECTOR('',#31506,10.);
#9647=VECTOR('',#31509,10.);
#9648=VECTOR('',#31512,10.);
#9649=VECTOR('',#31515,10.);
#9650=VECTOR('',#31518,10.);
#9651=VECTOR('',#31521,10.);
#9652=VECTOR('',#31524,10.);
#9653=VECTOR('',#31527,10.);
#9654=VECTOR('',#31530,10.);
#9655=VECTOR('',#31533,10.);
#9656=VECTOR('',#31536,10.);
#9657=VECTOR('',#31539,10.);
#9658=VECTOR('',#31544,10.);
#9659=VECTOR('',#31547,10.);
#9660=VECTOR('',#31550,10.);
#9661=VECTOR('',#31555,10.);
#9662=VECTOR('',#31558,10.);
#9663=VECTOR('',#31561,10.);
#9664=VECTOR('',#31564,10.);
#9665=VECTOR('',#31567,10.);
#9666=VECTOR('',#31570,10.);
#9667=VECTOR('',#31573,10.);
#9668=VECTOR('',#31576,10.);
#9669=VECTOR('',#31579,10.);
#9670=VECTOR('',#31582,10.);
#9671=VECTOR('',#31585,10.);
#9672=VECTOR('',#31588,10.);
#9673=VECTOR('',#31591,10.);
#9674=VECTOR('',#31594,10.);
#9675=VECTOR('',#31597,10.);
#9676=VECTOR('',#31602,10.);
#9677=VECTOR('',#31605,10.);
#9678=VECTOR('',#31608,10.);
#9679=VECTOR('',#31613,10.);
#9680=VECTOR('',#31616,10.);
#9681=VECTOR('',#31619,10.);
#9682=VECTOR('',#31622,10.);
#9683=VECTOR('',#31625,10.);
#9684=VECTOR('',#31628,10.);
#9685=VECTOR('',#31631,10.);
#9686=VECTOR('',#31634,10.);
#9687=VECTOR('',#31637,10.);
#9688=VECTOR('',#31640,10.);
#9689=VECTOR('',#31643,10.);
#9690=VECTOR('',#31646,10.);
#9691=VECTOR('',#31649,10.);
#9692=VECTOR('',#31652,10.);
#9693=VECTOR('',#31655,10.);
#9694=VECTOR('',#31660,10.);
#9695=VECTOR('',#31663,10.);
#9696=VECTOR('',#31666,10.);
#9697=VECTOR('',#31671,10.);
#9698=VECTOR('',#31674,10.);
#9699=VECTOR('',#31677,10.);
#9700=VECTOR('',#31680,10.);
#9701=VECTOR('',#31683,10.);
#9702=VECTOR('',#31686,10.);
#9703=VECTOR('',#31689,10.);
#9704=VECTOR('',#31692,10.);
#9705=VECTOR('',#31695,10.);
#9706=VECTOR('',#31698,10.);
#9707=VECTOR('',#31701,10.);
#9708=VECTOR('',#31704,10.);
#9709=VECTOR('',#31707,10.);
#9710=VECTOR('',#31710,10.);
#9711=VECTOR('',#31713,10.);
#9712=VECTOR('',#31718,10.);
#9713=VECTOR('',#31721,10.);
#9714=VECTOR('',#31724,10.);
#9715=VECTOR('',#31729,10.);
#9716=VECTOR('',#31732,10.);
#9717=VECTOR('',#31735,10.);
#9718=VECTOR('',#31738,10.);
#9719=VECTOR('',#31741,10.);
#9720=VECTOR('',#31744,10.);
#9721=VECTOR('',#31747,10.);
#9722=VECTOR('',#31750,10.);
#9723=VECTOR('',#31753,10.);
#9724=VECTOR('',#31756,10.);
#9725=VECTOR('',#31759,10.);
#9726=VECTOR('',#31762,10.);
#9727=VECTOR('',#31765,10.);
#9728=VECTOR('',#31768,10.);
#9729=VECTOR('',#31771,10.);
#9730=VECTOR('',#31776,10.);
#9731=VECTOR('',#31779,10.);
#9732=VECTOR('',#31782,10.);
#9733=VECTOR('',#31787,10.);
#9734=VECTOR('',#31790,10.);
#9735=VECTOR('',#31793,10.);
#9736=VECTOR('',#31796,10.);
#9737=VECTOR('',#31799,10.);
#9738=VECTOR('',#31802,10.);
#9739=VECTOR('',#31805,10.);
#9740=VECTOR('',#31808,10.);
#9741=VECTOR('',#31811,10.);
#9742=VECTOR('',#31814,10.);
#9743=VECTOR('',#31817,10.);
#9744=VECTOR('',#31820,10.);
#9745=VECTOR('',#31823,10.);
#9746=VECTOR('',#31826,10.);
#9747=VECTOR('',#31829,10.);
#9748=VECTOR('',#31834,10.);
#9749=VECTOR('',#31837,10.);
#9750=VECTOR('',#31840,10.);
#9751=VECTOR('',#31845,10.);
#9752=VECTOR('',#31848,10.);
#9753=VECTOR('',#31851,10.);
#9754=VECTOR('',#31854,10.);
#9755=VECTOR('',#31857,10.);
#9756=VECTOR('',#31860,10.);
#9757=VECTOR('',#31863,10.);
#9758=VECTOR('',#31866,10.);
#9759=VECTOR('',#31869,10.);
#9760=VECTOR('',#31872,10.);
#9761=VECTOR('',#31875,10.);
#9762=VECTOR('',#31878,10.);
#9763=VECTOR('',#31881,10.);
#9764=VECTOR('',#31884,10.);
#9765=VECTOR('',#31887,10.);
#9766=VECTOR('',#31894,8.5);
#9767=VECTOR('',#31903,8.5);
#10577=CIRCLE('',#26066,8.5);
#10578=CIRCLE('',#26140,8.5);
#10579=CIRCLE('',#26405,8.5);
#10580=CIRCLE('',#26408,8.5);
#11844=VERTEX_POINT('',#38098);
#11845=VERTEX_POINT('',#38099);
#11846=VERTEX_POINT('',#38101);
#11847=VERTEX_POINT('',#38103);
#11848=VERTEX_POINT('',#38105);
#11849=VERTEX_POINT('',#38107);
#11850=VERTEX_POINT('',#38111);
#11851=VERTEX_POINT('',#38113);
#11852=VERTEX_POINT('',#38115);
#11853=VERTEX_POINT('',#38117);
#11854=VERTEX_POINT('',#38119);
#11855=VERTEX_POINT('',#38121);
#11856=VERTEX_POINT('',#38123);
#11857=VERTEX_POINT('',#38125);
#11858=VERTEX_POINT('',#38127);
#11859=VERTEX_POINT('',#38129);
#11860=VERTEX_POINT('',#38131);
#11861=VERTEX_POINT('',#38133);
#11862=VERTEX_POINT('',#38135);
#11863=VERTEX_POINT('',#38137);
#11864=VERTEX_POINT('',#38139);
#11865=VERTEX_POINT('',#38141);
#11866=VERTEX_POINT('',#38143);
#11867=VERTEX_POINT('',#38145);
#11868=VERTEX_POINT('',#38147);
#11869=VERTEX_POINT('',#38149);
#11870=VERTEX_POINT('',#38151);
#11871=VERTEX_POINT('',#38153);
#11872=VERTEX_POINT('',#38155);
#11873=VERTEX_POINT('',#38157);
#11874=VERTEX_POINT('',#38159);
#11875=VERTEX_POINT('',#38161);
#11876=VERTEX_POINT('',#38163);
#11877=VERTEX_POINT('',#38165);
#11878=VERTEX_POINT('',#38167);
#11879=VERTEX_POINT('',#38169);
#11880=VERTEX_POINT('',#38171);
#11881=VERTEX_POINT('',#38173);
#11882=VERTEX_POINT('',#38175);
#11883=VERTEX_POINT('',#38177);
#11884=VERTEX_POINT('',#38179);
#11885=VERTEX_POINT('',#38181);
#11886=VERTEX_POINT('',#38183);
#11887=VERTEX_POINT('',#38185);
#11888=VERTEX_POINT('',#38187);
#11889=VERTEX_POINT('',#38189);
#11890=VERTEX_POINT('',#38191);
#11891=VERTEX_POINT('',#38193);
#11892=VERTEX_POINT('',#38195);
#11893=VERTEX_POINT('',#38197);
#11894=VERTEX_POINT('',#38199);
#11895=VERTEX_POINT('',#38201);
#11896=VERTEX_POINT('',#38203);
#11897=VERTEX_POINT('',#38205);
#11898=VERTEX_POINT('',#38207);
#11899=VERTEX_POINT('',#38209);
#11900=VERTEX_POINT('',#38211);
#11901=VERTEX_POINT('',#38213);
#11902=VERTEX_POINT('',#38215);
#11903=VERTEX_POINT('',#38217);
#11904=VERTEX_POINT('',#38219);
#11905=VERTEX_POINT('',#38221);
#11906=VERTEX_POINT('',#38223);
#11907=VERTEX_POINT('',#38225);
#11908=VERTEX_POINT('',#38227);
#11909=VERTEX_POINT('',#38229);
#11910=VERTEX_POINT('',#38231);
#11911=VERTEX_POINT('',#38233);
#11912=VERTEX_POINT('',#38235);
#11913=VERTEX_POINT('',#38237);
#11914=VERTEX_POINT('',#38239);
#11915=VERTEX_POINT('',#38241);
#11916=VERTEX_POINT('',#38243);
#11917=VERTEX_POINT('',#38245);
#11918=VERTEX_POINT('',#38247);
#11919=VERTEX_POINT('',#38249);
#11920=VERTEX_POINT('',#38251);
#11921=VERTEX_POINT('',#38253);
#11922=VERTEX_POINT('',#38255);
#11923=VERTEX_POINT('',#38257);
#11924=VERTEX_POINT('',#38259);
#11925=VERTEX_POINT('',#38261);
#11926=VERTEX_POINT('',#38263);
#11927=VERTEX_POINT('',#38265);
#11928=VERTEX_POINT('',#38267);
#11929=VERTEX_POINT('',#38269);
#11930=VERTEX_POINT('',#38271);
#11931=VERTEX_POINT('',#38273);
#11932=VERTEX_POINT('',#38275);
#11933=VERTEX_POINT('',#38277);
#11934=VERTEX_POINT('',#38279);
#11935=VERTEX_POINT('',#38281);
#11936=VERTEX_POINT('',#38283);
#11937=VERTEX_POINT('',#38285);
#11938=VERTEX_POINT('',#38287);
#11939=VERTEX_POINT('',#38289);
#11940=VERTEX_POINT('',#38291);
#11941=VERTEX_POINT('',#38293);
#11942=VERTEX_POINT('',#38295);
#11943=VERTEX_POINT('',#38297);
#11944=VERTEX_POINT('',#38299);
#11945=VERTEX_POINT('',#38301);
#11946=VERTEX_POINT('',#38303);
#11947=VERTEX_POINT('',#38305);
#11948=VERTEX_POINT('',#38307);
#11949=VERTEX_POINT('',#38309);
#11950=VERTEX_POINT('',#38311);
#11951=VERTEX_POINT('',#38313);
#11952=VERTEX_POINT('',#38315);
#11953=VERTEX_POINT('',#38317);
#11954=VERTEX_POINT('',#38319);
#11955=VERTEX_POINT('',#38321);
#11956=VERTEX_POINT('',#38323);
#11957=VERTEX_POINT('',#38325);
#11958=VERTEX_POINT('',#38327);
#11959=VERTEX_POINT('',#38329);
#11960=VERTEX_POINT('',#38331);
#11961=VERTEX_POINT('',#38333);
#11962=VERTEX_POINT('',#38335);
#11963=VERTEX_POINT('',#38337);
#11964=VERTEX_POINT('',#38339);
#11965=VERTEX_POINT('',#38341);
#11966=VERTEX_POINT('',#38343);
#11967=VERTEX_POINT('',#38345);
#11968=VERTEX_POINT('',#38347);
#11969=VERTEX_POINT('',#38349);
#11970=VERTEX_POINT('',#38351);
#11971=VERTEX_POINT('',#38353);
#11972=VERTEX_POINT('',#38355);
#11973=VERTEX_POINT('',#38357);
#11974=VERTEX_POINT('',#38359);
#11975=VERTEX_POINT('',#38361);
#11976=VERTEX_POINT('',#38363);
#11977=VERTEX_POINT('',#38365);
#11978=VERTEX_POINT('',#38367);
#11979=VERTEX_POINT('',#38369);
#11980=VERTEX_POINT('',#38371);
#11981=VERTEX_POINT('',#38373);
#11982=VERTEX_POINT('',#38375);
#11983=VERTEX_POINT('',#38377);
#11984=VERTEX_POINT('',#38379);
#11985=VERTEX_POINT('',#38381);
#11986=VERTEX_POINT('',#38383);
#11987=VERTEX_POINT('',#38385);
#11988=VERTEX_POINT('',#38387);
#11989=VERTEX_POINT('',#38389);
#11990=VERTEX_POINT('',#38391);
#11991=VERTEX_POINT('',#38393);
#11992=VERTEX_POINT('',#38395);
#11993=VERTEX_POINT('',#38397);
#11994=VERTEX_POINT('',#38399);
#11995=VERTEX_POINT('',#38401);
#11996=VERTEX_POINT('',#38403);
#11997=VERTEX_POINT('',#38405);
#11998=VERTEX_POINT('',#38407);
#11999=VERTEX_POINT('',#38409);
#12000=VERTEX_POINT('',#38411);
#12001=VERTEX_POINT('',#38413);
#12002=VERTEX_POINT('',#38415);
#12003=VERTEX_POINT('',#38417);
#12004=VERTEX_POINT('',#38419);
#12005=VERTEX_POINT('',#38421);
#12006=VERTEX_POINT('',#38423);
#12007=VERTEX_POINT('',#38425);
#12008=VERTEX_POINT('',#38427);
#12009=VERTEX_POINT('',#38429);
#12010=VERTEX_POINT('',#38431);
#12011=VERTEX_POINT('',#38433);
#12012=VERTEX_POINT('',#38435);
#12013=VERTEX_POINT('',#38437);
#12014=VERTEX_POINT('',#38439);
#12015=VERTEX_POINT('',#38441);
#12016=VERTEX_POINT('',#38443);
#12017=VERTEX_POINT('',#38445);
#12018=VERTEX_POINT('',#38447);
#12019=VERTEX_POINT('',#38449);
#12020=VERTEX_POINT('',#38451);
#12021=VERTEX_POINT('',#38453);
#12022=VERTEX_POINT('',#38455);
#12023=VERTEX_POINT('',#38457);
#12024=VERTEX_POINT('',#38459);
#12025=VERTEX_POINT('',#38461);
#12026=VERTEX_POINT('',#38463);
#12027=VERTEX_POINT('',#38465);
#12028=VERTEX_POINT('',#38467);
#12029=VERTEX_POINT('',#38469);
#12030=VERTEX_POINT('',#38471);
#12031=VERTEX_POINT('',#38473);
#12032=VERTEX_POINT('',#38475);
#12033=VERTEX_POINT('',#38477);
#12034=VERTEX_POINT('',#38479);
#12035=VERTEX_POINT('',#38481);
#12036=VERTEX_POINT('',#38483);
#12037=VERTEX_POINT('',#38485);
#12038=VERTEX_POINT('',#38487);
#12039=VERTEX_POINT('',#38489);
#12040=VERTEX_POINT('',#38491);
#12041=VERTEX_POINT('',#38493);
#12042=VERTEX_POINT('',#38495);
#12043=VERTEX_POINT('',#38497);
#12044=VERTEX_POINT('',#38499);
#12045=VERTEX_POINT('',#38501);
#12046=VERTEX_POINT('',#38503);
#12047=VERTEX_POINT('',#38505);
#12048=VERTEX_POINT('',#38507);
#12049=VERTEX_POINT('',#38509);
#12050=VERTEX_POINT('',#38511);
#12051=VERTEX_POINT('',#38513);
#12052=VERTEX_POINT('',#38515);
#12053=VERTEX_POINT('',#38517);
#12054=VERTEX_POINT('',#38519);
#12055=VERTEX_POINT('',#38521);
#12056=VERTEX_POINT('',#38523);
#12057=VERTEX_POINT('',#38525);
#12058=VERTEX_POINT('',#38527);
#12059=VERTEX_POINT('',#38529);
#12060=VERTEX_POINT('',#38531);
#12061=VERTEX_POINT('',#38533);
#12062=VERTEX_POINT('',#38535);
#12063=VERTEX_POINT('',#38537);
#12064=VERTEX_POINT('',#38539);
#12065=VERTEX_POINT('',#38541);
#12066=VERTEX_POINT('',#38543);
#12067=VERTEX_POINT('',#38545);
#12068=VERTEX_POINT('',#38547);
#12069=VERTEX_POINT('',#38549);
#12070=VERTEX_POINT('',#38551);
#12071=VERTEX_POINT('',#38553);
#12072=VERTEX_POINT('',#38555);
#12073=VERTEX_POINT('',#38557);
#12074=VERTEX_POINT('',#38559);
#12075=VERTEX_POINT('',#38561);
#12076=VERTEX_POINT('',#38563);
#12077=VERTEX_POINT('',#38565);
#12078=VERTEX_POINT('',#38567);
#12079=VERTEX_POINT('',#38569);
#12080=VERTEX_POINT('',#38571);
#12081=VERTEX_POINT('',#38573);
#12082=VERTEX_POINT('',#38575);
#12083=VERTEX_POINT('',#38577);
#12084=VERTEX_POINT('',#38579);
#12085=VERTEX_POINT('',#38581);
#12086=VERTEX_POINT('',#38583);
#12087=VERTEX_POINT('',#38585);
#12088=VERTEX_POINT('',#38588);
#12089=VERTEX_POINT('',#38591);
#12090=VERTEX_POINT('',#38593);
#12091=VERTEX_POINT('',#38595);
#12092=VERTEX_POINT('',#38599);
#12093=VERTEX_POINT('',#38603);
#12094=VERTEX_POINT('',#38605);
#12095=VERTEX_POINT('',#38607);
#12096=VERTEX_POINT('',#38609);
#12097=VERTEX_POINT('',#38613);
#12098=VERTEX_POINT('',#38615);
#12099=VERTEX_POINT('',#38617);
#12100=VERTEX_POINT('',#38621);
#12101=VERTEX_POINT('',#38625);
#12102=VERTEX_POINT('',#38627);
#12103=VERTEX_POINT('',#38629);
#12104=VERTEX_POINT('',#38631);
#12105=VERTEX_POINT('',#38635);
#12106=VERTEX_POINT('',#38637);
#12107=VERTEX_POINT('',#38639);
#12108=VERTEX_POINT('',#38643);
#12109=VERTEX_POINT('',#38647);
#12110=VERTEX_POINT('',#38649);
#12111=VERTEX_POINT('',#38651);
#12112=VERTEX_POINT('',#38653);
#12113=VERTEX_POINT('',#38657);
#12114=VERTEX_POINT('',#38659);
#12115=VERTEX_POINT('',#38661);
#12116=VERTEX_POINT('',#38665);
#12117=VERTEX_POINT('',#38669);
#12118=VERTEX_POINT('',#38671);
#12119=VERTEX_POINT('',#38673);
#12120=VERTEX_POINT('',#38675);
#12121=VERTEX_POINT('',#38679);
#12122=VERTEX_POINT('',#38681);
#12123=VERTEX_POINT('',#38683);
#12124=VERTEX_POINT('',#38687);
#12125=VERTEX_POINT('',#38691);
#12126=VERTEX_POINT('',#38693);
#12127=VERTEX_POINT('',#38695);
#12128=VERTEX_POINT('',#38697);
#12129=VERTEX_POINT('',#38701);
#12130=VERTEX_POINT('',#38703);
#12131=VERTEX_POINT('',#38705);
#12132=VERTEX_POINT('',#38709);
#12133=VERTEX_POINT('',#38713);
#12134=VERTEX_POINT('',#38715);
#12135=VERTEX_POINT('',#38717);
#12136=VERTEX_POINT('',#38719);
#12137=VERTEX_POINT('',#38723);
#12138=VERTEX_POINT('',#38725);
#12139=VERTEX_POINT('',#38727);
#12140=VERTEX_POINT('',#38731);
#12141=VERTEX_POINT('',#38735);
#12142=VERTEX_POINT('',#38737);
#12143=VERTEX_POINT('',#38739);
#12144=VERTEX_POINT('',#38741);
#12145=VERTEX_POINT('',#38745);
#12146=VERTEX_POINT('',#38747);
#12147=VERTEX_POINT('',#38749);
#12148=VERTEX_POINT('',#38753);
#12149=VERTEX_POINT('',#38757);
#12150=VERTEX_POINT('',#38759);
#12151=VERTEX_POINT('',#38761);
#12152=VERTEX_POINT('',#38763);
#12153=VERTEX_POINT('',#38767);
#12154=VERTEX_POINT('',#38769);
#12155=VERTEX_POINT('',#38771);
#12156=VERTEX_POINT('',#38775);
#12157=VERTEX_POINT('',#38779);
#12158=VERTEX_POINT('',#38781);
#12159=VERTEX_POINT('',#38783);
#12160=VERTEX_POINT('',#38785);
#12161=VERTEX_POINT('',#38789);
#12162=VERTEX_POINT('',#38791);
#12163=VERTEX_POINT('',#38793);
#12164=VERTEX_POINT('',#38797);
#12165=VERTEX_POINT('',#38801);
#12166=VERTEX_POINT('',#38803);
#12167=VERTEX_POINT('',#38805);
#12168=VERTEX_POINT('',#38807);
#12169=VERTEX_POINT('',#38811);
#12170=VERTEX_POINT('',#38813);
#12171=VERTEX_POINT('',#38815);
#12172=VERTEX_POINT('',#38819);
#12173=VERTEX_POINT('',#38823);
#12174=VERTEX_POINT('',#38825);
#12175=VERTEX_POINT('',#38827);
#12176=VERTEX_POINT('',#38829);
#12177=VERTEX_POINT('',#38833);
#12178=VERTEX_POINT('',#38835);
#12179=VERTEX_POINT('',#38837);
#12180=VERTEX_POINT('',#38841);
#12181=VERTEX_POINT('',#38845);
#12182=VERTEX_POINT('',#38846);
#12183=VERTEX_POINT('',#38848);
#12184=VERTEX_POINT('',#38851);
#12185=VERTEX_POINT('',#38855);
#12186=VERTEX_POINT('',#38857);
#12187=VERTEX_POINT('',#38861);
#12188=VERTEX_POINT('',#38865);
#12189=VERTEX_POINT('',#38866);
#12190=VERTEX_POINT('',#38868);
#12191=VERTEX_POINT('',#38871);
#12192=VERTEX_POINT('',#38875);
#12193=VERTEX_POINT('',#38877);
#12194=VERTEX_POINT('',#38881);
#12195=VERTEX_POINT('',#38885);
#12196=VERTEX_POINT('',#38886);
#12197=VERTEX_POINT('',#38888);
#12198=VERTEX_POINT('',#38891);
#12199=VERTEX_POINT('',#38895);
#12200=VERTEX_POINT('',#38897);
#12201=VERTEX_POINT('',#38901);
#12202=VERTEX_POINT('',#38905);
#12203=VERTEX_POINT('',#38906);
#12204=VERTEX_POINT('',#38908);
#12205=VERTEX_POINT('',#38911);
#12206=VERTEX_POINT('',#38915);
#12207=VERTEX_POINT('',#38917);
#12208=VERTEX_POINT('',#38921);
#12209=VERTEX_POINT('',#38925);
#12210=VERTEX_POINT('',#38926);
#12211=VERTEX_POINT('',#38928);
#12212=VERTEX_POINT('',#38931);
#12213=VERTEX_POINT('',#38935);
#12214=VERTEX_POINT('',#38937);
#12215=VERTEX_POINT('',#38941);
#12216=VERTEX_POINT('',#38945);
#12217=VERTEX_POINT('',#38946);
#12218=VERTEX_POINT('',#38948);
#12219=VERTEX_POINT('',#38951);
#12220=VERTEX_POINT('',#38955);
#12221=VERTEX_POINT('',#38957);
#12222=VERTEX_POINT('',#38961);
#12223=VERTEX_POINT('',#38965);
#12224=VERTEX_POINT('',#38966);
#12225=VERTEX_POINT('',#38968);
#12226=VERTEX_POINT('',#38971);
#12227=VERTEX_POINT('',#38975);
#12228=VERTEX_POINT('',#38977);
#12229=VERTEX_POINT('',#38981);
#12230=VERTEX_POINT('',#38985);
#12231=VERTEX_POINT('',#38986);
#12232=VERTEX_POINT('',#38988);
#12233=VERTEX_POINT('',#38991);
#12234=VERTEX_POINT('',#38995);
#12235=VERTEX_POINT('',#38997);
#12236=VERTEX_POINT('',#39001);
#12237=VERTEX_POINT('',#39005);
#12238=VERTEX_POINT('',#39006);
#12239=VERTEX_POINT('',#39008);
#12240=VERTEX_POINT('',#39011);
#12241=VERTEX_POINT('',#39015);
#12242=VERTEX_POINT('',#39017);
#12243=VERTEX_POINT('',#39021);
#12244=VERTEX_POINT('',#39025);
#12245=VERTEX_POINT('',#39026);
#12246=VERTEX_POINT('',#39028);
#12247=VERTEX_POINT('',#39031);
#12248=VERTEX_POINT('',#39035);
#12249=VERTEX_POINT('',#39037);
#12250=VERTEX_POINT('',#39041);
#12251=VERTEX_POINT('',#39045);
#12252=VERTEX_POINT('',#39046);
#12253=VERTEX_POINT('',#39048);
#12254=VERTEX_POINT('',#39051);
#12255=VERTEX_POINT('',#39055);
#12256=VERTEX_POINT('',#39057);
#12257=VERTEX_POINT('',#39061);
#12258=VERTEX_POINT('',#39065);
#12259=VERTEX_POINT('',#39066);
#12260=VERTEX_POINT('',#39068);
#12261=VERTEX_POINT('',#39071);
#12262=VERTEX_POINT('',#39075);
#12263=VERTEX_POINT('',#39077);
#12264=VERTEX_POINT('',#39081);
#12265=VERTEX_POINT('',#39085);
#12266=VERTEX_POINT('',#39087);
#12267=VERTEX_POINT('',#39089);
#12268=VERTEX_POINT('',#39093);
#12269=VERTEX_POINT('',#39095);
#12270=VERTEX_POINT('',#39097);
#12271=VERTEX_POINT('',#39099);
#12272=VERTEX_POINT('',#39101);
#12273=VERTEX_POINT('',#39103);
#12274=VERTEX_POINT('',#39105);
#12275=VERTEX_POINT('',#39107);
#12276=VERTEX_POINT('',#39109);
#12277=VERTEX_POINT('',#39111);
#12278=VERTEX_POINT('',#39113);
#12279=VERTEX_POINT('',#39115);
#12280=VERTEX_POINT('',#39117);
#12281=VERTEX_POINT('',#39119);
#12282=VERTEX_POINT('',#39121);
#12283=VERTEX_POINT('',#39123);
#12284=VERTEX_POINT('',#39125);
#12285=VERTEX_POINT('',#39128);
#12286=VERTEX_POINT('',#39130);
#12287=VERTEX_POINT('',#39132);
#12288=VERTEX_POINT('',#39134);
#12289=VERTEX_POINT('',#39136);
#12290=VERTEX_POINT('',#39138);
#12291=VERTEX_POINT('',#39140);
#12292=VERTEX_POINT('',#39142);
#12293=VERTEX_POINT('',#39144);
#12294=VERTEX_POINT('',#39146);
#12295=VERTEX_POINT('',#39148);
#12296=VERTEX_POINT('',#39150);
#12297=VERTEX_POINT('',#39152);
#12298=VERTEX_POINT('',#39154);
#12299=VERTEX_POINT('',#39156);
#12300=VERTEX_POINT('',#39158);
#12301=VERTEX_POINT('',#39160);
#12302=VERTEX_POINT('',#39162);
#12303=VERTEX_POINT('',#39165);
#12304=VERTEX_POINT('',#39167);
#12305=VERTEX_POINT('',#39169);
#12306=VERTEX_POINT('',#39171);
#12307=VERTEX_POINT('',#39173);
#12308=VERTEX_POINT('',#39175);
#12309=VERTEX_POINT('',#39177);
#12310=VERTEX_POINT('',#39179);
#12311=VERTEX_POINT('',#39181);
#12312=VERTEX_POINT('',#39183);
#12313=VERTEX_POINT('',#39185);
#12314=VERTEX_POINT('',#39187);
#12315=VERTEX_POINT('',#39189);
#12316=VERTEX_POINT('',#39191);
#12317=VERTEX_POINT('',#39193);
#12318=VERTEX_POINT('',#39195);
#12319=VERTEX_POINT('',#39197);
#12320=VERTEX_POINT('',#39199);
#12321=VERTEX_POINT('',#39202);
#12322=VERTEX_POINT('',#39204);
#12323=VERTEX_POINT('',#39206);
#12324=VERTEX_POINT('',#39208);
#12325=VERTEX_POINT('',#39210);
#12326=VERTEX_POINT('',#39212);
#12327=VERTEX_POINT('',#39214);
#12328=VERTEX_POINT('',#39216);
#12329=VERTEX_POINT('',#39218);
#12330=VERTEX_POINT('',#39220);
#12331=VERTEX_POINT('',#39222);
#12332=VERTEX_POINT('',#39224);
#12333=VERTEX_POINT('',#39226);
#12334=VERTEX_POINT('',#39228);
#12335=VERTEX_POINT('',#39230);
#12336=VERTEX_POINT('',#39232);
#12337=VERTEX_POINT('',#39234);
#12338=VERTEX_POINT('',#39236);
#12339=VERTEX_POINT('',#39239);
#12340=VERTEX_POINT('',#39241);
#12341=VERTEX_POINT('',#39243);
#12342=VERTEX_POINT('',#39245);
#12343=VERTEX_POINT('',#39247);
#12344=VERTEX_POINT('',#39249);
#12345=VERTEX_POINT('',#39251);
#12346=VERTEX_POINT('',#39253);
#12347=VERTEX_POINT('',#39255);
#12348=VERTEX_POINT('',#39257);
#12349=VERTEX_POINT('',#39259);
#12350=VERTEX_POINT('',#39261);
#12351=VERTEX_POINT('',#39263);
#12352=VERTEX_POINT('',#39265);
#12353=VERTEX_POINT('',#39267);
#12354=VERTEX_POINT('',#39269);
#12355=VERTEX_POINT('',#39271);
#12356=VERTEX_POINT('',#39273);
#12357=VERTEX_POINT('',#39276);
#12358=VERTEX_POINT('',#39278);
#12359=VERTEX_POINT('',#39280);
#12360=VERTEX_POINT('',#39282);
#12361=VERTEX_POINT('',#39284);
#12362=VERTEX_POINT('',#39286);
#12363=VERTEX_POINT('',#39288);
#12364=VERTEX_POINT('',#39290);
#12365=VERTEX_POINT('',#39292);
#12366=VERTEX_POINT('',#39294);
#12367=VERTEX_POINT('',#39296);
#12368=VERTEX_POINT('',#39298);
#12369=VERTEX_POINT('',#39300);
#12370=VERTEX_POINT('',#39302);
#12371=VERTEX_POINT('',#39304);
#12372=VERTEX_POINT('',#39306);
#12373=VERTEX_POINT('',#39308);
#12374=VERTEX_POINT('',#39310);
#12375=VERTEX_POINT('',#39313);
#12376=VERTEX_POINT('',#39315);
#12377=VERTEX_POINT('',#39317);
#12378=VERTEX_POINT('',#39319);
#12379=VERTEX_POINT('',#39321);
#12380=VERTEX_POINT('',#39323);
#12381=VERTEX_POINT('',#39325);
#12382=VERTEX_POINT('',#39327);
#12383=VERTEX_POINT('',#39329);
#12384=VERTEX_POINT('',#39331);
#12385=VERTEX_POINT('',#39333);
#12386=VERTEX_POINT('',#39335);
#12387=VERTEX_POINT('',#39337);
#12388=VERTEX_POINT('',#39339);
#12389=VERTEX_POINT('',#39341);
#12390=VERTEX_POINT('',#39343);
#12391=VERTEX_POINT('',#39345);
#12392=VERTEX_POINT('',#39347);
#12393=VERTEX_POINT('',#39350);
#12394=VERTEX_POINT('',#39352);
#12395=VERTEX_POINT('',#39354);
#12396=VERTEX_POINT('',#39356);
#12397=VERTEX_POINT('',#39358);
#12398=VERTEX_POINT('',#39360);
#12399=VERTEX_POINT('',#39362);
#12400=VERTEX_POINT('',#39364);
#12401=VERTEX_POINT('',#39366);
#12402=VERTEX_POINT('',#39368);
#12403=VERTEX_POINT('',#39370);
#12404=VERTEX_POINT('',#39372);
#12405=VERTEX_POINT('',#39374);
#12406=VERTEX_POINT('',#39376);
#12407=VERTEX_POINT('',#39378);
#12408=VERTEX_POINT('',#39380);
#12409=VERTEX_POINT('',#39382);
#12410=VERTEX_POINT('',#39384);
#12411=VERTEX_POINT('',#39387);
#12412=VERTEX_POINT('',#39389);
#12413=VERTEX_POINT('',#39391);
#12414=VERTEX_POINT('',#39393);
#12415=VERTEX_POINT('',#39395);
#12416=VERTEX_POINT('',#39397);
#12417=VERTEX_POINT('',#39399);
#12418=VERTEX_POINT('',#39401);
#12419=VERTEX_POINT('',#39403);
#12420=VERTEX_POINT('',#39405);
#12421=VERTEX_POINT('',#39407);
#12422=VERTEX_POINT('',#39409);
#12423=VERTEX_POINT('',#39411);
#12424=VERTEX_POINT('',#39413);
#12425=VERTEX_POINT('',#39415);
#12426=VERTEX_POINT('',#39417);
#12427=VERTEX_POINT('',#39419);
#12428=VERTEX_POINT('',#39421);
#12429=VERTEX_POINT('',#39424);
#12430=VERTEX_POINT('',#39426);
#12431=VERTEX_POINT('',#39428);
#12432=VERTEX_POINT('',#39430);
#12433=VERTEX_POINT('',#39432);
#12434=VERTEX_POINT('',#39434);
#12435=VERTEX_POINT('',#39436);
#12436=VERTEX_POINT('',#39438);
#12437=VERTEX_POINT('',#39440);
#12438=VERTEX_POINT('',#39442);
#12439=VERTEX_POINT('',#39444);
#12440=VERTEX_POINT('',#39446);
#12441=VERTEX_POINT('',#39448);
#12442=VERTEX_POINT('',#39450);
#12443=VERTEX_POINT('',#39452);
#12444=VERTEX_POINT('',#39454);
#12445=VERTEX_POINT('',#39456);
#12446=VERTEX_POINT('',#39458);
#12447=VERTEX_POINT('',#39461);
#12448=VERTEX_POINT('',#39463);
#12449=VERTEX_POINT('',#39465);
#12450=VERTEX_POINT('',#39467);
#12451=VERTEX_POINT('',#39469);
#12452=VERTEX_POINT('',#39471);
#12453=VERTEX_POINT('',#39473);
#12454=VERTEX_POINT('',#39475);
#12455=VERTEX_POINT('',#39477);
#12456=VERTEX_POINT('',#39479);
#12457=VERTEX_POINT('',#39481);
#12458=VERTEX_POINT('',#39483);
#12459=VERTEX_POINT('',#39485);
#12460=VERTEX_POINT('',#39487);
#12461=VERTEX_POINT('',#39489);
#12462=VERTEX_POINT('',#39491);
#12463=VERTEX_POINT('',#39493);
#12464=VERTEX_POINT('',#39495);
#12465=VERTEX_POINT('',#39498);
#12466=VERTEX_POINT('',#39500);
#12467=VERTEX_POINT('',#39502);
#12468=VERTEX_POINT('',#39504);
#12469=VERTEX_POINT('',#39506);
#12470=VERTEX_POINT('',#39508);
#12471=VERTEX_POINT('',#39510);
#12472=VERTEX_POINT('',#39512);
#12473=VERTEX_POINT('',#39514);
#12474=VERTEX_POINT('',#39516);
#12475=VERTEX_POINT('',#39518);
#12476=VERTEX_POINT('',#39520);
#12477=VERTEX_POINT('',#39522);
#12478=VERTEX_POINT('',#39524);
#12479=VERTEX_POINT('',#39526);
#12480=VERTEX_POINT('',#39528);
#12481=VERTEX_POINT('',#39530);
#12482=VERTEX_POINT('',#39532);
#12483=VERTEX_POINT('',#39535);
#12484=VERTEX_POINT('',#39538);
#12485=VERTEX_POINT('',#39543);
#12486=VERTEX_POINT('',#39545);
#12487=VERTEX_POINT('',#39549);
#12488=VERTEX_POINT('',#39554);
#12489=VERTEX_POINT('',#39556);
#12490=VERTEX_POINT('',#39560);
#12491=VERTEX_POINT('',#39565);
#12492=VERTEX_POINT('',#39567);
#12493=VERTEX_POINT('',#39571);
#12494=VERTEX_POINT('',#39576);
#12495=VERTEX_POINT('',#39578);
#12496=VERTEX_POINT('',#39582);
#12497=VERTEX_POINT('',#39587);
#12498=VERTEX_POINT('',#39589);
#12499=VERTEX_POINT('',#39593);
#12500=VERTEX_POINT('',#39598);
#12501=VERTEX_POINT('',#39600);
#12502=VERTEX_POINT('',#39604);
#12503=VERTEX_POINT('',#39609);
#12504=VERTEX_POINT('',#39611);
#12505=VERTEX_POINT('',#39615);
#12506=VERTEX_POINT('',#39620);
#12507=VERTEX_POINT('',#39622);
#12508=VERTEX_POINT('',#39626);
#12509=VERTEX_POINT('',#39631);
#12510=VERTEX_POINT('',#39633);
#12511=VERTEX_POINT('',#39637);
#12512=VERTEX_POINT('',#39642);
#12513=VERTEX_POINT('',#39644);
#12514=VERTEX_POINT('',#39648);
#12515=VERTEX_POINT('',#39653);
#12516=VERTEX_POINT('',#39655);
#12517=VERTEX_POINT('',#39659);
#12518=VERTEX_POINT('',#40120);
#12519=VERTEX_POINT('',#40125);
#14747=EDGE_CURVE('',#11844,#11845,#5889,.T.);
#14748=EDGE_CURVE('',#11845,#11846,#5890,.T.);
#14749=EDGE_CURVE('',#11846,#11847,#5891,.F.);
#14750=EDGE_CURVE('',#11847,#11848,#5892,.T.);
#14751=EDGE_CURVE('',#11848,#11849,#5893,.T.);
#14752=EDGE_CURVE('',#11849,#11844,#5894,.T.);
#14753=EDGE_CURVE('',#11850,#11846,#5895,.T.);
#14754=EDGE_CURVE('',#11845,#11851,#5896,.T.);
#14755=EDGE_CURVE('',#11851,#11852,#5897,.T.);
#14756=EDGE_CURVE('',#11852,#11853,#5898,.T.);
#14757=EDGE_CURVE('',#11853,#11854,#5899,.T.);
#14758=EDGE_CURVE('',#11854,#11855,#5900,.T.);
#14759=EDGE_CURVE('',#11855,#11856,#5901,.T.);
#14760=EDGE_CURVE('',#11856,#11857,#5902,.T.);
#14761=EDGE_CURVE('',#11857,#11858,#5903,.T.);
#14762=EDGE_CURVE('',#11858,#11859,#5904,.T.);
#14763=EDGE_CURVE('',#11859,#11860,#5905,.T.);
#14764=EDGE_CURVE('',#11860,#11861,#5906,.T.);
#14765=EDGE_CURVE('',#11861,#11862,#5907,.T.);
#14766=EDGE_CURVE('',#11862,#11863,#5908,.T.);
#14767=EDGE_CURVE('',#11863,#11864,#5909,.T.);
#14768=EDGE_CURVE('',#11864,#11865,#5910,.T.);
#14769=EDGE_CURVE('',#11865,#11866,#5911,.T.);
#14770=EDGE_CURVE('',#11867,#11866,#5912,.T.);
#14771=EDGE_CURVE('',#11867,#11868,#5913,.T.);
#14772=EDGE_CURVE('',#11868,#11869,#5914,.T.);
#14773=EDGE_CURVE('',#11870,#11869,#5915,.T.);
#14774=EDGE_CURVE('',#11870,#11871,#5916,.T.);
#14775=EDGE_CURVE('',#11871,#11872,#5917,.T.);
#14776=EDGE_CURVE('',#11872,#11873,#5918,.T.);
#14777=EDGE_CURVE('',#11873,#11874,#5919,.T.);
#14778=EDGE_CURVE('',#11874,#11875,#5920,.T.);
#14779=EDGE_CURVE('',#11875,#11876,#5921,.T.);
#14780=EDGE_CURVE('',#11876,#11877,#5922,.T.);
#14781=EDGE_CURVE('',#11877,#11878,#5923,.T.);
#14782=EDGE_CURVE('',#11878,#11879,#5924,.T.);
#14783=EDGE_CURVE('',#11879,#11880,#5925,.T.);
#14784=EDGE_CURVE('',#11880,#11881,#5926,.T.);
#14785=EDGE_CURVE('',#11881,#11882,#5927,.T.);
#14786=EDGE_CURVE('',#11882,#11883,#5928,.T.);
#14787=EDGE_CURVE('',#11883,#11884,#5929,.T.);
#14788=EDGE_CURVE('',#11884,#11885,#5930,.T.);
#14789=EDGE_CURVE('',#11885,#11886,#5931,.T.);
#14790=EDGE_CURVE('',#11887,#11886,#5932,.T.);
#14791=EDGE_CURVE('',#11887,#11888,#5933,.T.);
#14792=EDGE_CURVE('',#11888,#11889,#5934,.T.);
#14793=EDGE_CURVE('',#11890,#11889,#5935,.T.);
#14794=EDGE_CURVE('',#11890,#11891,#5936,.T.);
#14795=EDGE_CURVE('',#11891,#11892,#5937,.T.);
#14796=EDGE_CURVE('',#11892,#11893,#5938,.T.);
#14797=EDGE_CURVE('',#11893,#11894,#5939,.T.);
#14798=EDGE_CURVE('',#11894,#11895,#5940,.T.);
#14799=EDGE_CURVE('',#11895,#11896,#5941,.T.);
#14800=EDGE_CURVE('',#11896,#11897,#5942,.T.);
#14801=EDGE_CURVE('',#11897,#11898,#5943,.T.);
#14802=EDGE_CURVE('',#11898,#11899,#5944,.T.);
#14803=EDGE_CURVE('',#11899,#11900,#5945,.T.);
#14804=EDGE_CURVE('',#11900,#11901,#5946,.T.);
#14805=EDGE_CURVE('',#11901,#11902,#5947,.T.);
#14806=EDGE_CURVE('',#11902,#11903,#5948,.T.);
#14807=EDGE_CURVE('',#11903,#11904,#5949,.T.);
#14808=EDGE_CURVE('',#11904,#11905,#5950,.T.);
#14809=EDGE_CURVE('',#11905,#11906,#5951,.T.);
#14810=EDGE_CURVE('',#11907,#11906,#5952,.T.);
#14811=EDGE_CURVE('',#11907,#11908,#5953,.T.);
#14812=EDGE_CURVE('',#11908,#11909,#5954,.T.);
#14813=EDGE_CURVE('',#11910,#11909,#5955,.T.);
#14814=EDGE_CURVE('',#11910,#11911,#5956,.T.);
#14815=EDGE_CURVE('',#11911,#11912,#5957,.T.);
#14816=EDGE_CURVE('',#11912,#11913,#5958,.T.);
#14817=EDGE_CURVE('',#11913,#11914,#5959,.T.);
#14818=EDGE_CURVE('',#11914,#11915,#5960,.T.);
#14819=EDGE_CURVE('',#11915,#11916,#5961,.T.);
#14820=EDGE_CURVE('',#11916,#11917,#5962,.T.);
#14821=EDGE_CURVE('',#11917,#11918,#5963,.T.);
#14822=EDGE_CURVE('',#11918,#11919,#5964,.T.);
#14823=EDGE_CURVE('',#11919,#11920,#5965,.T.);
#14824=EDGE_CURVE('',#11920,#11921,#5966,.T.);
#14825=EDGE_CURVE('',#11921,#11922,#5967,.T.);
#14826=EDGE_CURVE('',#11922,#11923,#5968,.T.);
#14827=EDGE_CURVE('',#11923,#11924,#5969,.T.);
#14828=EDGE_CURVE('',#11924,#11925,#5970,.T.);
#14829=EDGE_CURVE('',#11925,#11926,#5971,.T.);
#14830=EDGE_CURVE('',#11927,#11926,#5972,.T.);
#14831=EDGE_CURVE('',#11927,#11928,#5973,.T.);
#14832=EDGE_CURVE('',#11928,#11929,#5974,.T.);
#14833=EDGE_CURVE('',#11930,#11929,#5975,.T.);
#14834=EDGE_CURVE('',#11930,#11931,#5976,.T.);
#14835=EDGE_CURVE('',#11931,#11932,#5977,.T.);
#14836=EDGE_CURVE('',#11932,#11933,#5978,.T.);
#14837=EDGE_CURVE('',#11933,#11934,#5979,.T.);
#14838=EDGE_CURVE('',#11934,#11935,#5980,.T.);
#14839=EDGE_CURVE('',#11935,#11936,#5981,.T.);
#14840=EDGE_CURVE('',#11936,#11937,#5982,.T.);
#14841=EDGE_CURVE('',#11937,#11938,#5983,.T.);
#14842=EDGE_CURVE('',#11938,#11939,#5984,.T.);
#14843=EDGE_CURVE('',#11939,#11940,#5985,.T.);
#14844=EDGE_CURVE('',#11940,#11941,#5986,.T.);
#14845=EDGE_CURVE('',#11941,#11942,#5987,.T.);
#14846=EDGE_CURVE('',#11942,#11943,#5988,.T.);
#14847=EDGE_CURVE('',#11943,#11944,#5989,.T.);
#14848=EDGE_CURVE('',#11944,#11945,#5990,.T.);
#14849=EDGE_CURVE('',#11945,#11946,#5991,.T.);
#14850=EDGE_CURVE('',#11947,#11946,#5992,.T.);
#14851=EDGE_CURVE('',#11947,#11948,#5993,.T.);
#14852=EDGE_CURVE('',#11948,#11949,#5994,.T.);
#14853=EDGE_CURVE('',#11950,#11949,#5995,.T.);
#14854=EDGE_CURVE('',#11950,#11951,#5996,.T.);
#14855=EDGE_CURVE('',#11951,#11952,#5997,.T.);
#14856=EDGE_CURVE('',#11952,#11953,#5998,.T.);
#14857=EDGE_CURVE('',#11953,#11954,#5999,.T.);
#14858=EDGE_CURVE('',#11954,#11955,#6000,.T.);
#14859=EDGE_CURVE('',#11955,#11956,#6001,.T.);
#14860=EDGE_CURVE('',#11956,#11957,#6002,.T.);
#14861=EDGE_CURVE('',#11957,#11958,#6003,.T.);
#14862=EDGE_CURVE('',#11958,#11959,#6004,.T.);
#14863=EDGE_CURVE('',#11959,#11960,#6005,.T.);
#14864=EDGE_CURVE('',#11960,#11961,#6006,.T.);
#14865=EDGE_CURVE('',#11961,#11962,#6007,.T.);
#14866=EDGE_CURVE('',#11962,#11963,#6008,.T.);
#14867=EDGE_CURVE('',#11963,#11964,#6009,.T.);
#14868=EDGE_CURVE('',#11964,#11965,#6010,.T.);
#14869=EDGE_CURVE('',#11965,#11966,#6011,.T.);
#14870=EDGE_CURVE('',#11967,#11966,#6012,.T.);
#14871=EDGE_CURVE('',#11967,#11968,#6013,.T.);
#14872=EDGE_CURVE('',#11968,#11969,#6014,.T.);
#14873=EDGE_CURVE('',#11970,#11969,#6015,.T.);
#14874=EDGE_CURVE('',#11970,#11971,#6016,.T.);
#14875=EDGE_CURVE('',#11971,#11972,#6017,.T.);
#14876=EDGE_CURVE('',#11972,#11973,#6018,.T.);
#14877=EDGE_CURVE('',#11973,#11974,#6019,.T.);
#14878=EDGE_CURVE('',#11974,#11975,#6020,.T.);
#14879=EDGE_CURVE('',#11975,#11976,#6021,.T.);
#14880=EDGE_CURVE('',#11976,#11977,#6022,.T.);
#14881=EDGE_CURVE('',#11977,#11978,#6023,.T.);
#14882=EDGE_CURVE('',#11978,#11979,#6024,.T.);
#14883=EDGE_CURVE('',#11979,#11980,#6025,.T.);
#14884=EDGE_CURVE('',#11980,#11981,#6026,.T.);
#14885=EDGE_CURVE('',#11981,#11982,#6027,.T.);
#14886=EDGE_CURVE('',#11982,#11983,#6028,.T.);
#14887=EDGE_CURVE('',#11983,#11984,#6029,.T.);
#14888=EDGE_CURVE('',#11984,#11985,#6030,.T.);
#14889=EDGE_CURVE('',#11985,#11986,#6031,.T.);
#14890=EDGE_CURVE('',#11987,#11986,#6032,.T.);
#14891=EDGE_CURVE('',#11987,#11988,#6033,.T.);
#14892=EDGE_CURVE('',#11988,#11989,#6034,.T.);
#14893=EDGE_CURVE('',#11990,#11989,#6035,.T.);
#14894=EDGE_CURVE('',#11990,#11991,#6036,.T.);
#14895=EDGE_CURVE('',#11991,#11992,#6037,.T.);
#14896=EDGE_CURVE('',#11992,#11993,#6038,.T.);
#14897=EDGE_CURVE('',#11993,#11994,#6039,.T.);
#14898=EDGE_CURVE('',#11994,#11995,#6040,.T.);
#14899=EDGE_CURVE('',#11995,#11996,#6041,.T.);
#14900=EDGE_CURVE('',#11996,#11997,#6042,.T.);
#14901=EDGE_CURVE('',#11997,#11998,#6043,.T.);
#14902=EDGE_CURVE('',#11998,#11999,#6044,.T.);
#14903=EDGE_CURVE('',#11999,#12000,#6045,.T.);
#14904=EDGE_CURVE('',#12000,#12001,#6046,.T.);
#14905=EDGE_CURVE('',#12001,#12002,#6047,.T.);
#14906=EDGE_CURVE('',#12002,#12003,#6048,.T.);
#14907=EDGE_CURVE('',#12003,#12004,#6049,.T.);
#14908=EDGE_CURVE('',#12004,#12005,#6050,.T.);
#14909=EDGE_CURVE('',#12005,#12006,#6051,.T.);
#14910=EDGE_CURVE('',#12007,#12006,#6052,.T.);
#14911=EDGE_CURVE('',#12007,#12008,#6053,.T.);
#14912=EDGE_CURVE('',#12008,#12009,#6054,.T.);
#14913=EDGE_CURVE('',#12010,#12009,#6055,.T.);
#14914=EDGE_CURVE('',#12010,#12011,#6056,.T.);
#14915=EDGE_CURVE('',#12011,#12012,#6057,.T.);
#14916=EDGE_CURVE('',#12012,#12013,#6058,.T.);
#14917=EDGE_CURVE('',#12013,#12014,#6059,.T.);
#14918=EDGE_CURVE('',#12014,#12015,#6060,.T.);
#14919=EDGE_CURVE('',#12015,#12016,#6061,.T.);
#14920=EDGE_CURVE('',#12016,#12017,#6062,.T.);
#14921=EDGE_CURVE('',#12017,#12018,#6063,.T.);
#14922=EDGE_CURVE('',#12018,#12019,#6064,.T.);
#14923=EDGE_CURVE('',#12019,#12020,#6065,.T.);
#14924=EDGE_CURVE('',#12020,#12021,#6066,.T.);
#14925=EDGE_CURVE('',#12021,#12022,#6067,.T.);
#14926=EDGE_CURVE('',#12022,#12023,#6068,.T.);
#14927=EDGE_CURVE('',#12023,#12024,#6069,.T.);
#14928=EDGE_CURVE('',#12024,#12025,#6070,.T.);
#14929=EDGE_CURVE('',#12025,#12026,#6071,.T.);
#14930=EDGE_CURVE('',#12027,#12026,#6072,.T.);
#14931=EDGE_CURVE('',#12027,#12028,#6073,.T.);
#14932=EDGE_CURVE('',#12028,#12029,#6074,.T.);
#14933=EDGE_CURVE('',#12030,#12029,#6075,.T.);
#14934=EDGE_CURVE('',#12030,#12031,#6076,.T.);
#14935=EDGE_CURVE('',#12031,#12032,#6077,.T.);
#14936=EDGE_CURVE('',#12032,#12033,#6078,.T.);
#14937=EDGE_CURVE('',#12033,#12034,#6079,.T.);
#14938=EDGE_CURVE('',#12034,#12035,#6080,.T.);
#14939=EDGE_CURVE('',#12035,#12036,#6081,.T.);
#14940=EDGE_CURVE('',#12036,#12037,#6082,.T.);
#14941=EDGE_CURVE('',#12037,#12038,#6083,.T.);
#14942=EDGE_CURVE('',#12038,#12039,#6084,.T.);
#14943=EDGE_CURVE('',#12039,#12040,#6085,.T.);
#14944=EDGE_CURVE('',#12040,#12041,#6086,.T.);
#14945=EDGE_CURVE('',#12041,#12042,#6087,.T.);
#14946=EDGE_CURVE('',#12042,#12043,#6088,.T.);
#14947=EDGE_CURVE('',#12043,#12044,#6089,.T.);
#14948=EDGE_CURVE('',#12044,#12045,#6090,.T.);
#14949=EDGE_CURVE('',#12045,#12046,#6091,.T.);
#14950=EDGE_CURVE('',#12047,#12046,#6092,.T.);
#14951=EDGE_CURVE('',#12047,#12048,#6093,.T.);
#14952=EDGE_CURVE('',#12048,#12049,#6094,.T.);
#14953=EDGE_CURVE('',#12050,#12049,#6095,.T.);
#14954=EDGE_CURVE('',#12050,#12051,#6096,.T.);
#14955=EDGE_CURVE('',#12051,#12052,#6097,.T.);
#14956=EDGE_CURVE('',#12052,#12053,#6098,.T.);
#14957=EDGE_CURVE('',#12053,#12054,#6099,.T.);
#14958=EDGE_CURVE('',#12054,#12055,#6100,.T.);
#14959=EDGE_CURVE('',#12055,#12056,#6101,.T.);
#14960=EDGE_CURVE('',#12056,#12057,#6102,.T.);
#14961=EDGE_CURVE('',#12057,#12058,#6103,.T.);
#14962=EDGE_CURVE('',#12058,#12059,#6104,.T.);
#14963=EDGE_CURVE('',#12059,#12060,#6105,.T.);
#14964=EDGE_CURVE('',#12060,#12061,#6106,.T.);
#14965=EDGE_CURVE('',#12061,#12062,#6107,.T.);
#14966=EDGE_CURVE('',#12062,#12063,#6108,.T.);
#14967=EDGE_CURVE('',#12063,#12064,#6109,.T.);
#14968=EDGE_CURVE('',#12064,#12065,#6110,.T.);
#14969=EDGE_CURVE('',#12065,#12066,#6111,.T.);
#14970=EDGE_CURVE('',#12067,#12066,#6112,.T.);
#14971=EDGE_CURVE('',#12067,#12068,#6113,.T.);
#14972=EDGE_CURVE('',#12068,#12069,#6114,.T.);
#14973=EDGE_CURVE('',#12070,#12069,#6115,.T.);
#14974=EDGE_CURVE('',#12070,#12071,#6116,.T.);
#14975=EDGE_CURVE('',#12071,#12072,#6117,.T.);
#14976=EDGE_CURVE('',#12072,#12073,#6118,.T.);
#14977=EDGE_CURVE('',#12073,#12074,#6119,.T.);
#14978=EDGE_CURVE('',#12074,#12075,#6120,.T.);
#14979=EDGE_CURVE('',#12075,#12076,#6121,.T.);
#14980=EDGE_CURVE('',#12076,#12077,#6122,.T.);
#14981=EDGE_CURVE('',#12077,#12078,#6123,.T.);
#14982=EDGE_CURVE('',#12078,#12079,#6124,.T.);
#14983=EDGE_CURVE('',#12079,#12080,#6125,.T.);
#14984=EDGE_CURVE('',#12080,#12081,#6126,.T.);
#14985=EDGE_CURVE('',#12081,#12082,#6127,.T.);
#14986=EDGE_CURVE('',#12082,#12083,#6128,.T.);
#14987=EDGE_CURVE('',#12083,#12084,#6129,.T.);
#14988=EDGE_CURVE('',#12084,#12085,#6130,.T.);
#14989=EDGE_CURVE('',#12085,#12086,#6131,.T.);
#14990=EDGE_CURVE('',#12087,#12086,#6132,.T.);
#14991=EDGE_CURVE('',#12087,#11850,#6133,.T.);
#14992=EDGE_CURVE('',#12088,#12088,#10577,.T.);
#14993=EDGE_CURVE('',#11844,#12089,#6134,.T.);
#14994=EDGE_CURVE('',#12090,#12089,#6135,.T.);
#14995=EDGE_CURVE('',#12091,#12090,#6136,.T.);
#14996=EDGE_CURVE('',#11851,#12091,#6137,.T.);
#14997=EDGE_CURVE('',#11849,#12092,#6138,.T.);
#14998=EDGE_CURVE('',#12089,#12092,#6139,.T.);
#14999=EDGE_CURVE('',#12093,#12070,#6140,.T.);
#15000=EDGE_CURVE('',#12069,#12094,#6141,.F.);
#15001=EDGE_CURVE('',#12094,#12095,#6142,.T.);
#15002=EDGE_CURVE('',#12095,#12096,#6143,.T.);
#15003=EDGE_CURVE('',#12096,#12093,#6144,.T.);
#15004=EDGE_CURVE('',#12093,#12097,#6145,.T.);
#15005=EDGE_CURVE('',#12098,#12097,#6146,.T.);
#15006=EDGE_CURVE('',#12099,#12098,#6147,.T.);
#15007=EDGE_CURVE('',#12071,#12099,#6148,.T.);
#15008=EDGE_CURVE('',#12096,#12100,#6149,.T.);
#15009=EDGE_CURVE('',#12097,#12100,#6150,.T.);
#15010=EDGE_CURVE('',#12101,#12050,#6151,.T.);
#15011=EDGE_CURVE('',#12049,#12102,#6152,.F.);
#15012=EDGE_CURVE('',#12102,#12103,#6153,.T.);
#15013=EDGE_CURVE('',#12103,#12104,#6154,.T.);
#15014=EDGE_CURVE('',#12104,#12101,#6155,.T.);
#15015=EDGE_CURVE('',#12101,#12105,#6156,.T.);
#15016=EDGE_CURVE('',#12106,#12105,#6157,.T.);
#15017=EDGE_CURVE('',#12107,#12106,#6158,.T.);
#15018=EDGE_CURVE('',#12051,#12107,#6159,.T.);
#15019=EDGE_CURVE('',#12104,#12108,#6160,.T.);
#15020=EDGE_CURVE('',#12105,#12108,#6161,.T.);
#15021=EDGE_CURVE('',#12109,#12030,#6162,.T.);
#15022=EDGE_CURVE('',#12029,#12110,#6163,.F.);
#15023=EDGE_CURVE('',#12110,#12111,#6164,.T.);
#15024=EDGE_CURVE('',#12111,#12112,#6165,.T.);
#15025=EDGE_CURVE('',#12112,#12109,#6166,.T.);
#15026=EDGE_CURVE('',#12109,#12113,#6167,.T.);
#15027=EDGE_CURVE('',#12114,#12113,#6168,.T.);
#15028=EDGE_CURVE('',#12115,#12114,#6169,.T.);
#15029=EDGE_CURVE('',#12031,#12115,#6170,.T.);
#15030=EDGE_CURVE('',#12112,#12116,#6171,.T.);
#15031=EDGE_CURVE('',#12113,#12116,#6172,.T.);
#15032=EDGE_CURVE('',#12117,#12010,#6173,.T.);
#15033=EDGE_CURVE('',#12009,#12118,#6174,.F.);
#15034=EDGE_CURVE('',#12118,#12119,#6175,.T.);
#15035=EDGE_CURVE('',#12119,#12120,#6176,.T.);
#15036=EDGE_CURVE('',#12120,#12117,#6177,.T.);
#15037=EDGE_CURVE('',#12117,#12121,#6178,.T.);
#15038=EDGE_CURVE('',#12122,#12121,#6179,.T.);
#15039=EDGE_CURVE('',#12123,#12122,#6180,.T.);
#15040=EDGE_CURVE('',#12011,#12123,#6181,.T.);
#15041=EDGE_CURVE('',#12120,#12124,#6182,.T.);
#15042=EDGE_CURVE('',#12121,#12124,#6183,.T.);
#15043=EDGE_CURVE('',#12125,#11990,#6184,.T.);
#15044=EDGE_CURVE('',#11989,#12126,#6185,.F.);
#15045=EDGE_CURVE('',#12126,#12127,#6186,.T.);
#15046=EDGE_CURVE('',#12127,#12128,#6187,.T.);
#15047=EDGE_CURVE('',#12128,#12125,#6188,.T.);
#15048=EDGE_CURVE('',#12125,#12129,#6189,.T.);
#15049=EDGE_CURVE('',#12130,#12129,#6190,.T.);
#15050=EDGE_CURVE('',#12131,#12130,#6191,.T.);
#15051=EDGE_CURVE('',#11991,#12131,#6192,.T.);
#15052=EDGE_CURVE('',#12128,#12132,#6193,.T.);
#15053=EDGE_CURVE('',#12129,#12132,#6194,.T.);
#15054=EDGE_CURVE('',#12133,#11970,#6195,.T.);
#15055=EDGE_CURVE('',#11969,#12134,#6196,.F.);
#15056=EDGE_CURVE('',#12134,#12135,#6197,.T.);
#15057=EDGE_CURVE('',#12135,#12136,#6198,.T.);
#15058=EDGE_CURVE('',#12136,#12133,#6199,.T.);
#15059=EDGE_CURVE('',#12133,#12137,#6200,.T.);
#15060=EDGE_CURVE('',#12138,#12137,#6201,.T.);
#15061=EDGE_CURVE('',#12139,#12138,#6202,.T.);
#15062=EDGE_CURVE('',#11971,#12139,#6203,.T.);
#15063=EDGE_CURVE('',#12136,#12140,#6204,.T.);
#15064=EDGE_CURVE('',#12137,#12140,#6205,.T.);
#15065=EDGE_CURVE('',#12141,#11950,#6206,.T.);
#15066=EDGE_CURVE('',#11949,#12142,#6207,.F.);
#15067=EDGE_CURVE('',#12142,#12143,#6208,.T.);
#15068=EDGE_CURVE('',#12143,#12144,#6209,.T.);
#15069=EDGE_CURVE('',#12144,#12141,#6210,.T.);
#15070=EDGE_CURVE('',#12141,#12145,#6211,.T.);
#15071=EDGE_CURVE('',#12146,#12145,#6212,.T.);
#15072=EDGE_CURVE('',#12147,#12146,#6213,.T.);
#15073=EDGE_CURVE('',#11951,#12147,#6214,.T.);
#15074=EDGE_CURVE('',#12144,#12148,#6215,.T.);
#15075=EDGE_CURVE('',#12145,#12148,#6216,.T.);
#15076=EDGE_CURVE('',#12149,#11930,#6217,.T.);
#15077=EDGE_CURVE('',#11929,#12150,#6218,.F.);
#15078=EDGE_CURVE('',#12150,#12151,#6219,.T.);
#15079=EDGE_CURVE('',#12151,#12152,#6220,.T.);
#15080=EDGE_CURVE('',#12152,#12149,#6221,.T.);
#15081=EDGE_CURVE('',#12149,#12153,#6222,.T.);
#15082=EDGE_CURVE('',#12154,#12153,#6223,.T.);
#15083=EDGE_CURVE('',#12155,#12154,#6224,.T.);
#15084=EDGE_CURVE('',#11931,#12155,#6225,.T.);
#15085=EDGE_CURVE('',#12152,#12156,#6226,.T.);
#15086=EDGE_CURVE('',#12153,#12156,#6227,.T.);
#15087=EDGE_CURVE('',#12157,#11910,#6228,.T.);
#15088=EDGE_CURVE('',#11909,#12158,#6229,.F.);
#15089=EDGE_CURVE('',#12158,#12159,#6230,.T.);
#15090=EDGE_CURVE('',#12159,#12160,#6231,.T.);
#15091=EDGE_CURVE('',#12160,#12157,#6232,.T.);
#15092=EDGE_CURVE('',#12157,#12161,#6233,.T.);
#15093=EDGE_CURVE('',#12162,#12161,#6234,.T.);
#15094=EDGE_CURVE('',#12163,#12162,#6235,.T.);
#15095=EDGE_CURVE('',#11911,#12163,#6236,.T.);
#15096=EDGE_CURVE('',#12160,#12164,#6237,.T.);
#15097=EDGE_CURVE('',#12161,#12164,#6238,.T.);
#15098=EDGE_CURVE('',#12165,#11890,#6239,.T.);
#15099=EDGE_CURVE('',#11889,#12166,#6240,.F.);
#15100=EDGE_CURVE('',#12166,#12167,#6241,.T.);
#15101=EDGE_CURVE('',#12167,#12168,#6242,.T.);
#15102=EDGE_CURVE('',#12168,#12165,#6243,.T.);
#15103=EDGE_CURVE('',#12165,#12169,#6244,.T.);
#15104=EDGE_CURVE('',#12170,#12169,#6245,.T.);
#15105=EDGE_CURVE('',#12171,#12170,#6246,.T.);
#15106=EDGE_CURVE('',#11891,#12171,#6247,.T.);
#15107=EDGE_CURVE('',#12168,#12172,#6248,.T.);
#15108=EDGE_CURVE('',#12169,#12172,#6249,.T.);
#15109=EDGE_CURVE('',#12173,#11870,#6250,.T.);
#15110=EDGE_CURVE('',#11869,#12174,#6251,.F.);
#15111=EDGE_CURVE('',#12174,#12175,#6252,.T.);
#15112=EDGE_CURVE('',#12175,#12176,#6253,.T.);
#15113=EDGE_CURVE('',#12176,#12173,#6254,.T.);
#15114=EDGE_CURVE('',#12173,#12177,#6255,.T.);
#15115=EDGE_CURVE('',#12178,#12177,#6256,.T.);
#15116=EDGE_CURVE('',#12179,#12178,#6257,.T.);
#15117=EDGE_CURVE('',#11871,#12179,#6258,.T.);
#15118=EDGE_CURVE('',#12176,#12180,#6259,.T.);
#15119=EDGE_CURVE('',#12177,#12180,#6260,.T.);
#15120=EDGE_CURVE('',#12181,#12182,#6261,.T.);
#15121=EDGE_CURVE('',#12182,#12183,#6262,.T.);
#15122=EDGE_CURVE('',#12183,#11867,#6263,.F.);
#15123=EDGE_CURVE('',#11866,#12184,#6264,.T.);
#15124=EDGE_CURVE('',#12184,#12181,#6265,.T.);
#15125=EDGE_CURVE('',#12182,#12185,#6266,.T.);
#15126=EDGE_CURVE('',#12186,#12185,#6267,.T.);
#15127=EDGE_CURVE('',#12183,#12186,#6268,.T.);
#15128=EDGE_CURVE('',#12181,#12187,#6269,.T.);
#15129=EDGE_CURVE('',#12185,#12187,#6270,.T.);
#15130=EDGE_CURVE('',#12188,#12189,#6271,.T.);
#15131=EDGE_CURVE('',#12189,#12190,#6272,.T.);
#15132=EDGE_CURVE('',#12190,#12087,#6273,.F.);
#15133=EDGE_CURVE('',#12086,#12191,#6274,.T.);
#15134=EDGE_CURVE('',#12191,#12188,#6275,.T.);
#15135=EDGE_CURVE('',#12189,#12192,#6276,.T.);
#15136=EDGE_CURVE('',#12193,#12192,#6277,.T.);
#15137=EDGE_CURVE('',#12190,#12193,#6278,.T.);
#15138=EDGE_CURVE('',#12188,#12194,#6279,.T.);
#15139=EDGE_CURVE('',#12192,#12194,#6280,.T.);
#15140=EDGE_CURVE('',#12195,#12196,#6281,.T.);
#15141=EDGE_CURVE('',#12196,#12197,#6282,.T.);
#15142=EDGE_CURVE('',#12197,#12067,#6283,.F.);
#15143=EDGE_CURVE('',#12066,#12198,#6284,.T.);
#15144=EDGE_CURVE('',#12198,#12195,#6285,.T.);
#15145=EDGE_CURVE('',#12196,#12199,#6286,.T.);
#15146=EDGE_CURVE('',#12200,#12199,#6287,.T.);
#15147=EDGE_CURVE('',#12197,#12200,#6288,.T.);
#15148=EDGE_CURVE('',#12195,#12201,#6289,.T.);
#15149=EDGE_CURVE('',#12199,#12201,#6290,.T.);
#15150=EDGE_CURVE('',#12202,#12203,#6291,.T.);
#15151=EDGE_CURVE('',#12203,#12204,#6292,.T.);
#15152=EDGE_CURVE('',#12204,#12047,#6293,.F.);
#15153=EDGE_CURVE('',#12046,#12205,#6294,.T.);
#15154=EDGE_CURVE('',#12205,#12202,#6295,.T.);
#15155=EDGE_CURVE('',#12203,#12206,#6296,.T.);
#15156=EDGE_CURVE('',#12207,#12206,#6297,.T.);
#15157=EDGE_CURVE('',#12204,#12207,#6298,.T.);
#15158=EDGE_CURVE('',#12202,#12208,#6299,.T.);
#15159=EDGE_CURVE('',#12206,#12208,#6300,.T.);
#15160=EDGE_CURVE('',#12209,#12210,#6301,.T.);
#15161=EDGE_CURVE('',#12210,#12211,#6302,.T.);
#15162=EDGE_CURVE('',#12211,#12027,#6303,.F.);
#15163=EDGE_CURVE('',#12026,#12212,#6304,.T.);
#15164=EDGE_CURVE('',#12212,#12209,#6305,.T.);
#15165=EDGE_CURVE('',#12210,#12213,#6306,.T.);
#15166=EDGE_CURVE('',#12214,#12213,#6307,.T.);
#15167=EDGE_CURVE('',#12211,#12214,#6308,.T.);
#15168=EDGE_CURVE('',#12209,#12215,#6309,.T.);
#15169=EDGE_CURVE('',#12213,#12215,#6310,.T.);
#15170=EDGE_CURVE('',#12216,#12217,#6311,.T.);
#15171=EDGE_CURVE('',#12217,#12218,#6312,.T.);
#15172=EDGE_CURVE('',#12218,#12007,#6313,.F.);
#15173=EDGE_CURVE('',#12006,#12219,#6314,.T.);
#15174=EDGE_CURVE('',#12219,#12216,#6315,.T.);
#15175=EDGE_CURVE('',#12217,#12220,#6316,.T.);
#15176=EDGE_CURVE('',#12221,#12220,#6317,.T.);
#15177=EDGE_CURVE('',#12218,#12221,#6318,.T.);
#15178=EDGE_CURVE('',#12216,#12222,#6319,.T.);
#15179=EDGE_CURVE('',#12220,#12222,#6320,.T.);
#15180=EDGE_CURVE('',#12223,#12224,#6321,.T.);
#15181=EDGE_CURVE('',#12224,#12225,#6322,.T.);
#15182=EDGE_CURVE('',#12225,#11987,#6323,.F.);
#15183=EDGE_CURVE('',#11986,#12226,#6324,.T.);
#15184=EDGE_CURVE('',#12226,#12223,#6325,.T.);
#15185=EDGE_CURVE('',#12224,#12227,#6326,.T.);
#15186=EDGE_CURVE('',#12228,#12227,#6327,.T.);
#15187=EDGE_CURVE('',#12225,#12228,#6328,.T.);
#15188=EDGE_CURVE('',#12223,#12229,#6329,.T.);
#15189=EDGE_CURVE('',#12227,#12229,#6330,.T.);
#15190=EDGE_CURVE('',#12230,#12231,#6331,.T.);
#15191=EDGE_CURVE('',#12231,#12232,#6332,.T.);
#15192=EDGE_CURVE('',#12232,#11967,#6333,.F.);
#15193=EDGE_CURVE('',#11966,#12233,#6334,.T.);
#15194=EDGE_CURVE('',#12233,#12230,#6335,.T.);
#15195=EDGE_CURVE('',#12231,#12234,#6336,.T.);
#15196=EDGE_CURVE('',#12235,#12234,#6337,.T.);
#15197=EDGE_CURVE('',#12232,#12235,#6338,.T.);
#15198=EDGE_CURVE('',#12230,#12236,#6339,.T.);
#15199=EDGE_CURVE('',#12234,#12236,#6340,.T.);
#15200=EDGE_CURVE('',#12237,#12238,#6341,.T.);
#15201=EDGE_CURVE('',#12238,#12239,#6342,.T.);
#15202=EDGE_CURVE('',#12239,#11947,#6343,.F.);
#15203=EDGE_CURVE('',#11946,#12240,#6344,.T.);
#15204=EDGE_CURVE('',#12240,#12237,#6345,.T.);
#15205=EDGE_CURVE('',#12238,#12241,#6346,.T.);
#15206=EDGE_CURVE('',#12242,#12241,#6347,.T.);
#15207=EDGE_CURVE('',#12239,#12242,#6348,.T.);
#15208=EDGE_CURVE('',#12237,#12243,#6349,.T.);
#15209=EDGE_CURVE('',#12241,#12243,#6350,.T.);
#15210=EDGE_CURVE('',#12244,#12245,#6351,.T.);
#15211=EDGE_CURVE('',#12245,#12246,#6352,.T.);
#15212=EDGE_CURVE('',#12246,#11927,#6353,.F.);
#15213=EDGE_CURVE('',#11926,#12247,#6354,.T.);
#15214=EDGE_CURVE('',#12247,#12244,#6355,.T.);
#15215=EDGE_CURVE('',#12245,#12248,#6356,.T.);
#15216=EDGE_CURVE('',#12249,#12248,#6357,.T.);
#15217=EDGE_CURVE('',#12246,#12249,#6358,.T.);
#15218=EDGE_CURVE('',#12244,#12250,#6359,.T.);
#15219=EDGE_CURVE('',#12248,#12250,#6360,.T.);
#15220=EDGE_CURVE('',#12251,#12252,#6361,.T.);
#15221=EDGE_CURVE('',#12252,#12253,#6362,.T.);
#15222=EDGE_CURVE('',#12253,#11907,#6363,.F.);
#15223=EDGE_CURVE('',#11906,#12254,#6364,.T.);
#15224=EDGE_CURVE('',#12254,#12251,#6365,.T.);
#15225=EDGE_CURVE('',#12252,#12255,#6366,.T.);
#15226=EDGE_CURVE('',#12256,#12255,#6367,.T.);
#15227=EDGE_CURVE('',#12253,#12256,#6368,.T.);
#15228=EDGE_CURVE('',#12251,#12257,#6369,.T.);
#15229=EDGE_CURVE('',#12255,#12257,#6370,.T.);
#15230=EDGE_CURVE('',#12258,#12259,#6371,.T.);
#15231=EDGE_CURVE('',#12259,#12260,#6372,.T.);
#15232=EDGE_CURVE('',#12260,#11887,#6373,.F.);
#15233=EDGE_CURVE('',#11886,#12261,#6374,.T.);
#15234=EDGE_CURVE('',#12261,#12258,#6375,.T.);
#15235=EDGE_CURVE('',#12259,#12262,#6376,.T.);
#15236=EDGE_CURVE('',#12263,#12262,#6377,.T.);
#15237=EDGE_CURVE('',#12260,#12263,#6378,.T.);
#15238=EDGE_CURVE('',#12258,#12264,#6379,.T.);
#15239=EDGE_CURVE('',#12262,#12264,#6380,.T.);
#15240=EDGE_CURVE('',#12180,#12265,#6381,.T.);
#15241=EDGE_CURVE('',#12265,#12266,#6382,.T.);
#15242=EDGE_CURVE('',#12266,#12267,#6383,.F.);
#15243=EDGE_CURVE('',#12267,#12178,#6384,.T.);
#15244=EDGE_CURVE('',#12267,#12268,#6385,.T.);
#15245=EDGE_CURVE('',#12268,#12269,#6386,.T.);
#15246=EDGE_CURVE('',#12270,#12269,#6387,.T.);
#15247=EDGE_CURVE('',#12270,#12271,#6388,.T.);
#15248=EDGE_CURVE('',#12271,#12272,#6389,.T.);
#15249=EDGE_CURVE('',#12272,#12273,#6390,.T.);
#15250=EDGE_CURVE('',#12273,#12274,#6391,.T.);
#15251=EDGE_CURVE('',#12274,#12275,#6392,.T.);
#15252=EDGE_CURVE('',#12275,#12276,#6393,.T.);
#15253=EDGE_CURVE('',#12276,#12277,#6394,.T.);
#15254=EDGE_CURVE('',#12277,#12278,#6395,.T.);
#15255=EDGE_CURVE('',#12278,#12279,#6396,.T.);
#15256=EDGE_CURVE('',#12279,#12280,#6397,.T.);
#15257=EDGE_CURVE('',#12280,#12281,#6398,.T.);
#15258=EDGE_CURVE('',#12281,#12282,#6399,.T.);
#15259=EDGE_CURVE('',#12282,#12283,#6400,.T.);
#15260=EDGE_CURVE('',#12283,#12284,#6401,.T.);
#15261=EDGE_CURVE('',#12284,#12091,#6402,.T.);
#15262=EDGE_CURVE('',#12285,#12090,#6403,.T.);
#15263=EDGE_CURVE('',#12285,#12286,#6404,.T.);
#15264=EDGE_CURVE('',#12286,#12287,#6405,.T.);
#15265=EDGE_CURVE('',#12288,#12287,#6406,.T.);
#15266=EDGE_CURVE('',#12288,#12289,#6407,.T.);
#15267=EDGE_CURVE('',#12289,#12290,#6408,.T.);
#15268=EDGE_CURVE('',#12290,#12291,#6409,.T.);
#15269=EDGE_CURVE('',#12291,#12292,#6410,.T.);
#15270=EDGE_CURVE('',#12292,#12293,#6411,.T.);
#15271=EDGE_CURVE('',#12293,#12294,#6412,.T.);
#15272=EDGE_CURVE('',#12294,#12295,#6413,.T.);
#15273=EDGE_CURVE('',#12295,#12296,#6414,.T.);
#15274=EDGE_CURVE('',#12296,#12297,#6415,.T.);
#15275=EDGE_CURVE('',#12297,#12298,#6416,.T.);
#15276=EDGE_CURVE('',#12298,#12299,#6417,.T.);
#15277=EDGE_CURVE('',#12299,#12300,#6418,.T.);
#15278=EDGE_CURVE('',#12300,#12301,#6419,.T.);
#15279=EDGE_CURVE('',#12301,#12302,#6420,.T.);
#15280=EDGE_CURVE('',#12302,#12099,#6421,.T.);
#15281=EDGE_CURVE('',#12303,#12098,#6422,.T.);
#15282=EDGE_CURVE('',#12303,#12304,#6423,.T.);
#15283=EDGE_CURVE('',#12304,#12305,#6424,.T.);
#15284=EDGE_CURVE('',#12306,#12305,#6425,.T.);
#15285=EDGE_CURVE('',#12306,#12307,#6426,.T.);
#15286=EDGE_CURVE('',#12307,#12308,#6427,.T.);
#15287=EDGE_CURVE('',#12308,#12309,#6428,.T.);
#15288=EDGE_CURVE('',#12309,#12310,#6429,.T.);
#15289=EDGE_CURVE('',#12310,#12311,#6430,.T.);
#15290=EDGE_CURVE('',#12311,#12312,#6431,.T.);
#15291=EDGE_CURVE('',#12312,#12313,#6432,.T.);
#15292=EDGE_CURVE('',#12313,#12314,#6433,.T.);
#15293=EDGE_CURVE('',#12314,#12315,#6434,.T.);
#15294=EDGE_CURVE('',#12315,#12316,#6435,.T.);
#15295=EDGE_CURVE('',#12316,#12317,#6436,.T.);
#15296=EDGE_CURVE('',#12317,#12318,#6437,.T.);
#15297=EDGE_CURVE('',#12318,#12319,#6438,.T.);
#15298=EDGE_CURVE('',#12319,#12320,#6439,.T.);
#15299=EDGE_CURVE('',#12320,#12107,#6440,.T.);
#15300=EDGE_CURVE('',#12321,#12106,#6441,.T.);
#15301=EDGE_CURVE('',#12321,#12322,#6442,.T.);
#15302=EDGE_CURVE('',#12322,#12323,#6443,.T.);
#15303=EDGE_CURVE('',#12324,#12323,#6444,.T.);
#15304=EDGE_CURVE('',#12324,#12325,#6445,.T.);
#15305=EDGE_CURVE('',#12325,#12326,#6446,.T.);
#15306=EDGE_CURVE('',#12326,#12327,#6447,.T.);
#15307=EDGE_CURVE('',#12327,#12328,#6448,.T.);
#15308=EDGE_CURVE('',#12328,#12329,#6449,.T.);
#15309=EDGE_CURVE('',#12329,#12330,#6450,.T.);
#15310=EDGE_CURVE('',#12330,#12331,#6451,.T.);
#15311=EDGE_CURVE('',#12331,#12332,#6452,.T.);
#15312=EDGE_CURVE('',#12332,#12333,#6453,.T.);
#15313=EDGE_CURVE('',#12333,#12334,#6454,.T.);
#15314=EDGE_CURVE('',#12334,#12335,#6455,.T.);
#15315=EDGE_CURVE('',#12335,#12336,#6456,.T.);
#15316=EDGE_CURVE('',#12336,#12337,#6457,.T.);
#15317=EDGE_CURVE('',#12337,#12338,#6458,.T.);
#15318=EDGE_CURVE('',#12338,#12115,#6459,.T.);
#15319=EDGE_CURVE('',#12339,#12114,#6460,.T.);
#15320=EDGE_CURVE('',#12339,#12340,#6461,.T.);
#15321=EDGE_CURVE('',#12340,#12341,#6462,.T.);
#15322=EDGE_CURVE('',#12342,#12341,#6463,.T.);
#15323=EDGE_CURVE('',#12342,#12343,#6464,.T.);
#15324=EDGE_CURVE('',#12343,#12344,#6465,.T.);
#15325=EDGE_CURVE('',#12344,#12345,#6466,.T.);
#15326=EDGE_CURVE('',#12345,#12346,#6467,.T.);
#15327=EDGE_CURVE('',#12346,#12347,#6468,.T.);
#15328=EDGE_CURVE('',#12347,#12348,#6469,.T.);
#15329=EDGE_CURVE('',#12348,#12349,#6470,.T.);
#15330=EDGE_CURVE('',#12349,#12350,#6471,.T.);
#15331=EDGE_CURVE('',#12350,#12351,#6472,.T.);
#15332=EDGE_CURVE('',#12351,#12352,#6473,.T.);
#15333=EDGE_CURVE('',#12352,#12353,#6474,.T.);
#15334=EDGE_CURVE('',#12353,#12354,#6475,.T.);
#15335=EDGE_CURVE('',#12354,#12355,#6476,.T.);
#15336=EDGE_CURVE('',#12355,#12356,#6477,.T.);
#15337=EDGE_CURVE('',#12356,#12123,#6478,.T.);
#15338=EDGE_CURVE('',#12357,#12122,#6479,.T.);
#15339=EDGE_CURVE('',#12357,#12358,#6480,.T.);
#15340=EDGE_CURVE('',#12358,#12359,#6481,.T.);
#15341=EDGE_CURVE('',#12360,#12359,#6482,.T.);
#15342=EDGE_CURVE('',#12360,#12361,#6483,.T.);
#15343=EDGE_CURVE('',#12361,#12362,#6484,.T.);
#15344=EDGE_CURVE('',#12362,#12363,#6485,.T.);
#15345=EDGE_CURVE('',#12363,#12364,#6486,.T.);
#15346=EDGE_CURVE('',#12364,#12365,#6487,.T.);
#15347=EDGE_CURVE('',#12365,#12366,#6488,.T.);
#15348=EDGE_CURVE('',#12366,#12367,#6489,.T.);
#15349=EDGE_CURVE('',#12367,#12368,#6490,.T.);
#15350=EDGE_CURVE('',#12368,#12369,#6491,.T.);
#15351=EDGE_CURVE('',#12369,#12370,#6492,.T.);
#15352=EDGE_CURVE('',#12370,#12371,#6493,.T.);
#15353=EDGE_CURVE('',#12371,#12372,#6494,.T.);
#15354=EDGE_CURVE('',#12372,#12373,#6495,.T.);
#15355=EDGE_CURVE('',#12373,#12374,#6496,.T.);
#15356=EDGE_CURVE('',#12374,#12131,#6497,.T.);
#15357=EDGE_CURVE('',#12375,#12130,#6498,.T.);
#15358=EDGE_CURVE('',#12375,#12376,#6499,.T.);
#15359=EDGE_CURVE('',#12376,#12377,#6500,.T.);
#15360=EDGE_CURVE('',#12378,#12377,#6501,.T.);
#15361=EDGE_CURVE('',#12378,#12379,#6502,.T.);
#15362=EDGE_CURVE('',#12379,#12380,#6503,.T.);
#15363=EDGE_CURVE('',#12380,#12381,#6504,.T.);
#15364=EDGE_CURVE('',#12381,#12382,#6505,.T.);
#15365=EDGE_CURVE('',#12382,#12383,#6506,.T.);
#15366=EDGE_CURVE('',#12383,#12384,#6507,.T.);
#15367=EDGE_CURVE('',#12384,#12385,#6508,.T.);
#15368=EDGE_CURVE('',#12385,#12386,#6509,.T.);
#15369=EDGE_CURVE('',#12386,#12387,#6510,.T.);
#15370=EDGE_CURVE('',#12387,#12388,#6511,.T.);
#15371=EDGE_CURVE('',#12388,#12389,#6512,.T.);
#15372=EDGE_CURVE('',#12389,#12390,#6513,.T.);
#15373=EDGE_CURVE('',#12390,#12391,#6514,.T.);
#15374=EDGE_CURVE('',#12391,#12392,#6515,.T.);
#15375=EDGE_CURVE('',#12392,#12139,#6516,.T.);
#15376=EDGE_CURVE('',#12393,#12138,#6517,.T.);
#15377=EDGE_CURVE('',#12393,#12394,#6518,.T.);
#15378=EDGE_CURVE('',#12394,#12395,#6519,.T.);
#15379=EDGE_CURVE('',#12396,#12395,#6520,.T.);
#15380=EDGE_CURVE('',#12396,#12397,#6521,.T.);
#15381=EDGE_CURVE('',#12397,#12398,#6522,.T.);
#15382=EDGE_CURVE('',#12398,#12399,#6523,.T.);
#15383=EDGE_CURVE('',#12399,#12400,#6524,.T.);
#15384=EDGE_CURVE('',#12400,#12401,#6525,.T.);
#15385=EDGE_CURVE('',#12401,#12402,#6526,.T.);
#15386=EDGE_CURVE('',#12402,#12403,#6527,.T.);
#15387=EDGE_CURVE('',#12403,#12404,#6528,.T.);
#15388=EDGE_CURVE('',#12404,#12405,#6529,.T.);
#15389=EDGE_CURVE('',#12405,#12406,#6530,.T.);
#15390=EDGE_CURVE('',#12406,#12407,#6531,.T.);
#15391=EDGE_CURVE('',#12407,#12408,#6532,.T.);
#15392=EDGE_CURVE('',#12408,#12409,#6533,.T.);
#15393=EDGE_CURVE('',#12409,#12410,#6534,.T.);
#15394=EDGE_CURVE('',#12410,#12147,#6535,.T.);
#15395=EDGE_CURVE('',#12411,#12146,#6536,.T.);
#15396=EDGE_CURVE('',#12411,#12412,#6537,.T.);
#15397=EDGE_CURVE('',#12412,#12413,#6538,.T.);
#15398=EDGE_CURVE('',#12414,#12413,#6539,.T.);
#15399=EDGE_CURVE('',#12414,#12415,#6540,.T.);
#15400=EDGE_CURVE('',#12415,#12416,#6541,.T.);
#15401=EDGE_CURVE('',#12416,#12417,#6542,.T.);
#15402=EDGE_CURVE('',#12417,#12418,#6543,.T.);
#15403=EDGE_CURVE('',#12418,#12419,#6544,.T.);
#15404=EDGE_CURVE('',#12419,#12420,#6545,.T.);
#15405=EDGE_CURVE('',#12420,#12421,#6546,.T.);
#15406=EDGE_CURVE('',#12421,#12422,#6547,.T.);
#15407=EDGE_CURVE('',#12422,#12423,#6548,.T.);
#15408=EDGE_CURVE('',#12423,#12424,#6549,.T.);
#15409=EDGE_CURVE('',#12424,#12425,#6550,.T.);
#15410=EDGE_CURVE('',#12425,#12426,#6551,.T.);
#15411=EDGE_CURVE('',#12426,#12427,#6552,.T.);
#15412=EDGE_CURVE('',#12427,#12428,#6553,.T.);
#15413=EDGE_CURVE('',#12428,#12155,#6554,.T.);
#15414=EDGE_CURVE('',#12429,#12154,#6555,.T.);
#15415=EDGE_CURVE('',#12429,#12430,#6556,.T.);
#15416=EDGE_CURVE('',#12430,#12431,#6557,.T.);
#15417=EDGE_CURVE('',#12432,#12431,#6558,.T.);
#15418=EDGE_CURVE('',#12432,#12433,#6559,.T.);
#15419=EDGE_CURVE('',#12433,#12434,#6560,.T.);
#15420=EDGE_CURVE('',#12434,#12435,#6561,.T.);
#15421=EDGE_CURVE('',#12435,#12436,#6562,.T.);
#15422=EDGE_CURVE('',#12436,#12437,#6563,.T.);
#15423=EDGE_CURVE('',#12437,#12438,#6564,.T.);
#15424=EDGE_CURVE('',#12438,#12439,#6565,.T.);
#15425=EDGE_CURVE('',#12439,#12440,#6566,.T.);
#15426=EDGE_CURVE('',#12440,#12441,#6567,.T.);
#15427=EDGE_CURVE('',#12441,#12442,#6568,.T.);
#15428=EDGE_CURVE('',#12442,#12443,#6569,.T.);
#15429=EDGE_CURVE('',#12443,#12444,#6570,.T.);
#15430=EDGE_CURVE('',#12444,#12445,#6571,.T.);
#15431=EDGE_CURVE('',#12445,#12446,#6572,.T.);
#15432=EDGE_CURVE('',#12446,#12163,#6573,.T.);
#15433=EDGE_CURVE('',#12447,#12162,#6574,.T.);
#15434=EDGE_CURVE('',#12447,#12448,#6575,.T.);
#15435=EDGE_CURVE('',#12448,#12449,#6576,.T.);
#15436=EDGE_CURVE('',#12450,#12449,#6577,.T.);
#15437=EDGE_CURVE('',#12450,#12451,#6578,.T.);
#15438=EDGE_CURVE('',#12451,#12452,#6579,.T.);
#15439=EDGE_CURVE('',#12452,#12453,#6580,.T.);
#15440=EDGE_CURVE('',#12453,#12454,#6581,.T.);
#15441=EDGE_CURVE('',#12454,#12455,#6582,.T.);
#15442=EDGE_CURVE('',#12455,#12456,#6583,.T.);
#15443=EDGE_CURVE('',#12456,#12457,#6584,.T.);
#15444=EDGE_CURVE('',#12457,#12458,#6585,.T.);
#15445=EDGE_CURVE('',#12458,#12459,#6586,.T.);
#15446=EDGE_CURVE('',#12459,#12460,#6587,.T.);
#15447=EDGE_CURVE('',#12460,#12461,#6588,.T.);
#15448=EDGE_CURVE('',#12461,#12462,#6589,.T.);
#15449=EDGE_CURVE('',#12462,#12463,#6590,.T.);
#15450=EDGE_CURVE('',#12463,#12464,#6591,.T.);
#15451=EDGE_CURVE('',#12464,#12171,#6592,.T.);
#15452=EDGE_CURVE('',#12465,#12170,#6593,.T.);
#15453=EDGE_CURVE('',#12465,#12466,#6594,.T.);
#15454=EDGE_CURVE('',#12466,#12467,#6595,.T.);
#15455=EDGE_CURVE('',#12468,#12467,#6596,.T.);
#15456=EDGE_CURVE('',#12468,#12469,#6597,.T.);
#15457=EDGE_CURVE('',#12469,#12470,#6598,.T.);
#15458=EDGE_CURVE('',#12470,#12471,#6599,.T.);
#15459=EDGE_CURVE('',#12471,#12472,#6600,.T.);
#15460=EDGE_CURVE('',#12472,#12473,#6601,.T.);
#15461=EDGE_CURVE('',#12473,#12474,#6602,.T.);
#15462=EDGE_CURVE('',#12474,#12475,#6603,.T.);
#15463=EDGE_CURVE('',#12475,#12476,#6604,.T.);
#15464=EDGE_CURVE('',#12476,#12477,#6605,.T.);
#15465=EDGE_CURVE('',#12477,#12478,#6606,.T.);
#15466=EDGE_CURVE('',#12478,#12479,#6607,.T.);
#15467=EDGE_CURVE('',#12479,#12480,#6608,.T.);
#15468=EDGE_CURVE('',#12480,#12481,#6609,.T.);
#15469=EDGE_CURVE('',#12481,#12482,#6610,.T.);
#15470=EDGE_CURVE('',#12482,#12179,#6611,.T.);
#15471=EDGE_CURVE('',#12483,#12483,#10578,.T.);
#15472=EDGE_CURVE('',#12484,#12468,#6612,.T.);
#15473=EDGE_CURVE('',#12467,#12263,#6613,.F.);
#15474=EDGE_CURVE('',#12264,#12484,#6614,.T.);
#15475=EDGE_CURVE('',#12172,#12485,#6615,.T.);
#15476=EDGE_CURVE('',#12485,#12486,#6616,.T.);
#15477=EDGE_CURVE('',#12486,#12465,#6617,.F.);
#15478=EDGE_CURVE('',#12487,#12450,#6618,.T.);
#15479=EDGE_CURVE('',#12449,#12256,#6619,.F.);
#15480=EDGE_CURVE('',#12257,#12487,#6620,.T.);
#15481=EDGE_CURVE('',#12164,#12488,#6621,.T.);
#15482=EDGE_CURVE('',#12488,#12489,#6622,.T.);
#15483=EDGE_CURVE('',#12489,#12447,#6623,.F.);
#15484=EDGE_CURVE('',#12490,#12432,#6624,.T.);
#15485=EDGE_CURVE('',#12431,#12249,#6625,.F.);
#15486=EDGE_CURVE('',#12250,#12490,#6626,.T.);
#15487=EDGE_CURVE('',#12156,#12491,#6627,.T.);
#15488=EDGE_CURVE('',#12491,#12492,#6628,.T.);
#15489=EDGE_CURVE('',#12492,#12429,#6629,.F.);
#15490=EDGE_CURVE('',#12493,#12414,#6630,.T.);
#15491=EDGE_CURVE('',#12413,#12242,#6631,.F.);
#15492=EDGE_CURVE('',#12243,#12493,#6632,.T.);
#15493=EDGE_CURVE('',#12148,#12494,#6633,.T.);
#15494=EDGE_CURVE('',#12494,#12495,#6634,.T.);
#15495=EDGE_CURVE('',#12495,#12411,#6635,.F.);
#15496=EDGE_CURVE('',#12496,#12396,#6636,.T.);
#15497=EDGE_CURVE('',#12395,#12235,#6637,.F.);
#15498=EDGE_CURVE('',#12236,#12496,#6638,.T.);
#15499=EDGE_CURVE('',#12140,#12497,#6639,.T.);
#15500=EDGE_CURVE('',#12497,#12498,#6640,.T.);
#15501=EDGE_CURVE('',#12498,#12393,#6641,.F.);
#15502=EDGE_CURVE('',#12499,#12378,#6642,.T.);
#15503=EDGE_CURVE('',#12377,#12228,#6643,.F.);
#15504=EDGE_CURVE('',#12229,#12499,#6644,.T.);
#15505=EDGE_CURVE('',#12132,#12500,#6645,.T.);
#15506=EDGE_CURVE('',#12500,#12501,#6646,.T.);
#15507=EDGE_CURVE('',#12501,#12375,#6647,.F.);
#15508=EDGE_CURVE('',#12502,#12360,#6648,.T.);
#15509=EDGE_CURVE('',#12359,#12221,#6649,.F.);
#15510=EDGE_CURVE('',#12222,#12502,#6650,.T.);
#15511=EDGE_CURVE('',#12124,#12503,#6651,.T.);
#15512=EDGE_CURVE('',#12503,#12504,#6652,.T.);
#15513=EDGE_CURVE('',#12504,#12357,#6653,.F.);
#15514=EDGE_CURVE('',#12505,#12342,#6654,.T.);
#15515=EDGE_CURVE('',#12341,#12214,#6655,.F.);
#15516=EDGE_CURVE('',#12215,#12505,#6656,.T.);
#15517=EDGE_CURVE('',#12116,#12506,#6657,.T.);
#15518=EDGE_CURVE('',#12506,#12507,#6658,.T.);
#15519=EDGE_CURVE('',#12507,#12339,#6659,.F.);
#15520=EDGE_CURVE('',#12508,#12324,#6660,.T.);
#15521=EDGE_CURVE('',#12323,#12207,#6661,.F.);
#15522=EDGE_CURVE('',#12208,#12508,#6662,.T.);
#15523=EDGE_CURVE('',#12108,#12509,#6663,.T.);
#15524=EDGE_CURVE('',#12509,#12510,#6664,.T.);
#15525=EDGE_CURVE('',#12510,#12321,#6665,.F.);
#15526=EDGE_CURVE('',#12511,#12306,#6666,.T.);
#15527=EDGE_CURVE('',#12305,#12200,#6667,.F.);
#15528=EDGE_CURVE('',#12201,#12511,#6668,.T.);
#15529=EDGE_CURVE('',#12100,#12512,#6669,.T.);
#15530=EDGE_CURVE('',#12512,#12513,#6670,.T.);
#15531=EDGE_CURVE('',#12513,#12303,#6671,.F.);
#15532=EDGE_CURVE('',#12514,#12288,#6672,.T.);
#15533=EDGE_CURVE('',#12287,#12193,#6673,.F.);
#15534=EDGE_CURVE('',#12194,#12514,#6674,.T.);
#15535=EDGE_CURVE('',#12092,#12515,#6675,.T.);
#15536=EDGE_CURVE('',#12515,#12516,#6676,.T.);
#15537=EDGE_CURVE('',#12516,#12285,#6677,.F.);
#15538=EDGE_CURVE('',#12517,#12270,#6678,.T.);
#15539=EDGE_CURVE('',#12269,#12186,#6679,.F.);
#15540=EDGE_CURVE('',#12187,#12517,#6680,.T.);
#15541=EDGE_CURVE('',#11868,#12268,#6681,.T.);
#15542=EDGE_CURVE('',#12174,#12266,#6682,.T.);
#15543=EDGE_CURVE('',#12175,#12265,#6683,.T.);
#15544=EDGE_CURVE('',#11872,#12482,#6684,.T.);
#15545=EDGE_CURVE('',#11873,#12481,#6685,.T.);
#15546=EDGE_CURVE('',#11874,#12480,#6686,.T.);
#15547=EDGE_CURVE('',#11875,#12479,#6687,.T.);
#15548=EDGE_CURVE('',#11876,#12478,#6688,.T.);
#15549=EDGE_CURVE('',#11877,#12477,#6689,.T.);
#15550=EDGE_CURVE('',#11878,#12476,#6690,.T.);
#15551=EDGE_CURVE('',#11879,#12475,#6691,.T.);
#15552=EDGE_CURVE('',#11880,#12474,#6692,.T.);
#15553=EDGE_CURVE('',#11881,#12473,#6693,.T.);
#15554=EDGE_CURVE('',#11882,#12472,#6694,.T.);
#15555=EDGE_CURVE('',#11883,#12471,#6695,.T.);
#15556=EDGE_CURVE('',#11884,#12470,#6696,.T.);
#15557=EDGE_CURVE('',#11885,#12469,#6697,.T.);
#15558=EDGE_CURVE('',#12261,#12484,#6698,.T.);
#15559=EDGE_CURVE('',#11888,#12466,#6699,.T.);
#15560=EDGE_CURVE('',#12166,#12486,#6700,.T.);
#15561=EDGE_CURVE('',#12167,#12485,#6701,.T.);
#15562=EDGE_CURVE('',#11892,#12464,#6702,.T.);
#15563=EDGE_CURVE('',#11893,#12463,#6703,.T.);
#15564=EDGE_CURVE('',#11894,#12462,#6704,.T.);
#15565=EDGE_CURVE('',#11895,#12461,#6705,.T.);
#15566=EDGE_CURVE('',#11896,#12460,#6706,.T.);
#15567=EDGE_CURVE('',#11897,#12459,#6707,.T.);
#15568=EDGE_CURVE('',#11898,#12458,#6708,.T.);
#15569=EDGE_CURVE('',#11899,#12457,#6709,.T.);
#15570=EDGE_CURVE('',#11900,#12456,#6710,.T.);
#15571=EDGE_CURVE('',#11901,#12455,#6711,.T.);
#15572=EDGE_CURVE('',#11902,#12454,#6712,.T.);
#15573=EDGE_CURVE('',#11903,#12453,#6713,.T.);
#15574=EDGE_CURVE('',#11904,#12452,#6714,.T.);
#15575=EDGE_CURVE('',#11905,#12451,#6715,.T.);
#15576=EDGE_CURVE('',#12254,#12487,#6716,.T.);
#15577=EDGE_CURVE('',#11908,#12448,#6717,.T.);
#15578=EDGE_CURVE('',#12158,#12489,#6718,.T.);
#15579=EDGE_CURVE('',#12159,#12488,#6719,.T.);
#15580=EDGE_CURVE('',#11912,#12446,#6720,.T.);
#15581=EDGE_CURVE('',#11913,#12445,#6721,.T.);
#15582=EDGE_CURVE('',#11914,#12444,#6722,.T.);
#15583=EDGE_CURVE('',#11915,#12443,#6723,.T.);
#15584=EDGE_CURVE('',#11916,#12442,#6724,.T.);
#15585=EDGE_CURVE('',#11917,#12441,#6725,.T.);
#15586=EDGE_CURVE('',#11918,#12440,#6726,.T.);
#15587=EDGE_CURVE('',#11919,#12439,#6727,.T.);
#15588=EDGE_CURVE('',#11920,#12438,#6728,.T.);
#15589=EDGE_CURVE('',#11921,#12437,#6729,.T.);
#15590=EDGE_CURVE('',#11922,#12436,#6730,.T.);
#15591=EDGE_CURVE('',#11923,#12435,#6731,.T.);
#15592=EDGE_CURVE('',#11924,#12434,#6732,.T.);
#15593=EDGE_CURVE('',#11925,#12433,#6733,.T.);
#15594=EDGE_CURVE('',#12247,#12490,#6734,.T.);
#15595=EDGE_CURVE('',#11928,#12430,#6735,.T.);
#15596=EDGE_CURVE('',#12150,#12492,#6736,.T.);
#15597=EDGE_CURVE('',#12151,#12491,#6737,.T.);
#15598=EDGE_CURVE('',#11932,#12428,#6738,.T.);
#15599=EDGE_CURVE('',#11933,#12427,#6739,.T.);
#15600=EDGE_CURVE('',#11934,#12426,#6740,.T.);
#15601=EDGE_CURVE('',#11935,#12425,#6741,.T.);
#15602=EDGE_CURVE('',#11936,#12424,#6742,.T.);
#15603=EDGE_CURVE('',#11937,#12423,#6743,.T.);
#15604=EDGE_CURVE('',#11938,#12422,#6744,.T.);
#15605=EDGE_CURVE('',#11939,#12421,#6745,.T.);
#15606=EDGE_CURVE('',#11940,#12420,#6746,.T.);
#15607=EDGE_CURVE('',#11941,#12419,#6747,.T.);
#15608=EDGE_CURVE('',#11942,#12418,#6748,.T.);
#15609=EDGE_CURVE('',#11943,#12417,#6749,.T.);
#15610=EDGE_CURVE('',#11944,#12416,#6750,.T.);
#15611=EDGE_CURVE('',#11945,#12415,#6751,.T.);
#15612=EDGE_CURVE('',#12240,#12493,#6752,.T.);
#15613=EDGE_CURVE('',#11948,#12412,#6753,.T.);
#15614=EDGE_CURVE('',#12142,#12495,#6754,.T.);
#15615=EDGE_CURVE('',#12143,#12494,#6755,.T.);
#15616=EDGE_CURVE('',#11952,#12410,#6756,.T.);
#15617=EDGE_CURVE('',#11953,#12409,#6757,.T.);
#15618=EDGE_CURVE('',#11954,#12408,#6758,.T.);
#15619=EDGE_CURVE('',#11955,#12407,#6759,.T.);
#15620=EDGE_CURVE('',#11956,#12406,#6760,.T.);
#15621=EDGE_CURVE('',#11957,#12405,#6761,.T.);
#15622=EDGE_CURVE('',#11958,#12404,#6762,.T.);
#15623=EDGE_CURVE('',#11959,#12403,#6763,.T.);
#15624=EDGE_CURVE('',#11960,#12402,#6764,.T.);
#15625=EDGE_CURVE('',#11961,#12401,#6765,.T.);
#15626=EDGE_CURVE('',#11962,#12400,#6766,.T.);
#15627=EDGE_CURVE('',#11963,#12399,#6767,.T.);
#15628=EDGE_CURVE('',#11964,#12398,#6768,.T.);
#15629=EDGE_CURVE('',#11965,#12397,#6769,.T.);
#15630=EDGE_CURVE('',#12233,#12496,#6770,.T.);
#15631=EDGE_CURVE('',#11968,#12394,#6771,.T.);
#15632=EDGE_CURVE('',#12134,#12498,#6772,.T.);
#15633=EDGE_CURVE('',#12135,#12497,#6773,.T.);
#15634=EDGE_CURVE('',#11972,#12392,#6774,.T.);
#15635=EDGE_CURVE('',#11973,#12391,#6775,.T.);
#15636=EDGE_CURVE('',#11974,#12390,#6776,.T.);
#15637=EDGE_CURVE('',#11975,#12389,#6777,.T.);
#15638=EDGE_CURVE('',#11976,#12388,#6778,.T.);
#15639=EDGE_CURVE('',#11977,#12387,#6779,.T.);
#15640=EDGE_CURVE('',#11978,#12386,#6780,.T.);
#15641=EDGE_CURVE('',#11979,#12385,#6781,.T.);
#15642=EDGE_CURVE('',#11980,#12384,#6782,.T.);
#15643=EDGE_CURVE('',#11981,#12383,#6783,.T.);
#15644=EDGE_CURVE('',#11982,#12382,#6784,.T.);
#15645=EDGE_CURVE('',#11983,#12381,#6785,.T.);
#15646=EDGE_CURVE('',#11984,#12380,#6786,.T.);
#15647=EDGE_CURVE('',#11985,#12379,#6787,.T.);
#15648=EDGE_CURVE('',#12226,#12499,#6788,.T.);
#15649=EDGE_CURVE('',#11988,#12376,#6789,.T.);
#15650=EDGE_CURVE('',#12126,#12501,#6790,.T.);
#15651=EDGE_CURVE('',#12127,#12500,#6791,.T.);
#15652=EDGE_CURVE('',#11992,#12374,#6792,.T.);
#15653=EDGE_CURVE('',#11993,#12373,#6793,.T.);
#15654=EDGE_CURVE('',#11994,#12372,#6794,.T.);
#15655=EDGE_CURVE('',#11995,#12371,#6795,.T.);
#15656=EDGE_CURVE('',#11996,#12370,#6796,.T.);
#15657=EDGE_CURVE('',#11997,#12369,#6797,.T.);
#15658=EDGE_CURVE('',#11998,#12368,#6798,.T.);
#15659=EDGE_CURVE('',#11999,#12367,#6799,.T.);
#15660=EDGE_CURVE('',#12000,#12366,#6800,.T.);
#15661=EDGE_CURVE('',#12001,#12365,#6801,.T.);
#15662=EDGE_CURVE('',#12002,#12364,#6802,.T.);
#15663=EDGE_CURVE('',#12003,#12363,#6803,.T.);
#15664=EDGE_CURVE('',#12004,#12362,#6804,.T.);
#15665=EDGE_CURVE('',#12005,#12361,#6805,.T.);
#15666=EDGE_CURVE('',#12219,#12502,#6806,.T.);
#15667=EDGE_CURVE('',#12008,#12358,#6807,.T.);
#15668=EDGE_CURVE('',#12118,#12504,#6808,.T.);
#15669=EDGE_CURVE('',#12119,#12503,#6809,.T.);
#15670=EDGE_CURVE('',#12012,#12356,#6810,.T.);
#15671=EDGE_CURVE('',#12013,#12355,#6811,.T.);
#15672=EDGE_CURVE('',#12014,#12354,#6812,.T.);
#15673=EDGE_CURVE('',#12015,#12353,#6813,.T.);
#15674=EDGE_CURVE('',#12016,#12352,#6814,.T.);
#15675=EDGE_CURVE('',#12017,#12351,#6815,.T.);
#15676=EDGE_CURVE('',#12018,#12350,#6816,.T.);
#15677=EDGE_CURVE('',#12019,#12349,#6817,.T.);
#15678=EDGE_CURVE('',#12020,#12348,#6818,.T.);
#15679=EDGE_CURVE('',#12021,#12347,#6819,.T.);
#15680=EDGE_CURVE('',#12022,#12346,#6820,.T.);
#15681=EDGE_CURVE('',#12023,#12345,#6821,.T.);
#15682=EDGE_CURVE('',#12024,#12344,#6822,.T.);
#15683=EDGE_CURVE('',#12025,#12343,#6823,.T.);
#15684=EDGE_CURVE('',#12212,#12505,#6824,.T.);
#15685=EDGE_CURVE('',#12028,#12340,#6825,.T.);
#15686=EDGE_CURVE('',#12110,#12507,#6826,.T.);
#15687=EDGE_CURVE('',#12111,#12506,#6827,.T.);
#15688=EDGE_CURVE('',#12032,#12338,#6828,.T.);
#15689=EDGE_CURVE('',#12033,#12337,#6829,.T.);
#15690=EDGE_CURVE('',#12034,#12336,#6830,.T.);
#15691=EDGE_CURVE('',#12035,#12335,#6831,.T.);
#15692=EDGE_CURVE('',#12036,#12334,#6832,.T.);
#15693=EDGE_CURVE('',#12037,#12333,#6833,.T.);
#15694=EDGE_CURVE('',#12038,#12332,#6834,.T.);
#15695=EDGE_CURVE('',#12039,#12331,#6835,.T.);
#15696=EDGE_CURVE('',#12040,#12330,#6836,.T.);
#15697=EDGE_CURVE('',#12041,#12329,#6837,.T.);
#15698=EDGE_CURVE('',#12042,#12328,#6838,.T.);
#15699=EDGE_CURVE('',#12043,#12327,#6839,.T.);
#15700=EDGE_CURVE('',#12044,#12326,#6840,.T.);
#15701=EDGE_CURVE('',#12045,#12325,#6841,.T.);
#15702=EDGE_CURVE('',#12205,#12508,#6842,.T.);
#15703=EDGE_CURVE('',#12048,#12322,#6843,.T.);
#15704=EDGE_CURVE('',#12102,#12510,#6844,.T.);
#15705=EDGE_CURVE('',#12103,#12509,#6845,.T.);
#15706=EDGE_CURVE('',#12052,#12320,#6846,.T.);
#15707=EDGE_CURVE('',#12053,#12319,#6847,.T.);
#15708=EDGE_CURVE('',#12054,#12318,#6848,.T.);
#15709=EDGE_CURVE('',#12055,#12317,#6849,.T.);
#15710=EDGE_CURVE('',#12056,#12316,#6850,.T.);
#15711=EDGE_CURVE('',#12057,#12315,#6851,.T.);
#15712=EDGE_CURVE('',#12058,#12314,#6852,.T.);
#15713=EDGE_CURVE('',#12059,#12313,#6853,.T.);
#15714=EDGE_CURVE('',#12060,#12312,#6854,.T.);
#15715=EDGE_CURVE('',#12061,#12311,#6855,.T.);
#15716=EDGE_CURVE('',#12062,#12310,#6856,.T.);
#15717=EDGE_CURVE('',#12063,#12309,#6857,.T.);
#15718=EDGE_CURVE('',#12064,#12308,#6858,.T.);
#15719=EDGE_CURVE('',#12065,#12307,#6859,.T.);
#15720=EDGE_CURVE('',#12198,#12511,#6860,.T.);
#15721=EDGE_CURVE('',#12068,#12304,#6861,.T.);
#15722=EDGE_CURVE('',#12094,#12513,#6862,.T.);
#15723=EDGE_CURVE('',#12095,#12512,#6863,.T.);
#15724=EDGE_CURVE('',#12072,#12302,#6864,.T.);
#15725=EDGE_CURVE('',#12073,#12301,#6865,.T.);
#15726=EDGE_CURVE('',#12074,#12300,#6866,.T.);
#15727=EDGE_CURVE('',#12075,#12299,#6867,.T.);
#15728=EDGE_CURVE('',#12076,#12298,#6868,.T.);
#15729=EDGE_CURVE('',#12077,#12297,#6869,.T.);
#15730=EDGE_CURVE('',#12078,#12296,#6870,.T.);
#15731=EDGE_CURVE('',#12079,#12295,#6871,.T.);
#15732=EDGE_CURVE('',#12080,#12294,#6872,.T.);
#15733=EDGE_CURVE('',#12081,#12293,#6873,.T.);
#15734=EDGE_CURVE('',#12082,#12292,#6874,.T.);
#15735=EDGE_CURVE('',#12083,#12291,#6875,.T.);
#15736=EDGE_CURVE('',#12084,#12290,#6876,.T.);
#15737=EDGE_CURVE('',#12085,#12289,#6877,.T.);
#15738=EDGE_CURVE('',#12191,#12514,#6878,.T.);
#15739=EDGE_CURVE('',#11850,#12286,#6879,.T.);
#15740=EDGE_CURVE('',#11847,#12516,#6880,.T.);
#15741=EDGE_CURVE('',#11848,#12515,#6881,.T.);
#15742=EDGE_CURVE('',#11852,#12284,#6882,.T.);
#15743=EDGE_CURVE('',#11853,#12283,#6883,.T.);
#15744=EDGE_CURVE('',#11854,#12282,#6884,.T.);
#15745=EDGE_CURVE('',#11855,#12281,#6885,.T.);
#15746=EDGE_CURVE('',#11856,#12280,#6886,.T.);
#15747=EDGE_CURVE('',#11857,#12279,#6887,.T.);
#15748=EDGE_CURVE('',#11858,#12278,#6888,.T.);
#15749=EDGE_CURVE('',#11859,#12277,#6889,.T.);
#15750=EDGE_CURVE('',#11860,#12276,#6890,.T.);
#15751=EDGE_CURVE('',#11861,#12275,#6891,.T.);
#15752=EDGE_CURVE('',#11862,#12274,#6892,.T.);
#15753=EDGE_CURVE('',#11863,#12273,#6893,.T.);
#15754=EDGE_CURVE('',#11864,#12272,#6894,.T.);
#15755=EDGE_CURVE('',#11865,#12271,#6895,.T.);
#15756=EDGE_CURVE('',#12184,#12517,#6896,.T.);
#15757=EDGE_CURVE('',#12088,#12518,#6897,.T.);
#15758=EDGE_CURVE('',#12518,#12518,#10579,.T.);
#15759=EDGE_CURVE('',#12519,#12519,#10580,.T.);
#15760=EDGE_CURVE('',#12519,#12483,#6898,.T.);
#19988=ORIENTED_EDGE('',*,*,#14747,.T.);
#19989=ORIENTED_EDGE('',*,*,#14748,.T.);
#19990=ORIENTED_EDGE('',*,*,#14749,.T.);
#19991=ORIENTED_EDGE('',*,*,#14750,.T.);
#19992=ORIENTED_EDGE('',*,*,#14751,.T.);
#19993=ORIENTED_EDGE('',*,*,#14752,.T.);
#19994=ORIENTED_EDGE('',*,*,#14753,.T.);
#19995=ORIENTED_EDGE('',*,*,#14748,.F.);
#19996=ORIENTED_EDGE('',*,*,#14754,.T.);
#19997=ORIENTED_EDGE('',*,*,#14755,.T.);
#19998=ORIENTED_EDGE('',*,*,#14756,.T.);
#19999=ORIENTED_EDGE('',*,*,#14757,.T.);
#20000=ORIENTED_EDGE('',*,*,#14758,.T.);
#20001=ORIENTED_EDGE('',*,*,#14759,.T.);
#20002=ORIENTED_EDGE('',*,*,#14760,.T.);
#20003=ORIENTED_EDGE('',*,*,#14761,.T.);
#20004=ORIENTED_EDGE('',*,*,#14762,.T.);
#20005=ORIENTED_EDGE('',*,*,#14763,.T.);
#20006=ORIENTED_EDGE('',*,*,#14764,.T.);
#20007=ORIENTED_EDGE('',*,*,#14765,.T.);
#20008=ORIENTED_EDGE('',*,*,#14766,.T.);
#20009=ORIENTED_EDGE('',*,*,#14767,.T.);
#20010=ORIENTED_EDGE('',*,*,#14768,.T.);
#20011=ORIENTED_EDGE('',*,*,#14769,.T.);
#20012=ORIENTED_EDGE('',*,*,#14770,.F.);
#20013=ORIENTED_EDGE('',*,*,#14771,.T.);
#20014=ORIENTED_EDGE('',*,*,#14772,.T.);
#20015=ORIENTED_EDGE('',*,*,#14773,.F.);
#20016=ORIENTED_EDGE('',*,*,#14774,.T.);
#20017=ORIENTED_EDGE('',*,*,#14775,.T.);
#20018=ORIENTED_EDGE('',*,*,#14776,.T.);
#20019=ORIENTED_EDGE('',*,*,#14777,.T.);
#20020=ORIENTED_EDGE('',*,*,#14778,.T.);
#20021=ORIENTED_EDGE('',*,*,#14779,.T.);
#20022=ORIENTED_EDGE('',*,*,#14780,.T.);
#20023=ORIENTED_EDGE('',*,*,#14781,.T.);
#20024=ORIENTED_EDGE('',*,*,#14782,.T.);
#20025=ORIENTED_EDGE('',*,*,#14783,.T.);
#20026=ORIENTED_EDGE('',*,*,#14784,.T.);
#20027=ORIENTED_EDGE('',*,*,#14785,.T.);
#20028=ORIENTED_EDGE('',*,*,#14786,.T.);
#20029=ORIENTED_EDGE('',*,*,#14787,.T.);
#20030=ORIENTED_EDGE('',*,*,#14788,.T.);
#20031=ORIENTED_EDGE('',*,*,#14789,.T.);
#20032=ORIENTED_EDGE('',*,*,#14790,.F.);
#20033=ORIENTED_EDGE('',*,*,#14791,.T.);
#20034=ORIENTED_EDGE('',*,*,#14792,.T.);
#20035=ORIENTED_EDGE('',*,*,#14793,.F.);
#20036=ORIENTED_EDGE('',*,*,#14794,.T.);
#20037=ORIENTED_EDGE('',*,*,#14795,.T.);
#20038=ORIENTED_EDGE('',*,*,#14796,.T.);
#20039=ORIENTED_EDGE('',*,*,#14797,.T.);
#20040=ORIENTED_EDGE('',*,*,#14798,.T.);
#20041=ORIENTED_EDGE('',*,*,#14799,.T.);
#20042=ORIENTED_EDGE('',*,*,#14800,.T.);
#20043=ORIENTED_EDGE('',*,*,#14801,.T.);
#20044=ORIENTED_EDGE('',*,*,#14802,.T.);
#20045=ORIENTED_EDGE('',*,*,#14803,.T.);
#20046=ORIENTED_EDGE('',*,*,#14804,.T.);
#20047=ORIENTED_EDGE('',*,*,#14805,.T.);
#20048=ORIENTED_EDGE('',*,*,#14806,.T.);
#20049=ORIENTED_EDGE('',*,*,#14807,.T.);
#20050=ORIENTED_EDGE('',*,*,#14808,.T.);
#20051=ORIENTED_EDGE('',*,*,#14809,.T.);
#20052=ORIENTED_EDGE('',*,*,#14810,.F.);
#20053=ORIENTED_EDGE('',*,*,#14811,.T.);
#20054=ORIENTED_EDGE('',*,*,#14812,.T.);
#20055=ORIENTED_EDGE('',*,*,#14813,.F.);
#20056=ORIENTED_EDGE('',*,*,#14814,.T.);
#20057=ORIENTED_EDGE('',*,*,#14815,.T.);
#20058=ORIENTED_EDGE('',*,*,#14816,.T.);
#20059=ORIENTED_EDGE('',*,*,#14817,.T.);
#20060=ORIENTED_EDGE('',*,*,#14818,.T.);
#20061=ORIENTED_EDGE('',*,*,#14819,.T.);
#20062=ORIENTED_EDGE('',*,*,#14820,.T.);
#20063=ORIENTED_EDGE('',*,*,#14821,.T.);
#20064=ORIENTED_EDGE('',*,*,#14822,.T.);
#20065=ORIENTED_EDGE('',*,*,#14823,.T.);
#20066=ORIENTED_EDGE('',*,*,#14824,.T.);
#20067=ORIENTED_EDGE('',*,*,#14825,.T.);
#20068=ORIENTED_EDGE('',*,*,#14826,.T.);
#20069=ORIENTED_EDGE('',*,*,#14827,.T.);
#20070=ORIENTED_EDGE('',*,*,#14828,.T.);
#20071=ORIENTED_EDGE('',*,*,#14829,.T.);
#20072=ORIENTED_EDGE('',*,*,#14830,.F.);
#20073=ORIENTED_EDGE('',*,*,#14831,.T.);
#20074=ORIENTED_EDGE('',*,*,#14832,.T.);
#20075=ORIENTED_EDGE('',*,*,#14833,.F.);
#20076=ORIENTED_EDGE('',*,*,#14834,.T.);
#20077=ORIENTED_EDGE('',*,*,#14835,.T.);
#20078=ORIENTED_EDGE('',*,*,#14836,.T.);
#20079=ORIENTED_EDGE('',*,*,#14837,.T.);
#20080=ORIENTED_EDGE('',*,*,#14838,.T.);
#20081=ORIENTED_EDGE('',*,*,#14839,.T.);
#20082=ORIENTED_EDGE('',*,*,#14840,.T.);
#20083=ORIENTED_EDGE('',*,*,#14841,.T.);
#20084=ORIENTED_EDGE('',*,*,#14842,.T.);
#20085=ORIENTED_EDGE('',*,*,#14843,.T.);
#20086=ORIENTED_EDGE('',*,*,#14844,.T.);
#20087=ORIENTED_EDGE('',*,*,#14845,.T.);
#20088=ORIENTED_EDGE('',*,*,#14846,.T.);
#20089=ORIENTED_EDGE('',*,*,#14847,.T.);
#20090=ORIENTED_EDGE('',*,*,#14848,.T.);
#20091=ORIENTED_EDGE('',*,*,#14849,.T.);
#20092=ORIENTED_EDGE('',*,*,#14850,.F.);
#20093=ORIENTED_EDGE('',*,*,#14851,.T.);
#20094=ORIENTED_EDGE('',*,*,#14852,.T.);
#20095=ORIENTED_EDGE('',*,*,#14853,.F.);
#20096=ORIENTED_EDGE('',*,*,#14854,.T.);
#20097=ORIENTED_EDGE('',*,*,#14855,.T.);
#20098=ORIENTED_EDGE('',*,*,#14856,.T.);
#20099=ORIENTED_EDGE('',*,*,#14857,.T.);
#20100=ORIENTED_EDGE('',*,*,#14858,.T.);
#20101=ORIENTED_EDGE('',*,*,#14859,.T.);
#20102=ORIENTED_EDGE('',*,*,#14860,.T.);
#20103=ORIENTED_EDGE('',*,*,#14861,.T.);
#20104=ORIENTED_EDGE('',*,*,#14862,.T.);
#20105=ORIENTED_EDGE('',*,*,#14863,.T.);
#20106=ORIENTED_EDGE('',*,*,#14864,.T.);
#20107=ORIENTED_EDGE('',*,*,#14865,.T.);
#20108=ORIENTED_EDGE('',*,*,#14866,.T.);
#20109=ORIENTED_EDGE('',*,*,#14867,.T.);
#20110=ORIENTED_EDGE('',*,*,#14868,.T.);
#20111=ORIENTED_EDGE('',*,*,#14869,.T.);
#20112=ORIENTED_EDGE('',*,*,#14870,.F.);
#20113=ORIENTED_EDGE('',*,*,#14871,.T.);
#20114=ORIENTED_EDGE('',*,*,#14872,.T.);
#20115=ORIENTED_EDGE('',*,*,#14873,.F.);
#20116=ORIENTED_EDGE('',*,*,#14874,.T.);
#20117=ORIENTED_EDGE('',*,*,#14875,.T.);
#20118=ORIENTED_EDGE('',*,*,#14876,.T.);
#20119=ORIENTED_EDGE('',*,*,#14877,.T.);
#20120=ORIENTED_EDGE('',*,*,#14878,.T.);
#20121=ORIENTED_EDGE('',*,*,#14879,.T.);
#20122=ORIENTED_EDGE('',*,*,#14880,.T.);
#20123=ORIENTED_EDGE('',*,*,#14881,.T.);
#20124=ORIENTED_EDGE('',*,*,#14882,.T.);
#20125=ORIENTED_EDGE('',*,*,#14883,.T.);
#20126=ORIENTED_EDGE('',*,*,#14884,.T.);
#20127=ORIENTED_EDGE('',*,*,#14885,.T.);
#20128=ORIENTED_EDGE('',*,*,#14886,.T.);
#20129=ORIENTED_EDGE('',*,*,#14887,.T.);
#20130=ORIENTED_EDGE('',*,*,#14888,.T.);
#20131=ORIENTED_EDGE('',*,*,#14889,.T.);
#20132=ORIENTED_EDGE('',*,*,#14890,.F.);
#20133=ORIENTED_EDGE('',*,*,#14891,.T.);
#20134=ORIENTED_EDGE('',*,*,#14892,.T.);
#20135=ORIENTED_EDGE('',*,*,#14893,.F.);
#20136=ORIENTED_EDGE('',*,*,#14894,.T.);
#20137=ORIENTED_EDGE('',*,*,#14895,.T.);
#20138=ORIENTED_EDGE('',*,*,#14896,.T.);
#20139=ORIENTED_EDGE('',*,*,#14897,.T.);
#20140=ORIENTED_EDGE('',*,*,#14898,.T.);
#20141=ORIENTED_EDGE('',*,*,#14899,.T.);
#20142=ORIENTED_EDGE('',*,*,#14900,.T.);
#20143=ORIENTED_EDGE('',*,*,#14901,.T.);
#20144=ORIENTED_EDGE('',*,*,#14902,.T.);
#20145=ORIENTED_EDGE('',*,*,#14903,.T.);
#20146=ORIENTED_EDGE('',*,*,#14904,.T.);
#20147=ORIENTED_EDGE('',*,*,#14905,.T.);
#20148=ORIENTED_EDGE('',*,*,#14906,.T.);
#20149=ORIENTED_EDGE('',*,*,#14907,.T.);
#20150=ORIENTED_EDGE('',*,*,#14908,.T.);
#20151=ORIENTED_EDGE('',*,*,#14909,.T.);
#20152=ORIENTED_EDGE('',*,*,#14910,.F.);
#20153=ORIENTED_EDGE('',*,*,#14911,.T.);
#20154=ORIENTED_EDGE('',*,*,#14912,.T.);
#20155=ORIENTED_EDGE('',*,*,#14913,.F.);
#20156=ORIENTED_EDGE('',*,*,#14914,.T.);
#20157=ORIENTED_EDGE('',*,*,#14915,.T.);
#20158=ORIENTED_EDGE('',*,*,#14916,.T.);
#20159=ORIENTED_EDGE('',*,*,#14917,.T.);
#20160=ORIENTED_EDGE('',*,*,#14918,.T.);
#20161=ORIENTED_EDGE('',*,*,#14919,.T.);
#20162=ORIENTED_EDGE('',*,*,#14920,.T.);
#20163=ORIENTED_EDGE('',*,*,#14921,.T.);
#20164=ORIENTED_EDGE('',*,*,#14922,.T.);
#20165=ORIENTED_EDGE('',*,*,#14923,.T.);
#20166=ORIENTED_EDGE('',*,*,#14924,.T.);
#20167=ORIENTED_EDGE('',*,*,#14925,.T.);
#20168=ORIENTED_EDGE('',*,*,#14926,.T.);
#20169=ORIENTED_EDGE('',*,*,#14927,.T.);
#20170=ORIENTED_EDGE('',*,*,#14928,.T.);
#20171=ORIENTED_EDGE('',*,*,#14929,.T.);
#20172=ORIENTED_EDGE('',*,*,#14930,.F.);
#20173=ORIENTED_EDGE('',*,*,#14931,.T.);
#20174=ORIENTED_EDGE('',*,*,#14932,.T.);
#20175=ORIENTED_EDGE('',*,*,#14933,.F.);
#20176=ORIENTED_EDGE('',*,*,#14934,.T.);
#20177=ORIENTED_EDGE('',*,*,#14935,.T.);
#20178=ORIENTED_EDGE('',*,*,#14936,.T.);
#20179=ORIENTED_EDGE('',*,*,#14937,.T.);
#20180=ORIENTED_EDGE('',*,*,#14938,.T.);
#20181=ORIENTED_EDGE('',*,*,#14939,.T.);
#20182=ORIENTED_EDGE('',*,*,#14940,.T.);
#20183=ORIENTED_EDGE('',*,*,#14941,.T.);
#20184=ORIENTED_EDGE('',*,*,#14942,.T.);
#20185=ORIENTED_EDGE('',*,*,#14943,.T.);
#20186=ORIENTED_EDGE('',*,*,#14944,.T.);
#20187=ORIENTED_EDGE('',*,*,#14945,.T.);
#20188=ORIENTED_EDGE('',*,*,#14946,.T.);
#20189=ORIENTED_EDGE('',*,*,#14947,.T.);
#20190=ORIENTED_EDGE('',*,*,#14948,.T.);
#20191=ORIENTED_EDGE('',*,*,#14949,.T.);
#20192=ORIENTED_EDGE('',*,*,#14950,.F.);
#20193=ORIENTED_EDGE('',*,*,#14951,.T.);
#20194=ORIENTED_EDGE('',*,*,#14952,.T.);
#20195=ORIENTED_EDGE('',*,*,#14953,.F.);
#20196=ORIENTED_EDGE('',*,*,#14954,.T.);
#20197=ORIENTED_EDGE('',*,*,#14955,.T.);
#20198=ORIENTED_EDGE('',*,*,#14956,.T.);
#20199=ORIENTED_EDGE('',*,*,#14957,.T.);
#20200=ORIENTED_EDGE('',*,*,#14958,.T.);
#20201=ORIENTED_EDGE('',*,*,#14959,.T.);
#20202=ORIENTED_EDGE('',*,*,#14960,.T.);
#20203=ORIENTED_EDGE('',*,*,#14961,.T.);
#20204=ORIENTED_EDGE('',*,*,#14962,.T.);
#20205=ORIENTED_EDGE('',*,*,#14963,.T.);
#20206=ORIENTED_EDGE('',*,*,#14964,.T.);
#20207=ORIENTED_EDGE('',*,*,#14965,.T.);
#20208=ORIENTED_EDGE('',*,*,#14966,.T.);
#20209=ORIENTED_EDGE('',*,*,#14967,.T.);
#20210=ORIENTED_EDGE('',*,*,#14968,.T.);
#20211=ORIENTED_EDGE('',*,*,#14969,.T.);
#20212=ORIENTED_EDGE('',*,*,#14970,.F.);
#20213=ORIENTED_EDGE('',*,*,#14971,.T.);
#20214=ORIENTED_EDGE('',*,*,#14972,.T.);
#20215=ORIENTED_EDGE('',*,*,#14973,.F.);
#20216=ORIENTED_EDGE('',*,*,#14974,.T.);
#20217=ORIENTED_EDGE('',*,*,#14975,.T.);
#20218=ORIENTED_EDGE('',*,*,#14976,.T.);
#20219=ORIENTED_EDGE('',*,*,#14977,.T.);
#20220=ORIENTED_EDGE('',*,*,#14978,.T.);
#20221=ORIENTED_EDGE('',*,*,#14979,.T.);
#20222=ORIENTED_EDGE('',*,*,#14980,.T.);
#20223=ORIENTED_EDGE('',*,*,#14981,.T.);
#20224=ORIENTED_EDGE('',*,*,#14982,.T.);
#20225=ORIENTED_EDGE('',*,*,#14983,.T.);
#20226=ORIENTED_EDGE('',*,*,#14984,.T.);
#20227=ORIENTED_EDGE('',*,*,#14985,.T.);
#20228=ORIENTED_EDGE('',*,*,#14986,.T.);
#20229=ORIENTED_EDGE('',*,*,#14987,.T.);
#20230=ORIENTED_EDGE('',*,*,#14988,.T.);
#20231=ORIENTED_EDGE('',*,*,#14989,.T.);
#20232=ORIENTED_EDGE('',*,*,#14990,.F.);
#20233=ORIENTED_EDGE('',*,*,#14991,.T.);
#20234=ORIENTED_EDGE('',*,*,#14992,.F.);
#20235=ORIENTED_EDGE('',*,*,#14747,.F.);
#20236=ORIENTED_EDGE('',*,*,#14993,.T.);
#20237=ORIENTED_EDGE('',*,*,#14994,.F.);
#20238=ORIENTED_EDGE('',*,*,#14995,.F.);
#20239=ORIENTED_EDGE('',*,*,#14996,.F.);
#20240=ORIENTED_EDGE('',*,*,#14754,.F.);
#20241=ORIENTED_EDGE('',*,*,#14752,.F.);
#20242=ORIENTED_EDGE('',*,*,#14997,.T.);
#20243=ORIENTED_EDGE('',*,*,#14998,.F.);
#20244=ORIENTED_EDGE('',*,*,#14993,.F.);
#20245=ORIENTED_EDGE('',*,*,#14999,.T.);
#20246=ORIENTED_EDGE('',*,*,#14973,.T.);
#20247=ORIENTED_EDGE('',*,*,#15000,.T.);
#20248=ORIENTED_EDGE('',*,*,#15001,.T.);
#20249=ORIENTED_EDGE('',*,*,#15002,.T.);
#20250=ORIENTED_EDGE('',*,*,#15003,.T.);
#20251=ORIENTED_EDGE('',*,*,#14999,.F.);
#20252=ORIENTED_EDGE('',*,*,#15004,.T.);
#20253=ORIENTED_EDGE('',*,*,#15005,.F.);
#20254=ORIENTED_EDGE('',*,*,#15006,.F.);
#20255=ORIENTED_EDGE('',*,*,#15007,.F.);
#20256=ORIENTED_EDGE('',*,*,#14974,.F.);
#20257=ORIENTED_EDGE('',*,*,#15003,.F.);
#20258=ORIENTED_EDGE('',*,*,#15008,.T.);
#20259=ORIENTED_EDGE('',*,*,#15009,.F.);
#20260=ORIENTED_EDGE('',*,*,#15004,.F.);
#20261=ORIENTED_EDGE('',*,*,#15010,.T.);
#20262=ORIENTED_EDGE('',*,*,#14953,.T.);
#20263=ORIENTED_EDGE('',*,*,#15011,.T.);
#20264=ORIENTED_EDGE('',*,*,#15012,.T.);
#20265=ORIENTED_EDGE('',*,*,#15013,.T.);
#20266=ORIENTED_EDGE('',*,*,#15014,.T.);
#20267=ORIENTED_EDGE('',*,*,#15010,.F.);
#20268=ORIENTED_EDGE('',*,*,#15015,.T.);
#20269=ORIENTED_EDGE('',*,*,#15016,.F.);
#20270=ORIENTED_EDGE('',*,*,#15017,.F.);
#20271=ORIENTED_EDGE('',*,*,#15018,.F.);
#20272=ORIENTED_EDGE('',*,*,#14954,.F.);
#20273=ORIENTED_EDGE('',*,*,#15014,.F.);
#20274=ORIENTED_EDGE('',*,*,#15019,.T.);
#20275=ORIENTED_EDGE('',*,*,#15020,.F.);
#20276=ORIENTED_EDGE('',*,*,#15015,.F.);
#20277=ORIENTED_EDGE('',*,*,#15021,.T.);
#20278=ORIENTED_EDGE('',*,*,#14933,.T.);
#20279=ORIENTED_EDGE('',*,*,#15022,.T.);
#20280=ORIENTED_EDGE('',*,*,#15023,.T.);
#20281=ORIENTED_EDGE('',*,*,#15024,.T.);
#20282=ORIENTED_EDGE('',*,*,#15025,.T.);
#20283=ORIENTED_EDGE('',*,*,#15021,.F.);
#20284=ORIENTED_EDGE('',*,*,#15026,.T.);
#20285=ORIENTED_EDGE('',*,*,#15027,.F.);
#20286=ORIENTED_EDGE('',*,*,#15028,.F.);
#20287=ORIENTED_EDGE('',*,*,#15029,.F.);
#20288=ORIENTED_EDGE('',*,*,#14934,.F.);
#20289=ORIENTED_EDGE('',*,*,#15025,.F.);
#20290=ORIENTED_EDGE('',*,*,#15030,.T.);
#20291=ORIENTED_EDGE('',*,*,#15031,.F.);
#20292=ORIENTED_EDGE('',*,*,#15026,.F.);
#20293=ORIENTED_EDGE('',*,*,#15032,.T.);
#20294=ORIENTED_EDGE('',*,*,#14913,.T.);
#20295=ORIENTED_EDGE('',*,*,#15033,.T.);
#20296=ORIENTED_EDGE('',*,*,#15034,.T.);
#20297=ORIENTED_EDGE('',*,*,#15035,.T.);
#20298=ORIENTED_EDGE('',*,*,#15036,.T.);
#20299=ORIENTED_EDGE('',*,*,#15032,.F.);
#20300=ORIENTED_EDGE('',*,*,#15037,.T.);
#20301=ORIENTED_EDGE('',*,*,#15038,.F.);
#20302=ORIENTED_EDGE('',*,*,#15039,.F.);
#20303=ORIENTED_EDGE('',*,*,#15040,.F.);
#20304=ORIENTED_EDGE('',*,*,#14914,.F.);
#20305=ORIENTED_EDGE('',*,*,#15036,.F.);
#20306=ORIENTED_EDGE('',*,*,#15041,.T.);
#20307=ORIENTED_EDGE('',*,*,#15042,.F.);
#20308=ORIENTED_EDGE('',*,*,#15037,.F.);
#20309=ORIENTED_EDGE('',*,*,#15043,.T.);
#20310=ORIENTED_EDGE('',*,*,#14893,.T.);
#20311=ORIENTED_EDGE('',*,*,#15044,.T.);
#20312=ORIENTED_EDGE('',*,*,#15045,.T.);
#20313=ORIENTED_EDGE('',*,*,#15046,.T.);
#20314=ORIENTED_EDGE('',*,*,#15047,.T.);
#20315=ORIENTED_EDGE('',*,*,#15043,.F.);
#20316=ORIENTED_EDGE('',*,*,#15048,.T.);
#20317=ORIENTED_EDGE('',*,*,#15049,.F.);
#20318=ORIENTED_EDGE('',*,*,#15050,.F.);
#20319=ORIENTED_EDGE('',*,*,#15051,.F.);
#20320=ORIENTED_EDGE('',*,*,#14894,.F.);
#20321=ORIENTED_EDGE('',*,*,#15047,.F.);
#20322=ORIENTED_EDGE('',*,*,#15052,.T.);
#20323=ORIENTED_EDGE('',*,*,#15053,.F.);
#20324=ORIENTED_EDGE('',*,*,#15048,.F.);
#20325=ORIENTED_EDGE('',*,*,#15054,.T.);
#20326=ORIENTED_EDGE('',*,*,#14873,.T.);
#20327=ORIENTED_EDGE('',*,*,#15055,.T.);
#20328=ORIENTED_EDGE('',*,*,#15056,.T.);
#20329=ORIENTED_EDGE('',*,*,#15057,.T.);
#20330=ORIENTED_EDGE('',*,*,#15058,.T.);
#20331=ORIENTED_EDGE('',*,*,#15054,.F.);
#20332=ORIENTED_EDGE('',*,*,#15059,.T.);
#20333=ORIENTED_EDGE('',*,*,#15060,.F.);
#20334=ORIENTED_EDGE('',*,*,#15061,.F.);
#20335=ORIENTED_EDGE('',*,*,#15062,.F.);
#20336=ORIENTED_EDGE('',*,*,#14874,.F.);
#20337=ORIENTED_EDGE('',*,*,#15058,.F.);
#20338=ORIENTED_EDGE('',*,*,#15063,.T.);
#20339=ORIENTED_EDGE('',*,*,#15064,.F.);
#20340=ORIENTED_EDGE('',*,*,#15059,.F.);
#20341=ORIENTED_EDGE('',*,*,#15065,.T.);
#20342=ORIENTED_EDGE('',*,*,#14853,.T.);
#20343=ORIENTED_EDGE('',*,*,#15066,.T.);
#20344=ORIENTED_EDGE('',*,*,#15067,.T.);
#20345=ORIENTED_EDGE('',*,*,#15068,.T.);
#20346=ORIENTED_EDGE('',*,*,#15069,.T.);
#20347=ORIENTED_EDGE('',*,*,#15065,.F.);
#20348=ORIENTED_EDGE('',*,*,#15070,.T.);
#20349=ORIENTED_EDGE('',*,*,#15071,.F.);
#20350=ORIENTED_EDGE('',*,*,#15072,.F.);
#20351=ORIENTED_EDGE('',*,*,#15073,.F.);
#20352=ORIENTED_EDGE('',*,*,#14854,.F.);
#20353=ORIENTED_EDGE('',*,*,#15069,.F.);
#20354=ORIENTED_EDGE('',*,*,#15074,.T.);
#20355=ORIENTED_EDGE('',*,*,#15075,.F.);
#20356=ORIENTED_EDGE('',*,*,#15070,.F.);
#20357=ORIENTED_EDGE('',*,*,#15076,.T.);
#20358=ORIENTED_EDGE('',*,*,#14833,.T.);
#20359=ORIENTED_EDGE('',*,*,#15077,.T.);
#20360=ORIENTED_EDGE('',*,*,#15078,.T.);
#20361=ORIENTED_EDGE('',*,*,#15079,.T.);
#20362=ORIENTED_EDGE('',*,*,#15080,.T.);
#20363=ORIENTED_EDGE('',*,*,#15076,.F.);
#20364=ORIENTED_EDGE('',*,*,#15081,.T.);
#20365=ORIENTED_EDGE('',*,*,#15082,.F.);
#20366=ORIENTED_EDGE('',*,*,#15083,.F.);
#20367=ORIENTED_EDGE('',*,*,#15084,.F.);
#20368=ORIENTED_EDGE('',*,*,#14834,.F.);
#20369=ORIENTED_EDGE('',*,*,#15080,.F.);
#20370=ORIENTED_EDGE('',*,*,#15085,.T.);
#20371=ORIENTED_EDGE('',*,*,#15086,.F.);
#20372=ORIENTED_EDGE('',*,*,#15081,.F.);
#20373=ORIENTED_EDGE('',*,*,#15087,.T.);
#20374=ORIENTED_EDGE('',*,*,#14813,.T.);
#20375=ORIENTED_EDGE('',*,*,#15088,.T.);
#20376=ORIENTED_EDGE('',*,*,#15089,.T.);
#20377=ORIENTED_EDGE('',*,*,#15090,.T.);
#20378=ORIENTED_EDGE('',*,*,#15091,.T.);
#20379=ORIENTED_EDGE('',*,*,#15087,.F.);
#20380=ORIENTED_EDGE('',*,*,#15092,.T.);
#20381=ORIENTED_EDGE('',*,*,#15093,.F.);
#20382=ORIENTED_EDGE('',*,*,#15094,.F.);
#20383=ORIENTED_EDGE('',*,*,#15095,.F.);
#20384=ORIENTED_EDGE('',*,*,#14814,.F.);
#20385=ORIENTED_EDGE('',*,*,#15091,.F.);
#20386=ORIENTED_EDGE('',*,*,#15096,.T.);
#20387=ORIENTED_EDGE('',*,*,#15097,.F.);
#20388=ORIENTED_EDGE('',*,*,#15092,.F.);
#20389=ORIENTED_EDGE('',*,*,#15098,.T.);
#20390=ORIENTED_EDGE('',*,*,#14793,.T.);
#20391=ORIENTED_EDGE('',*,*,#15099,.T.);
#20392=ORIENTED_EDGE('',*,*,#15100,.T.);
#20393=ORIENTED_EDGE('',*,*,#15101,.T.);
#20394=ORIENTED_EDGE('',*,*,#15102,.T.);
#20395=ORIENTED_EDGE('',*,*,#15098,.F.);
#20396=ORIENTED_EDGE('',*,*,#15103,.T.);
#20397=ORIENTED_EDGE('',*,*,#15104,.F.);
#20398=ORIENTED_EDGE('',*,*,#15105,.F.);
#20399=ORIENTED_EDGE('',*,*,#15106,.F.);
#20400=ORIENTED_EDGE('',*,*,#14794,.F.);
#20401=ORIENTED_EDGE('',*,*,#15102,.F.);
#20402=ORIENTED_EDGE('',*,*,#15107,.T.);
#20403=ORIENTED_EDGE('',*,*,#15108,.F.);
#20404=ORIENTED_EDGE('',*,*,#15103,.F.);
#20405=ORIENTED_EDGE('',*,*,#15109,.T.);
#20406=ORIENTED_EDGE('',*,*,#14773,.T.);
#20407=ORIENTED_EDGE('',*,*,#15110,.T.);
#20408=ORIENTED_EDGE('',*,*,#15111,.T.);
#20409=ORIENTED_EDGE('',*,*,#15112,.T.);
#20410=ORIENTED_EDGE('',*,*,#15113,.T.);
#20411=ORIENTED_EDGE('',*,*,#15109,.F.);
#20412=ORIENTED_EDGE('',*,*,#15114,.T.);
#20413=ORIENTED_EDGE('',*,*,#15115,.F.);
#20414=ORIENTED_EDGE('',*,*,#15116,.F.);
#20415=ORIENTED_EDGE('',*,*,#15117,.F.);
#20416=ORIENTED_EDGE('',*,*,#14774,.F.);
#20417=ORIENTED_EDGE('',*,*,#15113,.F.);
#20418=ORIENTED_EDGE('',*,*,#15118,.T.);
#20419=ORIENTED_EDGE('',*,*,#15119,.F.);
#20420=ORIENTED_EDGE('',*,*,#15114,.F.);
#20421=ORIENTED_EDGE('',*,*,#15120,.T.);
#20422=ORIENTED_EDGE('',*,*,#15121,.T.);
#20423=ORIENTED_EDGE('',*,*,#15122,.T.);
#20424=ORIENTED_EDGE('',*,*,#14770,.T.);
#20425=ORIENTED_EDGE('',*,*,#15123,.T.);
#20426=ORIENTED_EDGE('',*,*,#15124,.T.);
#20427=ORIENTED_EDGE('',*,*,#15121,.F.);
#20428=ORIENTED_EDGE('',*,*,#15125,.T.);
#20429=ORIENTED_EDGE('',*,*,#15126,.F.);
#20430=ORIENTED_EDGE('',*,*,#15127,.F.);
#20431=ORIENTED_EDGE('',*,*,#15120,.F.);
#20432=ORIENTED_EDGE('',*,*,#15128,.T.);
#20433=ORIENTED_EDGE('',*,*,#15129,.F.);
#20434=ORIENTED_EDGE('',*,*,#15125,.F.);
#20435=ORIENTED_EDGE('',*,*,#15130,.T.);
#20436=ORIENTED_EDGE('',*,*,#15131,.T.);
#20437=ORIENTED_EDGE('',*,*,#15132,.T.);
#20438=ORIENTED_EDGE('',*,*,#14990,.T.);
#20439=ORIENTED_EDGE('',*,*,#15133,.T.);
#20440=ORIENTED_EDGE('',*,*,#15134,.T.);
#20441=ORIENTED_EDGE('',*,*,#15131,.F.);
#20442=ORIENTED_EDGE('',*,*,#15135,.T.);
#20443=ORIENTED_EDGE('',*,*,#15136,.F.);
#20444=ORIENTED_EDGE('',*,*,#15137,.F.);
#20445=ORIENTED_EDGE('',*,*,#15130,.F.);
#20446=ORIENTED_EDGE('',*,*,#15138,.T.);
#20447=ORIENTED_EDGE('',*,*,#15139,.F.);
#20448=ORIENTED_EDGE('',*,*,#15135,.F.);
#20449=ORIENTED_EDGE('',*,*,#15140,.T.);
#20450=ORIENTED_EDGE('',*,*,#15141,.T.);
#20451=ORIENTED_EDGE('',*,*,#15142,.T.);
#20452=ORIENTED_EDGE('',*,*,#14970,.T.);
#20453=ORIENTED_EDGE('',*,*,#15143,.T.);
#20454=ORIENTED_EDGE('',*,*,#15144,.T.);
#20455=ORIENTED_EDGE('',*,*,#15141,.F.);
#20456=ORIENTED_EDGE('',*,*,#15145,.T.);
#20457=ORIENTED_EDGE('',*,*,#15146,.F.);
#20458=ORIENTED_EDGE('',*,*,#15147,.F.);
#20459=ORIENTED_EDGE('',*,*,#15140,.F.);
#20460=ORIENTED_EDGE('',*,*,#15148,.T.);
#20461=ORIENTED_EDGE('',*,*,#15149,.F.);
#20462=ORIENTED_EDGE('',*,*,#15145,.F.);
#20463=ORIENTED_EDGE('',*,*,#15150,.T.);
#20464=ORIENTED_EDGE('',*,*,#15151,.T.);
#20465=ORIENTED_EDGE('',*,*,#15152,.T.);
#20466=ORIENTED_EDGE('',*,*,#14950,.T.);
#20467=ORIENTED_EDGE('',*,*,#15153,.T.);
#20468=ORIENTED_EDGE('',*,*,#15154,.T.);
#20469=ORIENTED_EDGE('',*,*,#15151,.F.);
#20470=ORIENTED_EDGE('',*,*,#15155,.T.);
#20471=ORIENTED_EDGE('',*,*,#15156,.F.);
#20472=ORIENTED_EDGE('',*,*,#15157,.F.);
#20473=ORIENTED_EDGE('',*,*,#15150,.F.);
#20474=ORIENTED_EDGE('',*,*,#15158,.T.);
#20475=ORIENTED_EDGE('',*,*,#15159,.F.);
#20476=ORIENTED_EDGE('',*,*,#15155,.F.);
#20477=ORIENTED_EDGE('',*,*,#15160,.T.);
#20478=ORIENTED_EDGE('',*,*,#15161,.T.);
#20479=ORIENTED_EDGE('',*,*,#15162,.T.);
#20480=ORIENTED_EDGE('',*,*,#14930,.T.);
#20481=ORIENTED_EDGE('',*,*,#15163,.T.);
#20482=ORIENTED_EDGE('',*,*,#15164,.T.);
#20483=ORIENTED_EDGE('',*,*,#15161,.F.);
#20484=ORIENTED_EDGE('',*,*,#15165,.T.);
#20485=ORIENTED_EDGE('',*,*,#15166,.F.);
#20486=ORIENTED_EDGE('',*,*,#15167,.F.);
#20487=ORIENTED_EDGE('',*,*,#15160,.F.);
#20488=ORIENTED_EDGE('',*,*,#15168,.T.);
#20489=ORIENTED_EDGE('',*,*,#15169,.F.);
#20490=ORIENTED_EDGE('',*,*,#15165,.F.);
#20491=ORIENTED_EDGE('',*,*,#15170,.T.);
#20492=ORIENTED_EDGE('',*,*,#15171,.T.);
#20493=ORIENTED_EDGE('',*,*,#15172,.T.);
#20494=ORIENTED_EDGE('',*,*,#14910,.T.);
#20495=ORIENTED_EDGE('',*,*,#15173,.T.);
#20496=ORIENTED_EDGE('',*,*,#15174,.T.);
#20497=ORIENTED_EDGE('',*,*,#15171,.F.);
#20498=ORIENTED_EDGE('',*,*,#15175,.T.);
#20499=ORIENTED_EDGE('',*,*,#15176,.F.);
#20500=ORIENTED_EDGE('',*,*,#15177,.F.);
#20501=ORIENTED_EDGE('',*,*,#15170,.F.);
#20502=ORIENTED_EDGE('',*,*,#15178,.T.);
#20503=ORIENTED_EDGE('',*,*,#15179,.F.);
#20504=ORIENTED_EDGE('',*,*,#15175,.F.);
#20505=ORIENTED_EDGE('',*,*,#15180,.T.);
#20506=ORIENTED_EDGE('',*,*,#15181,.T.);
#20507=ORIENTED_EDGE('',*,*,#15182,.T.);
#20508=ORIENTED_EDGE('',*,*,#14890,.T.);
#20509=ORIENTED_EDGE('',*,*,#15183,.T.);
#20510=ORIENTED_EDGE('',*,*,#15184,.T.);
#20511=ORIENTED_EDGE('',*,*,#15181,.F.);
#20512=ORIENTED_EDGE('',*,*,#15185,.T.);
#20513=ORIENTED_EDGE('',*,*,#15186,.F.);
#20514=ORIENTED_EDGE('',*,*,#15187,.F.);
#20515=ORIENTED_EDGE('',*,*,#15180,.F.);
#20516=ORIENTED_EDGE('',*,*,#15188,.T.);
#20517=ORIENTED_EDGE('',*,*,#15189,.F.);
#20518=ORIENTED_EDGE('',*,*,#15185,.F.);
#20519=ORIENTED_EDGE('',*,*,#15190,.T.);
#20520=ORIENTED_EDGE('',*,*,#15191,.T.);
#20521=ORIENTED_EDGE('',*,*,#15192,.T.);
#20522=ORIENTED_EDGE('',*,*,#14870,.T.);
#20523=ORIENTED_EDGE('',*,*,#15193,.T.);
#20524=ORIENTED_EDGE('',*,*,#15194,.T.);
#20525=ORIENTED_EDGE('',*,*,#15191,.F.);
#20526=ORIENTED_EDGE('',*,*,#15195,.T.);
#20527=ORIENTED_EDGE('',*,*,#15196,.F.);
#20528=ORIENTED_EDGE('',*,*,#15197,.F.);
#20529=ORIENTED_EDGE('',*,*,#15190,.F.);
#20530=ORIENTED_EDGE('',*,*,#15198,.T.);
#20531=ORIENTED_EDGE('',*,*,#15199,.F.);
#20532=ORIENTED_EDGE('',*,*,#15195,.F.);
#20533=ORIENTED_EDGE('',*,*,#15200,.T.);
#20534=ORIENTED_EDGE('',*,*,#15201,.T.);
#20535=ORIENTED_EDGE('',*,*,#15202,.T.);
#20536=ORIENTED_EDGE('',*,*,#14850,.T.);
#20537=ORIENTED_EDGE('',*,*,#15203,.T.);
#20538=ORIENTED_EDGE('',*,*,#15204,.T.);
#20539=ORIENTED_EDGE('',*,*,#15201,.F.);
#20540=ORIENTED_EDGE('',*,*,#15205,.T.);
#20541=ORIENTED_EDGE('',*,*,#15206,.F.);
#20542=ORIENTED_EDGE('',*,*,#15207,.F.);
#20543=ORIENTED_EDGE('',*,*,#15200,.F.);
#20544=ORIENTED_EDGE('',*,*,#15208,.T.);
#20545=ORIENTED_EDGE('',*,*,#15209,.F.);
#20546=ORIENTED_EDGE('',*,*,#15205,.F.);
#20547=ORIENTED_EDGE('',*,*,#15210,.T.);
#20548=ORIENTED_EDGE('',*,*,#15211,.T.);
#20549=ORIENTED_EDGE('',*,*,#15212,.T.);
#20550=ORIENTED_EDGE('',*,*,#14830,.T.);
#20551=ORIENTED_EDGE('',*,*,#15213,.T.);
#20552=ORIENTED_EDGE('',*,*,#15214,.T.);
#20553=ORIENTED_EDGE('',*,*,#15211,.F.);
#20554=ORIENTED_EDGE('',*,*,#15215,.T.);
#20555=ORIENTED_EDGE('',*,*,#15216,.F.);
#20556=ORIENTED_EDGE('',*,*,#15217,.F.);
#20557=ORIENTED_EDGE('',*,*,#15210,.F.);
#20558=ORIENTED_EDGE('',*,*,#15218,.T.);
#20559=ORIENTED_EDGE('',*,*,#15219,.F.);
#20560=ORIENTED_EDGE('',*,*,#15215,.F.);
#20561=ORIENTED_EDGE('',*,*,#15220,.T.);
#20562=ORIENTED_EDGE('',*,*,#15221,.T.);
#20563=ORIENTED_EDGE('',*,*,#15222,.T.);
#20564=ORIENTED_EDGE('',*,*,#14810,.T.);
#20565=ORIENTED_EDGE('',*,*,#15223,.T.);
#20566=ORIENTED_EDGE('',*,*,#15224,.T.);
#20567=ORIENTED_EDGE('',*,*,#15221,.F.);
#20568=ORIENTED_EDGE('',*,*,#15225,.T.);
#20569=ORIENTED_EDGE('',*,*,#15226,.F.);
#20570=ORIENTED_EDGE('',*,*,#15227,.F.);
#20571=ORIENTED_EDGE('',*,*,#15220,.F.);
#20572=ORIENTED_EDGE('',*,*,#15228,.T.);
#20573=ORIENTED_EDGE('',*,*,#15229,.F.);
#20574=ORIENTED_EDGE('',*,*,#15225,.F.);
#20575=ORIENTED_EDGE('',*,*,#15230,.T.);
#20576=ORIENTED_EDGE('',*,*,#15231,.T.);
#20577=ORIENTED_EDGE('',*,*,#15232,.T.);
#20578=ORIENTED_EDGE('',*,*,#14790,.T.);
#20579=ORIENTED_EDGE('',*,*,#15233,.T.);
#20580=ORIENTED_EDGE('',*,*,#15234,.T.);
#20581=ORIENTED_EDGE('',*,*,#15231,.F.);
#20582=ORIENTED_EDGE('',*,*,#15235,.T.);
#20583=ORIENTED_EDGE('',*,*,#15236,.F.);
#20584=ORIENTED_EDGE('',*,*,#15237,.F.);
#20585=ORIENTED_EDGE('',*,*,#15230,.F.);
#20586=ORIENTED_EDGE('',*,*,#15238,.T.);
#20587=ORIENTED_EDGE('',*,*,#15239,.F.);
#20588=ORIENTED_EDGE('',*,*,#15235,.F.);
#20589=ORIENTED_EDGE('',*,*,#15240,.T.);
#20590=ORIENTED_EDGE('',*,*,#15241,.T.);
#20591=ORIENTED_EDGE('',*,*,#15242,.T.);
#20592=ORIENTED_EDGE('',*,*,#15243,.T.);
#20593=ORIENTED_EDGE('',*,*,#15115,.T.);
#20594=ORIENTED_EDGE('',*,*,#15119,.T.);
#20595=ORIENTED_EDGE('',*,*,#15243,.F.);
#20596=ORIENTED_EDGE('',*,*,#15244,.T.);
#20597=ORIENTED_EDGE('',*,*,#15245,.T.);
#20598=ORIENTED_EDGE('',*,*,#15246,.F.);
#20599=ORIENTED_EDGE('',*,*,#15247,.T.);
#20600=ORIENTED_EDGE('',*,*,#15248,.T.);
#20601=ORIENTED_EDGE('',*,*,#15249,.T.);
#20602=ORIENTED_EDGE('',*,*,#15250,.T.);
#20603=ORIENTED_EDGE('',*,*,#15251,.T.);
#20604=ORIENTED_EDGE('',*,*,#15252,.T.);
#20605=ORIENTED_EDGE('',*,*,#15253,.T.);
#20606=ORIENTED_EDGE('',*,*,#15254,.T.);
#20607=ORIENTED_EDGE('',*,*,#15255,.T.);
#20608=ORIENTED_EDGE('',*,*,#15256,.T.);
#20609=ORIENTED_EDGE('',*,*,#15257,.T.);
#20610=ORIENTED_EDGE('',*,*,#15258,.T.);
#20611=ORIENTED_EDGE('',*,*,#15259,.T.);
#20612=ORIENTED_EDGE('',*,*,#15260,.T.);
#20613=ORIENTED_EDGE('',*,*,#15261,.T.);
#20614=ORIENTED_EDGE('',*,*,#14995,.T.);
#20615=ORIENTED_EDGE('',*,*,#15262,.F.);
#20616=ORIENTED_EDGE('',*,*,#15263,.T.);
#20617=ORIENTED_EDGE('',*,*,#15264,.T.);
#20618=ORIENTED_EDGE('',*,*,#15265,.F.);
#20619=ORIENTED_EDGE('',*,*,#15266,.T.);
#20620=ORIENTED_EDGE('',*,*,#15267,.T.);
#20621=ORIENTED_EDGE('',*,*,#15268,.T.);
#20622=ORIENTED_EDGE('',*,*,#15269,.T.);
#20623=ORIENTED_EDGE('',*,*,#15270,.T.);
#20624=ORIENTED_EDGE('',*,*,#15271,.T.);
#20625=ORIENTED_EDGE('',*,*,#15272,.T.);
#20626=ORIENTED_EDGE('',*,*,#15273,.T.);
#20627=ORIENTED_EDGE('',*,*,#15274,.T.);
#20628=ORIENTED_EDGE('',*,*,#15275,.T.);
#20629=ORIENTED_EDGE('',*,*,#15276,.T.);
#20630=ORIENTED_EDGE('',*,*,#15277,.T.);
#20631=ORIENTED_EDGE('',*,*,#15278,.T.);
#20632=ORIENTED_EDGE('',*,*,#15279,.T.);
#20633=ORIENTED_EDGE('',*,*,#15280,.T.);
#20634=ORIENTED_EDGE('',*,*,#15006,.T.);
#20635=ORIENTED_EDGE('',*,*,#15281,.F.);
#20636=ORIENTED_EDGE('',*,*,#15282,.T.);
#20637=ORIENTED_EDGE('',*,*,#15283,.T.);
#20638=ORIENTED_EDGE('',*,*,#15284,.F.);
#20639=ORIENTED_EDGE('',*,*,#15285,.T.);
#20640=ORIENTED_EDGE('',*,*,#15286,.T.);
#20641=ORIENTED_EDGE('',*,*,#15287,.T.);
#20642=ORIENTED_EDGE('',*,*,#15288,.T.);
#20643=ORIENTED_EDGE('',*,*,#15289,.T.);
#20644=ORIENTED_EDGE('',*,*,#15290,.T.);
#20645=ORIENTED_EDGE('',*,*,#15291,.T.);
#20646=ORIENTED_EDGE('',*,*,#15292,.T.);
#20647=ORIENTED_EDGE('',*,*,#15293,.T.);
#20648=ORIENTED_EDGE('',*,*,#15294,.T.);
#20649=ORIENTED_EDGE('',*,*,#15295,.T.);
#20650=ORIENTED_EDGE('',*,*,#15296,.T.);
#20651=ORIENTED_EDGE('',*,*,#15297,.T.);
#20652=ORIENTED_EDGE('',*,*,#15298,.T.);
#20653=ORIENTED_EDGE('',*,*,#15299,.T.);
#20654=ORIENTED_EDGE('',*,*,#15017,.T.);
#20655=ORIENTED_EDGE('',*,*,#15300,.F.);
#20656=ORIENTED_EDGE('',*,*,#15301,.T.);
#20657=ORIENTED_EDGE('',*,*,#15302,.T.);
#20658=ORIENTED_EDGE('',*,*,#15303,.F.);
#20659=ORIENTED_EDGE('',*,*,#15304,.T.);
#20660=ORIENTED_EDGE('',*,*,#15305,.T.);
#20661=ORIENTED_EDGE('',*,*,#15306,.T.);
#20662=ORIENTED_EDGE('',*,*,#15307,.T.);
#20663=ORIENTED_EDGE('',*,*,#15308,.T.);
#20664=ORIENTED_EDGE('',*,*,#15309,.T.);
#20665=ORIENTED_EDGE('',*,*,#15310,.T.);
#20666=ORIENTED_EDGE('',*,*,#15311,.T.);
#20667=ORIENTED_EDGE('',*,*,#15312,.T.);
#20668=ORIENTED_EDGE('',*,*,#15313,.T.);
#20669=ORIENTED_EDGE('',*,*,#15314,.T.);
#20670=ORIENTED_EDGE('',*,*,#15315,.T.);
#20671=ORIENTED_EDGE('',*,*,#15316,.T.);
#20672=ORIENTED_EDGE('',*,*,#15317,.T.);
#20673=ORIENTED_EDGE('',*,*,#15318,.T.);
#20674=ORIENTED_EDGE('',*,*,#15028,.T.);
#20675=ORIENTED_EDGE('',*,*,#15319,.F.);
#20676=ORIENTED_EDGE('',*,*,#15320,.T.);
#20677=ORIENTED_EDGE('',*,*,#15321,.T.);
#20678=ORIENTED_EDGE('',*,*,#15322,.F.);
#20679=ORIENTED_EDGE('',*,*,#15323,.T.);
#20680=ORIENTED_EDGE('',*,*,#15324,.T.);
#20681=ORIENTED_EDGE('',*,*,#15325,.T.);
#20682=ORIENTED_EDGE('',*,*,#15326,.T.);
#20683=ORIENTED_EDGE('',*,*,#15327,.T.);
#20684=ORIENTED_EDGE('',*,*,#15328,.T.);
#20685=ORIENTED_EDGE('',*,*,#15329,.T.);
#20686=ORIENTED_EDGE('',*,*,#15330,.T.);
#20687=ORIENTED_EDGE('',*,*,#15331,.T.);
#20688=ORIENTED_EDGE('',*,*,#15332,.T.);
#20689=ORIENTED_EDGE('',*,*,#15333,.T.);
#20690=ORIENTED_EDGE('',*,*,#15334,.T.);
#20691=ORIENTED_EDGE('',*,*,#15335,.T.);
#20692=ORIENTED_EDGE('',*,*,#15336,.T.);
#20693=ORIENTED_EDGE('',*,*,#15337,.T.);
#20694=ORIENTED_EDGE('',*,*,#15039,.T.);
#20695=ORIENTED_EDGE('',*,*,#15338,.F.);
#20696=ORIENTED_EDGE('',*,*,#15339,.T.);
#20697=ORIENTED_EDGE('',*,*,#15340,.T.);
#20698=ORIENTED_EDGE('',*,*,#15341,.F.);
#20699=ORIENTED_EDGE('',*,*,#15342,.T.);
#20700=ORIENTED_EDGE('',*,*,#15343,.T.);
#20701=ORIENTED_EDGE('',*,*,#15344,.T.);
#20702=ORIENTED_EDGE('',*,*,#15345,.T.);
#20703=ORIENTED_EDGE('',*,*,#15346,.T.);
#20704=ORIENTED_EDGE('',*,*,#15347,.T.);
#20705=ORIENTED_EDGE('',*,*,#15348,.T.);
#20706=ORIENTED_EDGE('',*,*,#15349,.T.);
#20707=ORIENTED_EDGE('',*,*,#15350,.T.);
#20708=ORIENTED_EDGE('',*,*,#15351,.T.);
#20709=ORIENTED_EDGE('',*,*,#15352,.T.);
#20710=ORIENTED_EDGE('',*,*,#15353,.T.);
#20711=ORIENTED_EDGE('',*,*,#15354,.T.);
#20712=ORIENTED_EDGE('',*,*,#15355,.T.);
#20713=ORIENTED_EDGE('',*,*,#15356,.T.);
#20714=ORIENTED_EDGE('',*,*,#15050,.T.);
#20715=ORIENTED_EDGE('',*,*,#15357,.F.);
#20716=ORIENTED_EDGE('',*,*,#15358,.T.);
#20717=ORIENTED_EDGE('',*,*,#15359,.T.);
#20718=ORIENTED_EDGE('',*,*,#15360,.F.);
#20719=ORIENTED_EDGE('',*,*,#15361,.T.);
#20720=ORIENTED_EDGE('',*,*,#15362,.T.);
#20721=ORIENTED_EDGE('',*,*,#15363,.T.);
#20722=ORIENTED_EDGE('',*,*,#15364,.T.);
#20723=ORIENTED_EDGE('',*,*,#15365,.T.);
#20724=ORIENTED_EDGE('',*,*,#15366,.T.);
#20725=ORIENTED_EDGE('',*,*,#15367,.T.);
#20726=ORIENTED_EDGE('',*,*,#15368,.T.);
#20727=ORIENTED_EDGE('',*,*,#15369,.T.);
#20728=ORIENTED_EDGE('',*,*,#15370,.T.);
#20729=ORIENTED_EDGE('',*,*,#15371,.T.);
#20730=ORIENTED_EDGE('',*,*,#15372,.T.);
#20731=ORIENTED_EDGE('',*,*,#15373,.T.);
#20732=ORIENTED_EDGE('',*,*,#15374,.T.);
#20733=ORIENTED_EDGE('',*,*,#15375,.T.);
#20734=ORIENTED_EDGE('',*,*,#15061,.T.);
#20735=ORIENTED_EDGE('',*,*,#15376,.F.);
#20736=ORIENTED_EDGE('',*,*,#15377,.T.);
#20737=ORIENTED_EDGE('',*,*,#15378,.T.);
#20738=ORIENTED_EDGE('',*,*,#15379,.F.);
#20739=ORIENTED_EDGE('',*,*,#15380,.T.);
#20740=ORIENTED_EDGE('',*,*,#15381,.T.);
#20741=ORIENTED_EDGE('',*,*,#15382,.T.);
#20742=ORIENTED_EDGE('',*,*,#15383,.T.);
#20743=ORIENTED_EDGE('',*,*,#15384,.T.);
#20744=ORIENTED_EDGE('',*,*,#15385,.T.);
#20745=ORIENTED_EDGE('',*,*,#15386,.T.);
#20746=ORIENTED_EDGE('',*,*,#15387,.T.);
#20747=ORIENTED_EDGE('',*,*,#15388,.T.);
#20748=ORIENTED_EDGE('',*,*,#15389,.T.);
#20749=ORIENTED_EDGE('',*,*,#15390,.T.);
#20750=ORIENTED_EDGE('',*,*,#15391,.T.);
#20751=ORIENTED_EDGE('',*,*,#15392,.T.);
#20752=ORIENTED_EDGE('',*,*,#15393,.T.);
#20753=ORIENTED_EDGE('',*,*,#15394,.T.);
#20754=ORIENTED_EDGE('',*,*,#15072,.T.);
#20755=ORIENTED_EDGE('',*,*,#15395,.F.);
#20756=ORIENTED_EDGE('',*,*,#15396,.T.);
#20757=ORIENTED_EDGE('',*,*,#15397,.T.);
#20758=ORIENTED_EDGE('',*,*,#15398,.F.);
#20759=ORIENTED_EDGE('',*,*,#15399,.T.);
#20760=ORIENTED_EDGE('',*,*,#15400,.T.);
#20761=ORIENTED_EDGE('',*,*,#15401,.T.);
#20762=ORIENTED_EDGE('',*,*,#15402,.T.);
#20763=ORIENTED_EDGE('',*,*,#15403,.T.);
#20764=ORIENTED_EDGE('',*,*,#15404,.T.);
#20765=ORIENTED_EDGE('',*,*,#15405,.T.);
#20766=ORIENTED_EDGE('',*,*,#15406,.T.);
#20767=ORIENTED_EDGE('',*,*,#15407,.T.);
#20768=ORIENTED_EDGE('',*,*,#15408,.T.);
#20769=ORIENTED_EDGE('',*,*,#15409,.T.);
#20770=ORIENTED_EDGE('',*,*,#15410,.T.);
#20771=ORIENTED_EDGE('',*,*,#15411,.T.);
#20772=ORIENTED_EDGE('',*,*,#15412,.T.);
#20773=ORIENTED_EDGE('',*,*,#15413,.T.);
#20774=ORIENTED_EDGE('',*,*,#15083,.T.);
#20775=ORIENTED_EDGE('',*,*,#15414,.F.);
#20776=ORIENTED_EDGE('',*,*,#15415,.T.);
#20777=ORIENTED_EDGE('',*,*,#15416,.T.);
#20778=ORIENTED_EDGE('',*,*,#15417,.F.);
#20779=ORIENTED_EDGE('',*,*,#15418,.T.);
#20780=ORIENTED_EDGE('',*,*,#15419,.T.);
#20781=ORIENTED_EDGE('',*,*,#15420,.T.);
#20782=ORIENTED_EDGE('',*,*,#15421,.T.);
#20783=ORIENTED_EDGE('',*,*,#15422,.T.);
#20784=ORIENTED_EDGE('',*,*,#15423,.T.);
#20785=ORIENTED_EDGE('',*,*,#15424,.T.);
#20786=ORIENTED_EDGE('',*,*,#15425,.T.);
#20787=ORIENTED_EDGE('',*,*,#15426,.T.);
#20788=ORIENTED_EDGE('',*,*,#15427,.T.);
#20789=ORIENTED_EDGE('',*,*,#15428,.T.);
#20790=ORIENTED_EDGE('',*,*,#15429,.T.);
#20791=ORIENTED_EDGE('',*,*,#15430,.T.);
#20792=ORIENTED_EDGE('',*,*,#15431,.T.);
#20793=ORIENTED_EDGE('',*,*,#15432,.T.);
#20794=ORIENTED_EDGE('',*,*,#15094,.T.);
#20795=ORIENTED_EDGE('',*,*,#15433,.F.);
#20796=ORIENTED_EDGE('',*,*,#15434,.T.);
#20797=ORIENTED_EDGE('',*,*,#15435,.T.);
#20798=ORIENTED_EDGE('',*,*,#15436,.F.);
#20799=ORIENTED_EDGE('',*,*,#15437,.T.);
#20800=ORIENTED_EDGE('',*,*,#15438,.T.);
#20801=ORIENTED_EDGE('',*,*,#15439,.T.);
#20802=ORIENTED_EDGE('',*,*,#15440,.T.);
#20803=ORIENTED_EDGE('',*,*,#15441,.T.);
#20804=ORIENTED_EDGE('',*,*,#15442,.T.);
#20805=ORIENTED_EDGE('',*,*,#15443,.T.);
#20806=ORIENTED_EDGE('',*,*,#15444,.T.);
#20807=ORIENTED_EDGE('',*,*,#15445,.T.);
#20808=ORIENTED_EDGE('',*,*,#15446,.T.);
#20809=ORIENTED_EDGE('',*,*,#15447,.T.);
#20810=ORIENTED_EDGE('',*,*,#15448,.T.);
#20811=ORIENTED_EDGE('',*,*,#15449,.T.);
#20812=ORIENTED_EDGE('',*,*,#15450,.T.);
#20813=ORIENTED_EDGE('',*,*,#15451,.T.);
#20814=ORIENTED_EDGE('',*,*,#15105,.T.);
#20815=ORIENTED_EDGE('',*,*,#15452,.F.);
#20816=ORIENTED_EDGE('',*,*,#15453,.T.);
#20817=ORIENTED_EDGE('',*,*,#15454,.T.);
#20818=ORIENTED_EDGE('',*,*,#15455,.F.);
#20819=ORIENTED_EDGE('',*,*,#15456,.T.);
#20820=ORIENTED_EDGE('',*,*,#15457,.T.);
#20821=ORIENTED_EDGE('',*,*,#15458,.T.);
#20822=ORIENTED_EDGE('',*,*,#15459,.T.);
#20823=ORIENTED_EDGE('',*,*,#15460,.T.);
#20824=ORIENTED_EDGE('',*,*,#15461,.T.);
#20825=ORIENTED_EDGE('',*,*,#15462,.T.);
#20826=ORIENTED_EDGE('',*,*,#15463,.T.);
#20827=ORIENTED_EDGE('',*,*,#15464,.T.);
#20828=ORIENTED_EDGE('',*,*,#15465,.T.);
#20829=ORIENTED_EDGE('',*,*,#15466,.T.);
#20830=ORIENTED_EDGE('',*,*,#15467,.T.);
#20831=ORIENTED_EDGE('',*,*,#15468,.T.);
#20832=ORIENTED_EDGE('',*,*,#15469,.T.);
#20833=ORIENTED_EDGE('',*,*,#15470,.T.);
#20834=ORIENTED_EDGE('',*,*,#15116,.T.);
#20835=ORIENTED_EDGE('',*,*,#15471,.F.);
#20836=ORIENTED_EDGE('',*,*,#15472,.T.);
#20837=ORIENTED_EDGE('',*,*,#15455,.T.);
#20838=ORIENTED_EDGE('',*,*,#15473,.T.);
#20839=ORIENTED_EDGE('',*,*,#15236,.T.);
#20840=ORIENTED_EDGE('',*,*,#15239,.T.);
#20841=ORIENTED_EDGE('',*,*,#15474,.T.);
#20842=ORIENTED_EDGE('',*,*,#15475,.T.);
#20843=ORIENTED_EDGE('',*,*,#15476,.T.);
#20844=ORIENTED_EDGE('',*,*,#15477,.T.);
#20845=ORIENTED_EDGE('',*,*,#15452,.T.);
#20846=ORIENTED_EDGE('',*,*,#15104,.T.);
#20847=ORIENTED_EDGE('',*,*,#15108,.T.);
#20848=ORIENTED_EDGE('',*,*,#15478,.T.);
#20849=ORIENTED_EDGE('',*,*,#15436,.T.);
#20850=ORIENTED_EDGE('',*,*,#15479,.T.);
#20851=ORIENTED_EDGE('',*,*,#15226,.T.);
#20852=ORIENTED_EDGE('',*,*,#15229,.T.);
#20853=ORIENTED_EDGE('',*,*,#15480,.T.);
#20854=ORIENTED_EDGE('',*,*,#15481,.T.);
#20855=ORIENTED_EDGE('',*,*,#15482,.T.);
#20856=ORIENTED_EDGE('',*,*,#15483,.T.);
#20857=ORIENTED_EDGE('',*,*,#15433,.T.);
#20858=ORIENTED_EDGE('',*,*,#15093,.T.);
#20859=ORIENTED_EDGE('',*,*,#15097,.T.);
#20860=ORIENTED_EDGE('',*,*,#15484,.T.);
#20861=ORIENTED_EDGE('',*,*,#15417,.T.);
#20862=ORIENTED_EDGE('',*,*,#15485,.T.);
#20863=ORIENTED_EDGE('',*,*,#15216,.T.);
#20864=ORIENTED_EDGE('',*,*,#15219,.T.);
#20865=ORIENTED_EDGE('',*,*,#15486,.T.);
#20866=ORIENTED_EDGE('',*,*,#15487,.T.);
#20867=ORIENTED_EDGE('',*,*,#15488,.T.);
#20868=ORIENTED_EDGE('',*,*,#15489,.T.);
#20869=ORIENTED_EDGE('',*,*,#15414,.T.);
#20870=ORIENTED_EDGE('',*,*,#15082,.T.);
#20871=ORIENTED_EDGE('',*,*,#15086,.T.);
#20872=ORIENTED_EDGE('',*,*,#15490,.T.);
#20873=ORIENTED_EDGE('',*,*,#15398,.T.);
#20874=ORIENTED_EDGE('',*,*,#15491,.T.);
#20875=ORIENTED_EDGE('',*,*,#15206,.T.);
#20876=ORIENTED_EDGE('',*,*,#15209,.T.);
#20877=ORIENTED_EDGE('',*,*,#15492,.T.);
#20878=ORIENTED_EDGE('',*,*,#15493,.T.);
#20879=ORIENTED_EDGE('',*,*,#15494,.T.);
#20880=ORIENTED_EDGE('',*,*,#15495,.T.);
#20881=ORIENTED_EDGE('',*,*,#15395,.T.);
#20882=ORIENTED_EDGE('',*,*,#15071,.T.);
#20883=ORIENTED_EDGE('',*,*,#15075,.T.);
#20884=ORIENTED_EDGE('',*,*,#15496,.T.);
#20885=ORIENTED_EDGE('',*,*,#15379,.T.);
#20886=ORIENTED_EDGE('',*,*,#15497,.T.);
#20887=ORIENTED_EDGE('',*,*,#15196,.T.);
#20888=ORIENTED_EDGE('',*,*,#15199,.T.);
#20889=ORIENTED_EDGE('',*,*,#15498,.T.);
#20890=ORIENTED_EDGE('',*,*,#15499,.T.);
#20891=ORIENTED_EDGE('',*,*,#15500,.T.);
#20892=ORIENTED_EDGE('',*,*,#15501,.T.);
#20893=ORIENTED_EDGE('',*,*,#15376,.T.);
#20894=ORIENTED_EDGE('',*,*,#15060,.T.);
#20895=ORIENTED_EDGE('',*,*,#15064,.T.);
#20896=ORIENTED_EDGE('',*,*,#15502,.T.);
#20897=ORIENTED_EDGE('',*,*,#15360,.T.);
#20898=ORIENTED_EDGE('',*,*,#15503,.T.);
#20899=ORIENTED_EDGE('',*,*,#15186,.T.);
#20900=ORIENTED_EDGE('',*,*,#15189,.T.);
#20901=ORIENTED_EDGE('',*,*,#15504,.T.);
#20902=ORIENTED_EDGE('',*,*,#15505,.T.);
#20903=ORIENTED_EDGE('',*,*,#15506,.T.);
#20904=ORIENTED_EDGE('',*,*,#15507,.T.);
#20905=ORIENTED_EDGE('',*,*,#15357,.T.);
#20906=ORIENTED_EDGE('',*,*,#15049,.T.);
#20907=ORIENTED_EDGE('',*,*,#15053,.T.);
#20908=ORIENTED_EDGE('',*,*,#15508,.T.);
#20909=ORIENTED_EDGE('',*,*,#15341,.T.);
#20910=ORIENTED_EDGE('',*,*,#15509,.T.);
#20911=ORIENTED_EDGE('',*,*,#15176,.T.);
#20912=ORIENTED_EDGE('',*,*,#15179,.T.);
#20913=ORIENTED_EDGE('',*,*,#15510,.T.);
#20914=ORIENTED_EDGE('',*,*,#15511,.T.);
#20915=ORIENTED_EDGE('',*,*,#15512,.T.);
#20916=ORIENTED_EDGE('',*,*,#15513,.T.);
#20917=ORIENTED_EDGE('',*,*,#15338,.T.);
#20918=ORIENTED_EDGE('',*,*,#15038,.T.);
#20919=ORIENTED_EDGE('',*,*,#15042,.T.);
#20920=ORIENTED_EDGE('',*,*,#15514,.T.);
#20921=ORIENTED_EDGE('',*,*,#15322,.T.);
#20922=ORIENTED_EDGE('',*,*,#15515,.T.);
#20923=ORIENTED_EDGE('',*,*,#15166,.T.);
#20924=ORIENTED_EDGE('',*,*,#15169,.T.);
#20925=ORIENTED_EDGE('',*,*,#15516,.T.);
#20926=ORIENTED_EDGE('',*,*,#15517,.T.);
#20927=ORIENTED_EDGE('',*,*,#15518,.T.);
#20928=ORIENTED_EDGE('',*,*,#15519,.T.);
#20929=ORIENTED_EDGE('',*,*,#15319,.T.);
#20930=ORIENTED_EDGE('',*,*,#15027,.T.);
#20931=ORIENTED_EDGE('',*,*,#15031,.T.);
#20932=ORIENTED_EDGE('',*,*,#15520,.T.);
#20933=ORIENTED_EDGE('',*,*,#15303,.T.);
#20934=ORIENTED_EDGE('',*,*,#15521,.T.);
#20935=ORIENTED_EDGE('',*,*,#15156,.T.);
#20936=ORIENTED_EDGE('',*,*,#15159,.T.);
#20937=ORIENTED_EDGE('',*,*,#15522,.T.);
#20938=ORIENTED_EDGE('',*,*,#15523,.T.);
#20939=ORIENTED_EDGE('',*,*,#15524,.T.);
#20940=ORIENTED_EDGE('',*,*,#15525,.T.);
#20941=ORIENTED_EDGE('',*,*,#15300,.T.);
#20942=ORIENTED_EDGE('',*,*,#15016,.T.);
#20943=ORIENTED_EDGE('',*,*,#15020,.T.);
#20944=ORIENTED_EDGE('',*,*,#15526,.T.);
#20945=ORIENTED_EDGE('',*,*,#15284,.T.);
#20946=ORIENTED_EDGE('',*,*,#15527,.T.);
#20947=ORIENTED_EDGE('',*,*,#15146,.T.);
#20948=ORIENTED_EDGE('',*,*,#15149,.T.);
#20949=ORIENTED_EDGE('',*,*,#15528,.T.);
#20950=ORIENTED_EDGE('',*,*,#15529,.T.);
#20951=ORIENTED_EDGE('',*,*,#15530,.T.);
#20952=ORIENTED_EDGE('',*,*,#15531,.T.);
#20953=ORIENTED_EDGE('',*,*,#15281,.T.);
#20954=ORIENTED_EDGE('',*,*,#15005,.T.);
#20955=ORIENTED_EDGE('',*,*,#15009,.T.);
#20956=ORIENTED_EDGE('',*,*,#15532,.T.);
#20957=ORIENTED_EDGE('',*,*,#15265,.T.);
#20958=ORIENTED_EDGE('',*,*,#15533,.T.);
#20959=ORIENTED_EDGE('',*,*,#15136,.T.);
#20960=ORIENTED_EDGE('',*,*,#15139,.T.);
#20961=ORIENTED_EDGE('',*,*,#15534,.T.);
#20962=ORIENTED_EDGE('',*,*,#15535,.T.);
#20963=ORIENTED_EDGE('',*,*,#15536,.T.);
#20964=ORIENTED_EDGE('',*,*,#15537,.T.);
#20965=ORIENTED_EDGE('',*,*,#15262,.T.);
#20966=ORIENTED_EDGE('',*,*,#14994,.T.);
#20967=ORIENTED_EDGE('',*,*,#14998,.T.);
#20968=ORIENTED_EDGE('',*,*,#15538,.T.);
#20969=ORIENTED_EDGE('',*,*,#15246,.T.);
#20970=ORIENTED_EDGE('',*,*,#15539,.T.);
#20971=ORIENTED_EDGE('',*,*,#15126,.T.);
#20972=ORIENTED_EDGE('',*,*,#15129,.T.);
#20973=ORIENTED_EDGE('',*,*,#15540,.T.);
#20974=ORIENTED_EDGE('',*,*,#14772,.F.);
#20975=ORIENTED_EDGE('',*,*,#15541,.T.);
#20976=ORIENTED_EDGE('',*,*,#15244,.F.);
#20977=ORIENTED_EDGE('',*,*,#15242,.F.);
#20978=ORIENTED_EDGE('',*,*,#15542,.F.);
#20979=ORIENTED_EDGE('',*,*,#15110,.F.);
#20980=ORIENTED_EDGE('',*,*,#15111,.F.);
#20981=ORIENTED_EDGE('',*,*,#15542,.T.);
#20982=ORIENTED_EDGE('',*,*,#15241,.F.);
#20983=ORIENTED_EDGE('',*,*,#15543,.F.);
#20984=ORIENTED_EDGE('',*,*,#15112,.F.);
#20985=ORIENTED_EDGE('',*,*,#15543,.T.);
#20986=ORIENTED_EDGE('',*,*,#15240,.F.);
#20987=ORIENTED_EDGE('',*,*,#15118,.F.);
#20988=ORIENTED_EDGE('',*,*,#14775,.F.);
#20989=ORIENTED_EDGE('',*,*,#15117,.T.);
#20990=ORIENTED_EDGE('',*,*,#15470,.F.);
#20991=ORIENTED_EDGE('',*,*,#15544,.F.);
#20992=ORIENTED_EDGE('',*,*,#14776,.F.);
#20993=ORIENTED_EDGE('',*,*,#15544,.T.);
#20994=ORIENTED_EDGE('',*,*,#15469,.F.);
#20995=ORIENTED_EDGE('',*,*,#15545,.F.);
#20996=ORIENTED_EDGE('',*,*,#14777,.F.);
#20997=ORIENTED_EDGE('',*,*,#15545,.T.);
#20998=ORIENTED_EDGE('',*,*,#15468,.F.);
#20999=ORIENTED_EDGE('',*,*,#15546,.F.);
#21000=ORIENTED_EDGE('',*,*,#14778,.F.);
#21001=ORIENTED_EDGE('',*,*,#15546,.T.);
#21002=ORIENTED_EDGE('',*,*,#15467,.F.);
#21003=ORIENTED_EDGE('',*,*,#15547,.F.);
#21004=ORIENTED_EDGE('',*,*,#14779,.F.);
#21005=ORIENTED_EDGE('',*,*,#15547,.T.);
#21006=ORIENTED_EDGE('',*,*,#15466,.F.);
#21007=ORIENTED_EDGE('',*,*,#15548,.F.);
#21008=ORIENTED_EDGE('',*,*,#14780,.F.);
#21009=ORIENTED_EDGE('',*,*,#15548,.T.);
#21010=ORIENTED_EDGE('',*,*,#15465,.F.);
#21011=ORIENTED_EDGE('',*,*,#15549,.F.);
#21012=ORIENTED_EDGE('',*,*,#14781,.F.);
#21013=ORIENTED_EDGE('',*,*,#15549,.T.);
#21014=ORIENTED_EDGE('',*,*,#15464,.F.);
#21015=ORIENTED_EDGE('',*,*,#15550,.F.);
#21016=ORIENTED_EDGE('',*,*,#14782,.F.);
#21017=ORIENTED_EDGE('',*,*,#15550,.T.);
#21018=ORIENTED_EDGE('',*,*,#15463,.F.);
#21019=ORIENTED_EDGE('',*,*,#15551,.F.);
#21020=ORIENTED_EDGE('',*,*,#14783,.F.);
#21021=ORIENTED_EDGE('',*,*,#15551,.T.);
#21022=ORIENTED_EDGE('',*,*,#15462,.F.);
#21023=ORIENTED_EDGE('',*,*,#15552,.F.);
#21024=ORIENTED_EDGE('',*,*,#14784,.F.);
#21025=ORIENTED_EDGE('',*,*,#15552,.T.);
#21026=ORIENTED_EDGE('',*,*,#15461,.F.);
#21027=ORIENTED_EDGE('',*,*,#15553,.F.);
#21028=ORIENTED_EDGE('',*,*,#14785,.F.);
#21029=ORIENTED_EDGE('',*,*,#15553,.T.);
#21030=ORIENTED_EDGE('',*,*,#15460,.F.);
#21031=ORIENTED_EDGE('',*,*,#15554,.F.);
#21032=ORIENTED_EDGE('',*,*,#14786,.F.);
#21033=ORIENTED_EDGE('',*,*,#15554,.T.);
#21034=ORIENTED_EDGE('',*,*,#15459,.F.);
#21035=ORIENTED_EDGE('',*,*,#15555,.F.);
#21036=ORIENTED_EDGE('',*,*,#14787,.F.);
#21037=ORIENTED_EDGE('',*,*,#15555,.T.);
#21038=ORIENTED_EDGE('',*,*,#15458,.F.);
#21039=ORIENTED_EDGE('',*,*,#15556,.F.);
#21040=ORIENTED_EDGE('',*,*,#14788,.F.);
#21041=ORIENTED_EDGE('',*,*,#15556,.T.);
#21042=ORIENTED_EDGE('',*,*,#15457,.F.);
#21043=ORIENTED_EDGE('',*,*,#15557,.F.);
#21044=ORIENTED_EDGE('',*,*,#15233,.F.);
#21045=ORIENTED_EDGE('',*,*,#14789,.F.);
#21046=ORIENTED_EDGE('',*,*,#15557,.T.);
#21047=ORIENTED_EDGE('',*,*,#15456,.F.);
#21048=ORIENTED_EDGE('',*,*,#15472,.F.);
#21049=ORIENTED_EDGE('',*,*,#15558,.F.);
#21050=ORIENTED_EDGE('',*,*,#15234,.F.);
#21051=ORIENTED_EDGE('',*,*,#15558,.T.);
#21052=ORIENTED_EDGE('',*,*,#15474,.F.);
#21053=ORIENTED_EDGE('',*,*,#15238,.F.);
#21054=ORIENTED_EDGE('',*,*,#14791,.F.);
#21055=ORIENTED_EDGE('',*,*,#15232,.F.);
#21056=ORIENTED_EDGE('',*,*,#15237,.T.);
#21057=ORIENTED_EDGE('',*,*,#15473,.F.);
#21058=ORIENTED_EDGE('',*,*,#15454,.F.);
#21059=ORIENTED_EDGE('',*,*,#15559,.F.);
#21060=ORIENTED_EDGE('',*,*,#14792,.F.);
#21061=ORIENTED_EDGE('',*,*,#15559,.T.);
#21062=ORIENTED_EDGE('',*,*,#15453,.F.);
#21063=ORIENTED_EDGE('',*,*,#15477,.F.);
#21064=ORIENTED_EDGE('',*,*,#15560,.F.);
#21065=ORIENTED_EDGE('',*,*,#15099,.F.);
#21066=ORIENTED_EDGE('',*,*,#15100,.F.);
#21067=ORIENTED_EDGE('',*,*,#15560,.T.);
#21068=ORIENTED_EDGE('',*,*,#15476,.F.);
#21069=ORIENTED_EDGE('',*,*,#15561,.F.);
#21070=ORIENTED_EDGE('',*,*,#15101,.F.);
#21071=ORIENTED_EDGE('',*,*,#15561,.T.);
#21072=ORIENTED_EDGE('',*,*,#15475,.F.);
#21073=ORIENTED_EDGE('',*,*,#15107,.F.);
#21074=ORIENTED_EDGE('',*,*,#14795,.F.);
#21075=ORIENTED_EDGE('',*,*,#15106,.T.);
#21076=ORIENTED_EDGE('',*,*,#15451,.F.);
#21077=ORIENTED_EDGE('',*,*,#15562,.F.);
#21078=ORIENTED_EDGE('',*,*,#14796,.F.);
#21079=ORIENTED_EDGE('',*,*,#15562,.T.);
#21080=ORIENTED_EDGE('',*,*,#15450,.F.);
#21081=ORIENTED_EDGE('',*,*,#15563,.F.);
#21082=ORIENTED_EDGE('',*,*,#14797,.F.);
#21083=ORIENTED_EDGE('',*,*,#15563,.T.);
#21084=ORIENTED_EDGE('',*,*,#15449,.F.);
#21085=ORIENTED_EDGE('',*,*,#15564,.F.);
#21086=ORIENTED_EDGE('',*,*,#14798,.F.);
#21087=ORIENTED_EDGE('',*,*,#15564,.T.);
#21088=ORIENTED_EDGE('',*,*,#15448,.F.);
#21089=ORIENTED_EDGE('',*,*,#15565,.F.);
#21090=ORIENTED_EDGE('',*,*,#14799,.F.);
#21091=ORIENTED_EDGE('',*,*,#15565,.T.);
#21092=ORIENTED_EDGE('',*,*,#15447,.F.);
#21093=ORIENTED_EDGE('',*,*,#15566,.F.);
#21094=ORIENTED_EDGE('',*,*,#14800,.F.);
#21095=ORIENTED_EDGE('',*,*,#15566,.T.);
#21096=ORIENTED_EDGE('',*,*,#15446,.F.);
#21097=ORIENTED_EDGE('',*,*,#15567,.F.);
#21098=ORIENTED_EDGE('',*,*,#14801,.F.);
#21099=ORIENTED_EDGE('',*,*,#15567,.T.);
#21100=ORIENTED_EDGE('',*,*,#15445,.F.);
#21101=ORIENTED_EDGE('',*,*,#15568,.F.);
#21102=ORIENTED_EDGE('',*,*,#14802,.F.);
#21103=ORIENTED_EDGE('',*,*,#15568,.T.);
#21104=ORIENTED_EDGE('',*,*,#15444,.F.);
#21105=ORIENTED_EDGE('',*,*,#15569,.F.);
#21106=ORIENTED_EDGE('',*,*,#14803,.F.);
#21107=ORIENTED_EDGE('',*,*,#15569,.T.);
#21108=ORIENTED_EDGE('',*,*,#15443,.F.);
#21109=ORIENTED_EDGE('',*,*,#15570,.F.);
#21110=ORIENTED_EDGE('',*,*,#14804,.F.);
#21111=ORIENTED_EDGE('',*,*,#15570,.T.);
#21112=ORIENTED_EDGE('',*,*,#15442,.F.);
#21113=ORIENTED_EDGE('',*,*,#15571,.F.);
#21114=ORIENTED_EDGE('',*,*,#14805,.F.);
#21115=ORIENTED_EDGE('',*,*,#15571,.T.);
#21116=ORIENTED_EDGE('',*,*,#15441,.F.);
#21117=ORIENTED_EDGE('',*,*,#15572,.F.);
#21118=ORIENTED_EDGE('',*,*,#14806,.F.);
#21119=ORIENTED_EDGE('',*,*,#15572,.T.);
#21120=ORIENTED_EDGE('',*,*,#15440,.F.);
#21121=ORIENTED_EDGE('',*,*,#15573,.F.);
#21122=ORIENTED_EDGE('',*,*,#14807,.F.);
#21123=ORIENTED_EDGE('',*,*,#15573,.T.);
#21124=ORIENTED_EDGE('',*,*,#15439,.F.);
#21125=ORIENTED_EDGE('',*,*,#15574,.F.);
#21126=ORIENTED_EDGE('',*,*,#14808,.F.);
#21127=ORIENTED_EDGE('',*,*,#15574,.T.);
#21128=ORIENTED_EDGE('',*,*,#15438,.F.);
#21129=ORIENTED_EDGE('',*,*,#15575,.F.);
#21130=ORIENTED_EDGE('',*,*,#15223,.F.);
#21131=ORIENTED_EDGE('',*,*,#14809,.F.);
#21132=ORIENTED_EDGE('',*,*,#15575,.T.);
#21133=ORIENTED_EDGE('',*,*,#15437,.F.);
#21134=ORIENTED_EDGE('',*,*,#15478,.F.);
#21135=ORIENTED_EDGE('',*,*,#15576,.F.);
#21136=ORIENTED_EDGE('',*,*,#15224,.F.);
#21137=ORIENTED_EDGE('',*,*,#15576,.T.);
#21138=ORIENTED_EDGE('',*,*,#15480,.F.);
#21139=ORIENTED_EDGE('',*,*,#15228,.F.);
#21140=ORIENTED_EDGE('',*,*,#14811,.F.);
#21141=ORIENTED_EDGE('',*,*,#15222,.F.);
#21142=ORIENTED_EDGE('',*,*,#15227,.T.);
#21143=ORIENTED_EDGE('',*,*,#15479,.F.);
#21144=ORIENTED_EDGE('',*,*,#15435,.F.);
#21145=ORIENTED_EDGE('',*,*,#15577,.F.);
#21146=ORIENTED_EDGE('',*,*,#14812,.F.);
#21147=ORIENTED_EDGE('',*,*,#15577,.T.);
#21148=ORIENTED_EDGE('',*,*,#15434,.F.);
#21149=ORIENTED_EDGE('',*,*,#15483,.F.);
#21150=ORIENTED_EDGE('',*,*,#15578,.F.);
#21151=ORIENTED_EDGE('',*,*,#15088,.F.);
#21152=ORIENTED_EDGE('',*,*,#15089,.F.);
#21153=ORIENTED_EDGE('',*,*,#15578,.T.);
#21154=ORIENTED_EDGE('',*,*,#15482,.F.);
#21155=ORIENTED_EDGE('',*,*,#15579,.F.);
#21156=ORIENTED_EDGE('',*,*,#15090,.F.);
#21157=ORIENTED_EDGE('',*,*,#15579,.T.);
#21158=ORIENTED_EDGE('',*,*,#15481,.F.);
#21159=ORIENTED_EDGE('',*,*,#15096,.F.);
#21160=ORIENTED_EDGE('',*,*,#14815,.F.);
#21161=ORIENTED_EDGE('',*,*,#15095,.T.);
#21162=ORIENTED_EDGE('',*,*,#15432,.F.);
#21163=ORIENTED_EDGE('',*,*,#15580,.F.);
#21164=ORIENTED_EDGE('',*,*,#14816,.F.);
#21165=ORIENTED_EDGE('',*,*,#15580,.T.);
#21166=ORIENTED_EDGE('',*,*,#15431,.F.);
#21167=ORIENTED_EDGE('',*,*,#15581,.F.);
#21168=ORIENTED_EDGE('',*,*,#14817,.F.);
#21169=ORIENTED_EDGE('',*,*,#15581,.T.);
#21170=ORIENTED_EDGE('',*,*,#15430,.F.);
#21171=ORIENTED_EDGE('',*,*,#15582,.F.);
#21172=ORIENTED_EDGE('',*,*,#14818,.F.);
#21173=ORIENTED_EDGE('',*,*,#15582,.T.);
#21174=ORIENTED_EDGE('',*,*,#15429,.F.);
#21175=ORIENTED_EDGE('',*,*,#15583,.F.);
#21176=ORIENTED_EDGE('',*,*,#14819,.F.);
#21177=ORIENTED_EDGE('',*,*,#15583,.T.);
#21178=ORIENTED_EDGE('',*,*,#15428,.F.);
#21179=ORIENTED_EDGE('',*,*,#15584,.F.);
#21180=ORIENTED_EDGE('',*,*,#14820,.F.);
#21181=ORIENTED_EDGE('',*,*,#15584,.T.);
#21182=ORIENTED_EDGE('',*,*,#15427,.F.);
#21183=ORIENTED_EDGE('',*,*,#15585,.F.);
#21184=ORIENTED_EDGE('',*,*,#14821,.F.);
#21185=ORIENTED_EDGE('',*,*,#15585,.T.);
#21186=ORIENTED_EDGE('',*,*,#15426,.F.);
#21187=ORIENTED_EDGE('',*,*,#15586,.F.);
#21188=ORIENTED_EDGE('',*,*,#14822,.F.);
#21189=ORIENTED_EDGE('',*,*,#15586,.T.);
#21190=ORIENTED_EDGE('',*,*,#15425,.F.);
#21191=ORIENTED_EDGE('',*,*,#15587,.F.);
#21192=ORIENTED_EDGE('',*,*,#14823,.F.);
#21193=ORIENTED_EDGE('',*,*,#15587,.T.);
#21194=ORIENTED_EDGE('',*,*,#15424,.F.);
#21195=ORIENTED_EDGE('',*,*,#15588,.F.);
#21196=ORIENTED_EDGE('',*,*,#14824,.F.);
#21197=ORIENTED_EDGE('',*,*,#15588,.T.);
#21198=ORIENTED_EDGE('',*,*,#15423,.F.);
#21199=ORIENTED_EDGE('',*,*,#15589,.F.);
#21200=ORIENTED_EDGE('',*,*,#14825,.F.);
#21201=ORIENTED_EDGE('',*,*,#15589,.T.);
#21202=ORIENTED_EDGE('',*,*,#15422,.F.);
#21203=ORIENTED_EDGE('',*,*,#15590,.F.);
#21204=ORIENTED_EDGE('',*,*,#14826,.F.);
#21205=ORIENTED_EDGE('',*,*,#15590,.T.);
#21206=ORIENTED_EDGE('',*,*,#15421,.F.);
#21207=ORIENTED_EDGE('',*,*,#15591,.F.);
#21208=ORIENTED_EDGE('',*,*,#14827,.F.);
#21209=ORIENTED_EDGE('',*,*,#15591,.T.);
#21210=ORIENTED_EDGE('',*,*,#15420,.F.);
#21211=ORIENTED_EDGE('',*,*,#15592,.F.);
#21212=ORIENTED_EDGE('',*,*,#14828,.F.);
#21213=ORIENTED_EDGE('',*,*,#15592,.T.);
#21214=ORIENTED_EDGE('',*,*,#15419,.F.);
#21215=ORIENTED_EDGE('',*,*,#15593,.F.);
#21216=ORIENTED_EDGE('',*,*,#15213,.F.);
#21217=ORIENTED_EDGE('',*,*,#14829,.F.);
#21218=ORIENTED_EDGE('',*,*,#15593,.T.);
#21219=ORIENTED_EDGE('',*,*,#15418,.F.);
#21220=ORIENTED_EDGE('',*,*,#15484,.F.);
#21221=ORIENTED_EDGE('',*,*,#15594,.F.);
#21222=ORIENTED_EDGE('',*,*,#15214,.F.);
#21223=ORIENTED_EDGE('',*,*,#15594,.T.);
#21224=ORIENTED_EDGE('',*,*,#15486,.F.);
#21225=ORIENTED_EDGE('',*,*,#15218,.F.);
#21226=ORIENTED_EDGE('',*,*,#14831,.F.);
#21227=ORIENTED_EDGE('',*,*,#15212,.F.);
#21228=ORIENTED_EDGE('',*,*,#15217,.T.);
#21229=ORIENTED_EDGE('',*,*,#15485,.F.);
#21230=ORIENTED_EDGE('',*,*,#15416,.F.);
#21231=ORIENTED_EDGE('',*,*,#15595,.F.);
#21232=ORIENTED_EDGE('',*,*,#14832,.F.);
#21233=ORIENTED_EDGE('',*,*,#15595,.T.);
#21234=ORIENTED_EDGE('',*,*,#15415,.F.);
#21235=ORIENTED_EDGE('',*,*,#15489,.F.);
#21236=ORIENTED_EDGE('',*,*,#15596,.F.);
#21237=ORIENTED_EDGE('',*,*,#15077,.F.);
#21238=ORIENTED_EDGE('',*,*,#15078,.F.);
#21239=ORIENTED_EDGE('',*,*,#15596,.T.);
#21240=ORIENTED_EDGE('',*,*,#15488,.F.);
#21241=ORIENTED_EDGE('',*,*,#15597,.F.);
#21242=ORIENTED_EDGE('',*,*,#15079,.F.);
#21243=ORIENTED_EDGE('',*,*,#15597,.T.);
#21244=ORIENTED_EDGE('',*,*,#15487,.F.);
#21245=ORIENTED_EDGE('',*,*,#15085,.F.);
#21246=ORIENTED_EDGE('',*,*,#14835,.F.);
#21247=ORIENTED_EDGE('',*,*,#15084,.T.);
#21248=ORIENTED_EDGE('',*,*,#15413,.F.);
#21249=ORIENTED_EDGE('',*,*,#15598,.F.);
#21250=ORIENTED_EDGE('',*,*,#14836,.F.);
#21251=ORIENTED_EDGE('',*,*,#15598,.T.);
#21252=ORIENTED_EDGE('',*,*,#15412,.F.);
#21253=ORIENTED_EDGE('',*,*,#15599,.F.);
#21254=ORIENTED_EDGE('',*,*,#14837,.F.);
#21255=ORIENTED_EDGE('',*,*,#15599,.T.);
#21256=ORIENTED_EDGE('',*,*,#15411,.F.);
#21257=ORIENTED_EDGE('',*,*,#15600,.F.);
#21258=ORIENTED_EDGE('',*,*,#14838,.F.);
#21259=ORIENTED_EDGE('',*,*,#15600,.T.);
#21260=ORIENTED_EDGE('',*,*,#15410,.F.);
#21261=ORIENTED_EDGE('',*,*,#15601,.F.);
#21262=ORIENTED_EDGE('',*,*,#14839,.F.);
#21263=ORIENTED_EDGE('',*,*,#15601,.T.);
#21264=ORIENTED_EDGE('',*,*,#15409,.F.);
#21265=ORIENTED_EDGE('',*,*,#15602,.F.);
#21266=ORIENTED_EDGE('',*,*,#14840,.F.);
#21267=ORIENTED_EDGE('',*,*,#15602,.T.);
#21268=ORIENTED_EDGE('',*,*,#15408,.F.);
#21269=ORIENTED_EDGE('',*,*,#15603,.F.);
#21270=ORIENTED_EDGE('',*,*,#14841,.F.);
#21271=ORIENTED_EDGE('',*,*,#15603,.T.);
#21272=ORIENTED_EDGE('',*,*,#15407,.F.);
#21273=ORIENTED_EDGE('',*,*,#15604,.F.);
#21274=ORIENTED_EDGE('',*,*,#14842,.F.);
#21275=ORIENTED_EDGE('',*,*,#15604,.T.);
#21276=ORIENTED_EDGE('',*,*,#15406,.F.);
#21277=ORIENTED_EDGE('',*,*,#15605,.F.);
#21278=ORIENTED_EDGE('',*,*,#14843,.F.);
#21279=ORIENTED_EDGE('',*,*,#15605,.T.);
#21280=ORIENTED_EDGE('',*,*,#15405,.F.);
#21281=ORIENTED_EDGE('',*,*,#15606,.F.);
#21282=ORIENTED_EDGE('',*,*,#14844,.F.);
#21283=ORIENTED_EDGE('',*,*,#15606,.T.);
#21284=ORIENTED_EDGE('',*,*,#15404,.F.);
#21285=ORIENTED_EDGE('',*,*,#15607,.F.);
#21286=ORIENTED_EDGE('',*,*,#14845,.F.);
#21287=ORIENTED_EDGE('',*,*,#15607,.T.);
#21288=ORIENTED_EDGE('',*,*,#15403,.F.);
#21289=ORIENTED_EDGE('',*,*,#15608,.F.);
#21290=ORIENTED_EDGE('',*,*,#14846,.F.);
#21291=ORIENTED_EDGE('',*,*,#15608,.T.);
#21292=ORIENTED_EDGE('',*,*,#15402,.F.);
#21293=ORIENTED_EDGE('',*,*,#15609,.F.);
#21294=ORIENTED_EDGE('',*,*,#14847,.F.);
#21295=ORIENTED_EDGE('',*,*,#15609,.T.);
#21296=ORIENTED_EDGE('',*,*,#15401,.F.);
#21297=ORIENTED_EDGE('',*,*,#15610,.F.);
#21298=ORIENTED_EDGE('',*,*,#14848,.F.);
#21299=ORIENTED_EDGE('',*,*,#15610,.T.);
#21300=ORIENTED_EDGE('',*,*,#15400,.F.);
#21301=ORIENTED_EDGE('',*,*,#15611,.F.);
#21302=ORIENTED_EDGE('',*,*,#15203,.F.);
#21303=ORIENTED_EDGE('',*,*,#14849,.F.);
#21304=ORIENTED_EDGE('',*,*,#15611,.T.);
#21305=ORIENTED_EDGE('',*,*,#15399,.F.);
#21306=ORIENTED_EDGE('',*,*,#15490,.F.);
#21307=ORIENTED_EDGE('',*,*,#15612,.F.);
#21308=ORIENTED_EDGE('',*,*,#15204,.F.);
#21309=ORIENTED_EDGE('',*,*,#15612,.T.);
#21310=ORIENTED_EDGE('',*,*,#15492,.F.);
#21311=ORIENTED_EDGE('',*,*,#15208,.F.);
#21312=ORIENTED_EDGE('',*,*,#14851,.F.);
#21313=ORIENTED_EDGE('',*,*,#15202,.F.);
#21314=ORIENTED_EDGE('',*,*,#15207,.T.);
#21315=ORIENTED_EDGE('',*,*,#15491,.F.);
#21316=ORIENTED_EDGE('',*,*,#15397,.F.);
#21317=ORIENTED_EDGE('',*,*,#15613,.F.);
#21318=ORIENTED_EDGE('',*,*,#14852,.F.);
#21319=ORIENTED_EDGE('',*,*,#15613,.T.);
#21320=ORIENTED_EDGE('',*,*,#15396,.F.);
#21321=ORIENTED_EDGE('',*,*,#15495,.F.);
#21322=ORIENTED_EDGE('',*,*,#15614,.F.);
#21323=ORIENTED_EDGE('',*,*,#15066,.F.);
#21324=ORIENTED_EDGE('',*,*,#15067,.F.);
#21325=ORIENTED_EDGE('',*,*,#15614,.T.);
#21326=ORIENTED_EDGE('',*,*,#15494,.F.);
#21327=ORIENTED_EDGE('',*,*,#15615,.F.);
#21328=ORIENTED_EDGE('',*,*,#15068,.F.);
#21329=ORIENTED_EDGE('',*,*,#15615,.T.);
#21330=ORIENTED_EDGE('',*,*,#15493,.F.);
#21331=ORIENTED_EDGE('',*,*,#15074,.F.);
#21332=ORIENTED_EDGE('',*,*,#14855,.F.);
#21333=ORIENTED_EDGE('',*,*,#15073,.T.);
#21334=ORIENTED_EDGE('',*,*,#15394,.F.);
#21335=ORIENTED_EDGE('',*,*,#15616,.F.);
#21336=ORIENTED_EDGE('',*,*,#14856,.F.);
#21337=ORIENTED_EDGE('',*,*,#15616,.T.);
#21338=ORIENTED_EDGE('',*,*,#15393,.F.);
#21339=ORIENTED_EDGE('',*,*,#15617,.F.);
#21340=ORIENTED_EDGE('',*,*,#14857,.F.);
#21341=ORIENTED_EDGE('',*,*,#15617,.T.);
#21342=ORIENTED_EDGE('',*,*,#15392,.F.);
#21343=ORIENTED_EDGE('',*,*,#15618,.F.);
#21344=ORIENTED_EDGE('',*,*,#14858,.F.);
#21345=ORIENTED_EDGE('',*,*,#15618,.T.);
#21346=ORIENTED_EDGE('',*,*,#15391,.F.);
#21347=ORIENTED_EDGE('',*,*,#15619,.F.);
#21348=ORIENTED_EDGE('',*,*,#14859,.F.);
#21349=ORIENTED_EDGE('',*,*,#15619,.T.);
#21350=ORIENTED_EDGE('',*,*,#15390,.F.);
#21351=ORIENTED_EDGE('',*,*,#15620,.F.);
#21352=ORIENTED_EDGE('',*,*,#14860,.F.);
#21353=ORIENTED_EDGE('',*,*,#15620,.T.);
#21354=ORIENTED_EDGE('',*,*,#15389,.F.);
#21355=ORIENTED_EDGE('',*,*,#15621,.F.);
#21356=ORIENTED_EDGE('',*,*,#14861,.F.);
#21357=ORIENTED_EDGE('',*,*,#15621,.T.);
#21358=ORIENTED_EDGE('',*,*,#15388,.F.);
#21359=ORIENTED_EDGE('',*,*,#15622,.F.);
#21360=ORIENTED_EDGE('',*,*,#14862,.F.);
#21361=ORIENTED_EDGE('',*,*,#15622,.T.);
#21362=ORIENTED_EDGE('',*,*,#15387,.F.);
#21363=ORIENTED_EDGE('',*,*,#15623,.F.);
#21364=ORIENTED_EDGE('',*,*,#14863,.F.);
#21365=ORIENTED_EDGE('',*,*,#15623,.T.);
#21366=ORIENTED_EDGE('',*,*,#15386,.F.);
#21367=ORIENTED_EDGE('',*,*,#15624,.F.);
#21368=ORIENTED_EDGE('',*,*,#14864,.F.);
#21369=ORIENTED_EDGE('',*,*,#15624,.T.);
#21370=ORIENTED_EDGE('',*,*,#15385,.F.);
#21371=ORIENTED_EDGE('',*,*,#15625,.F.);
#21372=ORIENTED_EDGE('',*,*,#14865,.F.);
#21373=ORIENTED_EDGE('',*,*,#15625,.T.);
#21374=ORIENTED_EDGE('',*,*,#15384,.F.);
#21375=ORIENTED_EDGE('',*,*,#15626,.F.);
#21376=ORIENTED_EDGE('',*,*,#14866,.F.);
#21377=ORIENTED_EDGE('',*,*,#15626,.T.);
#21378=ORIENTED_EDGE('',*,*,#15383,.F.);
#21379=ORIENTED_EDGE('',*,*,#15627,.F.);
#21380=ORIENTED_EDGE('',*,*,#14867,.F.);
#21381=ORIENTED_EDGE('',*,*,#15627,.T.);
#21382=ORIENTED_EDGE('',*,*,#15382,.F.);
#21383=ORIENTED_EDGE('',*,*,#15628,.F.);
#21384=ORIENTED_EDGE('',*,*,#14868,.F.);
#21385=ORIENTED_EDGE('',*,*,#15628,.T.);
#21386=ORIENTED_EDGE('',*,*,#15381,.F.);
#21387=ORIENTED_EDGE('',*,*,#15629,.F.);
#21388=ORIENTED_EDGE('',*,*,#15193,.F.);
#21389=ORIENTED_EDGE('',*,*,#14869,.F.);
#21390=ORIENTED_EDGE('',*,*,#15629,.T.);
#21391=ORIENTED_EDGE('',*,*,#15380,.F.);
#21392=ORIENTED_EDGE('',*,*,#15496,.F.);
#21393=ORIENTED_EDGE('',*,*,#15630,.F.);
#21394=ORIENTED_EDGE('',*,*,#15194,.F.);
#21395=ORIENTED_EDGE('',*,*,#15630,.T.);
#21396=ORIENTED_EDGE('',*,*,#15498,.F.);
#21397=ORIENTED_EDGE('',*,*,#15198,.F.);
#21398=ORIENTED_EDGE('',*,*,#14871,.F.);
#21399=ORIENTED_EDGE('',*,*,#15192,.F.);
#21400=ORIENTED_EDGE('',*,*,#15197,.T.);
#21401=ORIENTED_EDGE('',*,*,#15497,.F.);
#21402=ORIENTED_EDGE('',*,*,#15378,.F.);
#21403=ORIENTED_EDGE('',*,*,#15631,.F.);
#21404=ORIENTED_EDGE('',*,*,#14872,.F.);
#21405=ORIENTED_EDGE('',*,*,#15631,.T.);
#21406=ORIENTED_EDGE('',*,*,#15377,.F.);
#21407=ORIENTED_EDGE('',*,*,#15501,.F.);
#21408=ORIENTED_EDGE('',*,*,#15632,.F.);
#21409=ORIENTED_EDGE('',*,*,#15055,.F.);
#21410=ORIENTED_EDGE('',*,*,#15056,.F.);
#21411=ORIENTED_EDGE('',*,*,#15632,.T.);
#21412=ORIENTED_EDGE('',*,*,#15500,.F.);
#21413=ORIENTED_EDGE('',*,*,#15633,.F.);
#21414=ORIENTED_EDGE('',*,*,#15057,.F.);
#21415=ORIENTED_EDGE('',*,*,#15633,.T.);
#21416=ORIENTED_EDGE('',*,*,#15499,.F.);
#21417=ORIENTED_EDGE('',*,*,#15063,.F.);
#21418=ORIENTED_EDGE('',*,*,#14875,.F.);
#21419=ORIENTED_EDGE('',*,*,#15062,.T.);
#21420=ORIENTED_EDGE('',*,*,#15375,.F.);
#21421=ORIENTED_EDGE('',*,*,#15634,.F.);
#21422=ORIENTED_EDGE('',*,*,#14876,.F.);
#21423=ORIENTED_EDGE('',*,*,#15634,.T.);
#21424=ORIENTED_EDGE('',*,*,#15374,.F.);
#21425=ORIENTED_EDGE('',*,*,#15635,.F.);
#21426=ORIENTED_EDGE('',*,*,#14877,.F.);
#21427=ORIENTED_EDGE('',*,*,#15635,.T.);
#21428=ORIENTED_EDGE('',*,*,#15373,.F.);
#21429=ORIENTED_EDGE('',*,*,#15636,.F.);
#21430=ORIENTED_EDGE('',*,*,#14878,.F.);
#21431=ORIENTED_EDGE('',*,*,#15636,.T.);
#21432=ORIENTED_EDGE('',*,*,#15372,.F.);
#21433=ORIENTED_EDGE('',*,*,#15637,.F.);
#21434=ORIENTED_EDGE('',*,*,#14879,.F.);
#21435=ORIENTED_EDGE('',*,*,#15637,.T.);
#21436=ORIENTED_EDGE('',*,*,#15371,.F.);
#21437=ORIENTED_EDGE('',*,*,#15638,.F.);
#21438=ORIENTED_EDGE('',*,*,#14880,.F.);
#21439=ORIENTED_EDGE('',*,*,#15638,.T.);
#21440=ORIENTED_EDGE('',*,*,#15370,.F.);
#21441=ORIENTED_EDGE('',*,*,#15639,.F.);
#21442=ORIENTED_EDGE('',*,*,#14881,.F.);
#21443=ORIENTED_EDGE('',*,*,#15639,.T.);
#21444=ORIENTED_EDGE('',*,*,#15369,.F.);
#21445=ORIENTED_EDGE('',*,*,#15640,.F.);
#21446=ORIENTED_EDGE('',*,*,#14882,.F.);
#21447=ORIENTED_EDGE('',*,*,#15640,.T.);
#21448=ORIENTED_EDGE('',*,*,#15368,.F.);
#21449=ORIENTED_EDGE('',*,*,#15641,.F.);
#21450=ORIENTED_EDGE('',*,*,#14883,.F.);
#21451=ORIENTED_EDGE('',*,*,#15641,.T.);
#21452=ORIENTED_EDGE('',*,*,#15367,.F.);
#21453=ORIENTED_EDGE('',*,*,#15642,.F.);
#21454=ORIENTED_EDGE('',*,*,#14884,.F.);
#21455=ORIENTED_EDGE('',*,*,#15642,.T.);
#21456=ORIENTED_EDGE('',*,*,#15366,.F.);
#21457=ORIENTED_EDGE('',*,*,#15643,.F.);
#21458=ORIENTED_EDGE('',*,*,#14885,.F.);
#21459=ORIENTED_EDGE('',*,*,#15643,.T.);
#21460=ORIENTED_EDGE('',*,*,#15365,.F.);
#21461=ORIENTED_EDGE('',*,*,#15644,.F.);
#21462=ORIENTED_EDGE('',*,*,#14886,.F.);
#21463=ORIENTED_EDGE('',*,*,#15644,.T.);
#21464=ORIENTED_EDGE('',*,*,#15364,.F.);
#21465=ORIENTED_EDGE('',*,*,#15645,.F.);
#21466=ORIENTED_EDGE('',*,*,#14887,.F.);
#21467=ORIENTED_EDGE('',*,*,#15645,.T.);
#21468=ORIENTED_EDGE('',*,*,#15363,.F.);
#21469=ORIENTED_EDGE('',*,*,#15646,.F.);
#21470=ORIENTED_EDGE('',*,*,#14888,.F.);
#21471=ORIENTED_EDGE('',*,*,#15646,.T.);
#21472=ORIENTED_EDGE('',*,*,#15362,.F.);
#21473=ORIENTED_EDGE('',*,*,#15647,.F.);
#21474=ORIENTED_EDGE('',*,*,#15183,.F.);
#21475=ORIENTED_EDGE('',*,*,#14889,.F.);
#21476=ORIENTED_EDGE('',*,*,#15647,.T.);
#21477=ORIENTED_EDGE('',*,*,#15361,.F.);
#21478=ORIENTED_EDGE('',*,*,#15502,.F.);
#21479=ORIENTED_EDGE('',*,*,#15648,.F.);
#21480=ORIENTED_EDGE('',*,*,#15184,.F.);
#21481=ORIENTED_EDGE('',*,*,#15648,.T.);
#21482=ORIENTED_EDGE('',*,*,#15504,.F.);
#21483=ORIENTED_EDGE('',*,*,#15188,.F.);
#21484=ORIENTED_EDGE('',*,*,#14891,.F.);
#21485=ORIENTED_EDGE('',*,*,#15182,.F.);
#21486=ORIENTED_EDGE('',*,*,#15187,.T.);
#21487=ORIENTED_EDGE('',*,*,#15503,.F.);
#21488=ORIENTED_EDGE('',*,*,#15359,.F.);
#21489=ORIENTED_EDGE('',*,*,#15649,.F.);
#21490=ORIENTED_EDGE('',*,*,#14892,.F.);
#21491=ORIENTED_EDGE('',*,*,#15649,.T.);
#21492=ORIENTED_EDGE('',*,*,#15358,.F.);
#21493=ORIENTED_EDGE('',*,*,#15507,.F.);
#21494=ORIENTED_EDGE('',*,*,#15650,.F.);
#21495=ORIENTED_EDGE('',*,*,#15044,.F.);
#21496=ORIENTED_EDGE('',*,*,#15045,.F.);
#21497=ORIENTED_EDGE('',*,*,#15650,.T.);
#21498=ORIENTED_EDGE('',*,*,#15506,.F.);
#21499=ORIENTED_EDGE('',*,*,#15651,.F.);
#21500=ORIENTED_EDGE('',*,*,#15046,.F.);
#21501=ORIENTED_EDGE('',*,*,#15651,.T.);
#21502=ORIENTED_EDGE('',*,*,#15505,.F.);
#21503=ORIENTED_EDGE('',*,*,#15052,.F.);
#21504=ORIENTED_EDGE('',*,*,#14895,.F.);
#21505=ORIENTED_EDGE('',*,*,#15051,.T.);
#21506=ORIENTED_EDGE('',*,*,#15356,.F.);
#21507=ORIENTED_EDGE('',*,*,#15652,.F.);
#21508=ORIENTED_EDGE('',*,*,#14896,.F.);
#21509=ORIENTED_EDGE('',*,*,#15652,.T.);
#21510=ORIENTED_EDGE('',*,*,#15355,.F.);
#21511=ORIENTED_EDGE('',*,*,#15653,.F.);
#21512=ORIENTED_EDGE('',*,*,#14897,.F.);
#21513=ORIENTED_EDGE('',*,*,#15653,.T.);
#21514=ORIENTED_EDGE('',*,*,#15354,.F.);
#21515=ORIENTED_EDGE('',*,*,#15654,.F.);
#21516=ORIENTED_EDGE('',*,*,#14898,.F.);
#21517=ORIENTED_EDGE('',*,*,#15654,.T.);
#21518=ORIENTED_EDGE('',*,*,#15353,.F.);
#21519=ORIENTED_EDGE('',*,*,#15655,.F.);
#21520=ORIENTED_EDGE('',*,*,#14899,.F.);
#21521=ORIENTED_EDGE('',*,*,#15655,.T.);
#21522=ORIENTED_EDGE('',*,*,#15352,.F.);
#21523=ORIENTED_EDGE('',*,*,#15656,.F.);
#21524=ORIENTED_EDGE('',*,*,#14900,.F.);
#21525=ORIENTED_EDGE('',*,*,#15656,.T.);
#21526=ORIENTED_EDGE('',*,*,#15351,.F.);
#21527=ORIENTED_EDGE('',*,*,#15657,.F.);
#21528=ORIENTED_EDGE('',*,*,#14901,.F.);
#21529=ORIENTED_EDGE('',*,*,#15657,.T.);
#21530=ORIENTED_EDGE('',*,*,#15350,.F.);
#21531=ORIENTED_EDGE('',*,*,#15658,.F.);
#21532=ORIENTED_EDGE('',*,*,#14902,.F.);
#21533=ORIENTED_EDGE('',*,*,#15658,.T.);
#21534=ORIENTED_EDGE('',*,*,#15349,.F.);
#21535=ORIENTED_EDGE('',*,*,#15659,.F.);
#21536=ORIENTED_EDGE('',*,*,#14903,.F.);
#21537=ORIENTED_EDGE('',*,*,#15659,.T.);
#21538=ORIENTED_EDGE('',*,*,#15348,.F.);
#21539=ORIENTED_EDGE('',*,*,#15660,.F.);
#21540=ORIENTED_EDGE('',*,*,#14904,.F.);
#21541=ORIENTED_EDGE('',*,*,#15660,.T.);
#21542=ORIENTED_EDGE('',*,*,#15347,.F.);
#21543=ORIENTED_EDGE('',*,*,#15661,.F.);
#21544=ORIENTED_EDGE('',*,*,#14905,.F.);
#21545=ORIENTED_EDGE('',*,*,#15661,.T.);
#21546=ORIENTED_EDGE('',*,*,#15346,.F.);
#21547=ORIENTED_EDGE('',*,*,#15662,.F.);
#21548=ORIENTED_EDGE('',*,*,#14906,.F.);
#21549=ORIENTED_EDGE('',*,*,#15662,.T.);
#21550=ORIENTED_EDGE('',*,*,#15345,.F.);
#21551=ORIENTED_EDGE('',*,*,#15663,.F.);
#21552=ORIENTED_EDGE('',*,*,#14907,.F.);
#21553=ORIENTED_EDGE('',*,*,#15663,.T.);
#21554=ORIENTED_EDGE('',*,*,#15344,.F.);
#21555=ORIENTED_EDGE('',*,*,#15664,.F.);
#21556=ORIENTED_EDGE('',*,*,#14908,.F.);
#21557=ORIENTED_EDGE('',*,*,#15664,.T.);
#21558=ORIENTED_EDGE('',*,*,#15343,.F.);
#21559=ORIENTED_EDGE('',*,*,#15665,.F.);
#21560=ORIENTED_EDGE('',*,*,#15173,.F.);
#21561=ORIENTED_EDGE('',*,*,#14909,.F.);
#21562=ORIENTED_EDGE('',*,*,#15665,.T.);
#21563=ORIENTED_EDGE('',*,*,#15342,.F.);
#21564=ORIENTED_EDGE('',*,*,#15508,.F.);
#21565=ORIENTED_EDGE('',*,*,#15666,.F.);
#21566=ORIENTED_EDGE('',*,*,#15174,.F.);
#21567=ORIENTED_EDGE('',*,*,#15666,.T.);
#21568=ORIENTED_EDGE('',*,*,#15510,.F.);
#21569=ORIENTED_EDGE('',*,*,#15178,.F.);
#21570=ORIENTED_EDGE('',*,*,#14911,.F.);
#21571=ORIENTED_EDGE('',*,*,#15172,.F.);
#21572=ORIENTED_EDGE('',*,*,#15177,.T.);
#21573=ORIENTED_EDGE('',*,*,#15509,.F.);
#21574=ORIENTED_EDGE('',*,*,#15340,.F.);
#21575=ORIENTED_EDGE('',*,*,#15667,.F.);
#21576=ORIENTED_EDGE('',*,*,#14912,.F.);
#21577=ORIENTED_EDGE('',*,*,#15667,.T.);
#21578=ORIENTED_EDGE('',*,*,#15339,.F.);
#21579=ORIENTED_EDGE('',*,*,#15513,.F.);
#21580=ORIENTED_EDGE('',*,*,#15668,.F.);
#21581=ORIENTED_EDGE('',*,*,#15033,.F.);
#21582=ORIENTED_EDGE('',*,*,#15034,.F.);
#21583=ORIENTED_EDGE('',*,*,#15668,.T.);
#21584=ORIENTED_EDGE('',*,*,#15512,.F.);
#21585=ORIENTED_EDGE('',*,*,#15669,.F.);
#21586=ORIENTED_EDGE('',*,*,#15035,.F.);
#21587=ORIENTED_EDGE('',*,*,#15669,.T.);
#21588=ORIENTED_EDGE('',*,*,#15511,.F.);
#21589=ORIENTED_EDGE('',*,*,#15041,.F.);
#21590=ORIENTED_EDGE('',*,*,#14915,.F.);
#21591=ORIENTED_EDGE('',*,*,#15040,.T.);
#21592=ORIENTED_EDGE('',*,*,#15337,.F.);
#21593=ORIENTED_EDGE('',*,*,#15670,.F.);
#21594=ORIENTED_EDGE('',*,*,#14916,.F.);
#21595=ORIENTED_EDGE('',*,*,#15670,.T.);
#21596=ORIENTED_EDGE('',*,*,#15336,.F.);
#21597=ORIENTED_EDGE('',*,*,#15671,.F.);
#21598=ORIENTED_EDGE('',*,*,#14917,.F.);
#21599=ORIENTED_EDGE('',*,*,#15671,.T.);
#21600=ORIENTED_EDGE('',*,*,#15335,.F.);
#21601=ORIENTED_EDGE('',*,*,#15672,.F.);
#21602=ORIENTED_EDGE('',*,*,#14918,.F.);
#21603=ORIENTED_EDGE('',*,*,#15672,.T.);
#21604=ORIENTED_EDGE('',*,*,#15334,.F.);
#21605=ORIENTED_EDGE('',*,*,#15673,.F.);
#21606=ORIENTED_EDGE('',*,*,#14919,.F.);
#21607=ORIENTED_EDGE('',*,*,#15673,.T.);
#21608=ORIENTED_EDGE('',*,*,#15333,.F.);
#21609=ORIENTED_EDGE('',*,*,#15674,.F.);
#21610=ORIENTED_EDGE('',*,*,#14920,.F.);
#21611=ORIENTED_EDGE('',*,*,#15674,.T.);
#21612=ORIENTED_EDGE('',*,*,#15332,.F.);
#21613=ORIENTED_EDGE('',*,*,#15675,.F.);
#21614=ORIENTED_EDGE('',*,*,#14921,.F.);
#21615=ORIENTED_EDGE('',*,*,#15675,.T.);
#21616=ORIENTED_EDGE('',*,*,#15331,.F.);
#21617=ORIENTED_EDGE('',*,*,#15676,.F.);
#21618=ORIENTED_EDGE('',*,*,#14922,.F.);
#21619=ORIENTED_EDGE('',*,*,#15676,.T.);
#21620=ORIENTED_EDGE('',*,*,#15330,.F.);
#21621=ORIENTED_EDGE('',*,*,#15677,.F.);
#21622=ORIENTED_EDGE('',*,*,#14923,.F.);
#21623=ORIENTED_EDGE('',*,*,#15677,.T.);
#21624=ORIENTED_EDGE('',*,*,#15329,.F.);
#21625=ORIENTED_EDGE('',*,*,#15678,.F.);
#21626=ORIENTED_EDGE('',*,*,#14924,.F.);
#21627=ORIENTED_EDGE('',*,*,#15678,.T.);
#21628=ORIENTED_EDGE('',*,*,#15328,.F.);
#21629=ORIENTED_EDGE('',*,*,#15679,.F.);
#21630=ORIENTED_EDGE('',*,*,#14925,.F.);
#21631=ORIENTED_EDGE('',*,*,#15679,.T.);
#21632=ORIENTED_EDGE('',*,*,#15327,.F.);
#21633=ORIENTED_EDGE('',*,*,#15680,.F.);
#21634=ORIENTED_EDGE('',*,*,#14926,.F.);
#21635=ORIENTED_EDGE('',*,*,#15680,.T.);
#21636=ORIENTED_EDGE('',*,*,#15326,.F.);
#21637=ORIENTED_EDGE('',*,*,#15681,.F.);
#21638=ORIENTED_EDGE('',*,*,#14927,.F.);
#21639=ORIENTED_EDGE('',*,*,#15681,.T.);
#21640=ORIENTED_EDGE('',*,*,#15325,.F.);
#21641=ORIENTED_EDGE('',*,*,#15682,.F.);
#21642=ORIENTED_EDGE('',*,*,#14928,.F.);
#21643=ORIENTED_EDGE('',*,*,#15682,.T.);
#21644=ORIENTED_EDGE('',*,*,#15324,.F.);
#21645=ORIENTED_EDGE('',*,*,#15683,.F.);
#21646=ORIENTED_EDGE('',*,*,#15163,.F.);
#21647=ORIENTED_EDGE('',*,*,#14929,.F.);
#21648=ORIENTED_EDGE('',*,*,#15683,.T.);
#21649=ORIENTED_EDGE('',*,*,#15323,.F.);
#21650=ORIENTED_EDGE('',*,*,#15514,.F.);
#21651=ORIENTED_EDGE('',*,*,#15684,.F.);
#21652=ORIENTED_EDGE('',*,*,#15164,.F.);
#21653=ORIENTED_EDGE('',*,*,#15684,.T.);
#21654=ORIENTED_EDGE('',*,*,#15516,.F.);
#21655=ORIENTED_EDGE('',*,*,#15168,.F.);
#21656=ORIENTED_EDGE('',*,*,#14931,.F.);
#21657=ORIENTED_EDGE('',*,*,#15162,.F.);
#21658=ORIENTED_EDGE('',*,*,#15167,.T.);
#21659=ORIENTED_EDGE('',*,*,#15515,.F.);
#21660=ORIENTED_EDGE('',*,*,#15321,.F.);
#21661=ORIENTED_EDGE('',*,*,#15685,.F.);
#21662=ORIENTED_EDGE('',*,*,#14932,.F.);
#21663=ORIENTED_EDGE('',*,*,#15685,.T.);
#21664=ORIENTED_EDGE('',*,*,#15320,.F.);
#21665=ORIENTED_EDGE('',*,*,#15519,.F.);
#21666=ORIENTED_EDGE('',*,*,#15686,.F.);
#21667=ORIENTED_EDGE('',*,*,#15022,.F.);
#21668=ORIENTED_EDGE('',*,*,#15023,.F.);
#21669=ORIENTED_EDGE('',*,*,#15686,.T.);
#21670=ORIENTED_EDGE('',*,*,#15518,.F.);
#21671=ORIENTED_EDGE('',*,*,#15687,.F.);
#21672=ORIENTED_EDGE('',*,*,#15024,.F.);
#21673=ORIENTED_EDGE('',*,*,#15687,.T.);
#21674=ORIENTED_EDGE('',*,*,#15517,.F.);
#21675=ORIENTED_EDGE('',*,*,#15030,.F.);
#21676=ORIENTED_EDGE('',*,*,#14935,.F.);
#21677=ORIENTED_EDGE('',*,*,#15029,.T.);
#21678=ORIENTED_EDGE('',*,*,#15318,.F.);
#21679=ORIENTED_EDGE('',*,*,#15688,.F.);
#21680=ORIENTED_EDGE('',*,*,#14936,.F.);
#21681=ORIENTED_EDGE('',*,*,#15688,.T.);
#21682=ORIENTED_EDGE('',*,*,#15317,.F.);
#21683=ORIENTED_EDGE('',*,*,#15689,.F.);
#21684=ORIENTED_EDGE('',*,*,#14937,.F.);
#21685=ORIENTED_EDGE('',*,*,#15689,.T.);
#21686=ORIENTED_EDGE('',*,*,#15316,.F.);
#21687=ORIENTED_EDGE('',*,*,#15690,.F.);
#21688=ORIENTED_EDGE('',*,*,#14938,.F.);
#21689=ORIENTED_EDGE('',*,*,#15690,.T.);
#21690=ORIENTED_EDGE('',*,*,#15315,.F.);
#21691=ORIENTED_EDGE('',*,*,#15691,.F.);
#21692=ORIENTED_EDGE('',*,*,#14939,.F.);
#21693=ORIENTED_EDGE('',*,*,#15691,.T.);
#21694=ORIENTED_EDGE('',*,*,#15314,.F.);
#21695=ORIENTED_EDGE('',*,*,#15692,.F.);
#21696=ORIENTED_EDGE('',*,*,#14940,.F.);
#21697=ORIENTED_EDGE('',*,*,#15692,.T.);
#21698=ORIENTED_EDGE('',*,*,#15313,.F.);
#21699=ORIENTED_EDGE('',*,*,#15693,.F.);
#21700=ORIENTED_EDGE('',*,*,#14941,.F.);
#21701=ORIENTED_EDGE('',*,*,#15693,.T.);
#21702=ORIENTED_EDGE('',*,*,#15312,.F.);
#21703=ORIENTED_EDGE('',*,*,#15694,.F.);
#21704=ORIENTED_EDGE('',*,*,#14942,.F.);
#21705=ORIENTED_EDGE('',*,*,#15694,.T.);
#21706=ORIENTED_EDGE('',*,*,#15311,.F.);
#21707=ORIENTED_EDGE('',*,*,#15695,.F.);
#21708=ORIENTED_EDGE('',*,*,#14943,.F.);
#21709=ORIENTED_EDGE('',*,*,#15695,.T.);
#21710=ORIENTED_EDGE('',*,*,#15310,.F.);
#21711=ORIENTED_EDGE('',*,*,#15696,.F.);
#21712=ORIENTED_EDGE('',*,*,#14944,.F.);
#21713=ORIENTED_EDGE('',*,*,#15696,.T.);
#21714=ORIENTED_EDGE('',*,*,#15309,.F.);
#21715=ORIENTED_EDGE('',*,*,#15697,.F.);
#21716=ORIENTED_EDGE('',*,*,#14945,.F.);
#21717=ORIENTED_EDGE('',*,*,#15697,.T.);
#21718=ORIENTED_EDGE('',*,*,#15308,.F.);
#21719=ORIENTED_EDGE('',*,*,#15698,.F.);
#21720=ORIENTED_EDGE('',*,*,#14946,.F.);
#21721=ORIENTED_EDGE('',*,*,#15698,.T.);
#21722=ORIENTED_EDGE('',*,*,#15307,.F.);
#21723=ORIENTED_EDGE('',*,*,#15699,.F.);
#21724=ORIENTED_EDGE('',*,*,#14947,.F.);
#21725=ORIENTED_EDGE('',*,*,#15699,.T.);
#21726=ORIENTED_EDGE('',*,*,#15306,.F.);
#21727=ORIENTED_EDGE('',*,*,#15700,.F.);
#21728=ORIENTED_EDGE('',*,*,#14948,.F.);
#21729=ORIENTED_EDGE('',*,*,#15700,.T.);
#21730=ORIENTED_EDGE('',*,*,#15305,.F.);
#21731=ORIENTED_EDGE('',*,*,#15701,.F.);
#21732=ORIENTED_EDGE('',*,*,#15153,.F.);
#21733=ORIENTED_EDGE('',*,*,#14949,.F.);
#21734=ORIENTED_EDGE('',*,*,#15701,.T.);
#21735=ORIENTED_EDGE('',*,*,#15304,.F.);
#21736=ORIENTED_EDGE('',*,*,#15520,.F.);
#21737=ORIENTED_EDGE('',*,*,#15702,.F.);
#21738=ORIENTED_EDGE('',*,*,#15154,.F.);
#21739=ORIENTED_EDGE('',*,*,#15702,.T.);
#21740=ORIENTED_EDGE('',*,*,#15522,.F.);
#21741=ORIENTED_EDGE('',*,*,#15158,.F.);
#21742=ORIENTED_EDGE('',*,*,#14951,.F.);
#21743=ORIENTED_EDGE('',*,*,#15152,.F.);
#21744=ORIENTED_EDGE('',*,*,#15157,.T.);
#21745=ORIENTED_EDGE('',*,*,#15521,.F.);
#21746=ORIENTED_EDGE('',*,*,#15302,.F.);
#21747=ORIENTED_EDGE('',*,*,#15703,.F.);
#21748=ORIENTED_EDGE('',*,*,#14952,.F.);
#21749=ORIENTED_EDGE('',*,*,#15703,.T.);
#21750=ORIENTED_EDGE('',*,*,#15301,.F.);
#21751=ORIENTED_EDGE('',*,*,#15525,.F.);
#21752=ORIENTED_EDGE('',*,*,#15704,.F.);
#21753=ORIENTED_EDGE('',*,*,#15011,.F.);
#21754=ORIENTED_EDGE('',*,*,#15012,.F.);
#21755=ORIENTED_EDGE('',*,*,#15704,.T.);
#21756=ORIENTED_EDGE('',*,*,#15524,.F.);
#21757=ORIENTED_EDGE('',*,*,#15705,.F.);
#21758=ORIENTED_EDGE('',*,*,#15013,.F.);
#21759=ORIENTED_EDGE('',*,*,#15705,.T.);
#21760=ORIENTED_EDGE('',*,*,#15523,.F.);
#21761=ORIENTED_EDGE('',*,*,#15019,.F.);
#21762=ORIENTED_EDGE('',*,*,#14955,.F.);
#21763=ORIENTED_EDGE('',*,*,#15018,.T.);
#21764=ORIENTED_EDGE('',*,*,#15299,.F.);
#21765=ORIENTED_EDGE('',*,*,#15706,.F.);
#21766=ORIENTED_EDGE('',*,*,#14956,.F.);
#21767=ORIENTED_EDGE('',*,*,#15706,.T.);
#21768=ORIENTED_EDGE('',*,*,#15298,.F.);
#21769=ORIENTED_EDGE('',*,*,#15707,.F.);
#21770=ORIENTED_EDGE('',*,*,#14957,.F.);
#21771=ORIENTED_EDGE('',*,*,#15707,.T.);
#21772=ORIENTED_EDGE('',*,*,#15297,.F.);
#21773=ORIENTED_EDGE('',*,*,#15708,.F.);
#21774=ORIENTED_EDGE('',*,*,#14958,.F.);
#21775=ORIENTED_EDGE('',*,*,#15708,.T.);
#21776=ORIENTED_EDGE('',*,*,#15296,.F.);
#21777=ORIENTED_EDGE('',*,*,#15709,.F.);
#21778=ORIENTED_EDGE('',*,*,#14959,.F.);
#21779=ORIENTED_EDGE('',*,*,#15709,.T.);
#21780=ORIENTED_EDGE('',*,*,#15295,.F.);
#21781=ORIENTED_EDGE('',*,*,#15710,.F.);
#21782=ORIENTED_EDGE('',*,*,#14960,.F.);
#21783=ORIENTED_EDGE('',*,*,#15710,.T.);
#21784=ORIENTED_EDGE('',*,*,#15294,.F.);
#21785=ORIENTED_EDGE('',*,*,#15711,.F.);
#21786=ORIENTED_EDGE('',*,*,#14961,.F.);
#21787=ORIENTED_EDGE('',*,*,#15711,.T.);
#21788=ORIENTED_EDGE('',*,*,#15293,.F.);
#21789=ORIENTED_EDGE('',*,*,#15712,.F.);
#21790=ORIENTED_EDGE('',*,*,#14962,.F.);
#21791=ORIENTED_EDGE('',*,*,#15712,.T.);
#21792=ORIENTED_EDGE('',*,*,#15292,.F.);
#21793=ORIENTED_EDGE('',*,*,#15713,.F.);
#21794=ORIENTED_EDGE('',*,*,#14963,.F.);
#21795=ORIENTED_EDGE('',*,*,#15713,.T.);
#21796=ORIENTED_EDGE('',*,*,#15291,.F.);
#21797=ORIENTED_EDGE('',*,*,#15714,.F.);
#21798=ORIENTED_EDGE('',*,*,#14964,.F.);
#21799=ORIENTED_EDGE('',*,*,#15714,.T.);
#21800=ORIENTED_EDGE('',*,*,#15290,.F.);
#21801=ORIENTED_EDGE('',*,*,#15715,.F.);
#21802=ORIENTED_EDGE('',*,*,#14965,.F.);
#21803=ORIENTED_EDGE('',*,*,#15715,.T.);
#21804=ORIENTED_EDGE('',*,*,#15289,.F.);
#21805=ORIENTED_EDGE('',*,*,#15716,.F.);
#21806=ORIENTED_EDGE('',*,*,#14966,.F.);
#21807=ORIENTED_EDGE('',*,*,#15716,.T.);
#21808=ORIENTED_EDGE('',*,*,#15288,.F.);
#21809=ORIENTED_EDGE('',*,*,#15717,.F.);
#21810=ORIENTED_EDGE('',*,*,#14967,.F.);
#21811=ORIENTED_EDGE('',*,*,#15717,.T.);
#21812=ORIENTED_EDGE('',*,*,#15287,.F.);
#21813=ORIENTED_EDGE('',*,*,#15718,.F.);
#21814=ORIENTED_EDGE('',*,*,#14968,.F.);
#21815=ORIENTED_EDGE('',*,*,#15718,.T.);
#21816=ORIENTED_EDGE('',*,*,#15286,.F.);
#21817=ORIENTED_EDGE('',*,*,#15719,.F.);
#21818=ORIENTED_EDGE('',*,*,#15143,.F.);
#21819=ORIENTED_EDGE('',*,*,#14969,.F.);
#21820=ORIENTED_EDGE('',*,*,#15719,.T.);
#21821=ORIENTED_EDGE('',*,*,#15285,.F.);
#21822=ORIENTED_EDGE('',*,*,#15526,.F.);
#21823=ORIENTED_EDGE('',*,*,#15720,.F.);
#21824=ORIENTED_EDGE('',*,*,#15144,.F.);
#21825=ORIENTED_EDGE('',*,*,#15720,.T.);
#21826=ORIENTED_EDGE('',*,*,#15528,.F.);
#21827=ORIENTED_EDGE('',*,*,#15148,.F.);
#21828=ORIENTED_EDGE('',*,*,#14971,.F.);
#21829=ORIENTED_EDGE('',*,*,#15142,.F.);
#21830=ORIENTED_EDGE('',*,*,#15147,.T.);
#21831=ORIENTED_EDGE('',*,*,#15527,.F.);
#21832=ORIENTED_EDGE('',*,*,#15283,.F.);
#21833=ORIENTED_EDGE('',*,*,#15721,.F.);
#21834=ORIENTED_EDGE('',*,*,#14972,.F.);
#21835=ORIENTED_EDGE('',*,*,#15721,.T.);
#21836=ORIENTED_EDGE('',*,*,#15282,.F.);
#21837=ORIENTED_EDGE('',*,*,#15531,.F.);
#21838=ORIENTED_EDGE('',*,*,#15722,.F.);
#21839=ORIENTED_EDGE('',*,*,#15000,.F.);
#21840=ORIENTED_EDGE('',*,*,#15001,.F.);
#21841=ORIENTED_EDGE('',*,*,#15722,.T.);
#21842=ORIENTED_EDGE('',*,*,#15530,.F.);
#21843=ORIENTED_EDGE('',*,*,#15723,.F.);
#21844=ORIENTED_EDGE('',*,*,#15002,.F.);
#21845=ORIENTED_EDGE('',*,*,#15723,.T.);
#21846=ORIENTED_EDGE('',*,*,#15529,.F.);
#21847=ORIENTED_EDGE('',*,*,#15008,.F.);
#21848=ORIENTED_EDGE('',*,*,#14975,.F.);
#21849=ORIENTED_EDGE('',*,*,#15007,.T.);
#21850=ORIENTED_EDGE('',*,*,#15280,.F.);
#21851=ORIENTED_EDGE('',*,*,#15724,.F.);
#21852=ORIENTED_EDGE('',*,*,#14976,.F.);
#21853=ORIENTED_EDGE('',*,*,#15724,.T.);
#21854=ORIENTED_EDGE('',*,*,#15279,.F.);
#21855=ORIENTED_EDGE('',*,*,#15725,.F.);
#21856=ORIENTED_EDGE('',*,*,#14977,.F.);
#21857=ORIENTED_EDGE('',*,*,#15725,.T.);
#21858=ORIENTED_EDGE('',*,*,#15278,.F.);
#21859=ORIENTED_EDGE('',*,*,#15726,.F.);
#21860=ORIENTED_EDGE('',*,*,#14978,.F.);
#21861=ORIENTED_EDGE('',*,*,#15726,.T.);
#21862=ORIENTED_EDGE('',*,*,#15277,.F.);
#21863=ORIENTED_EDGE('',*,*,#15727,.F.);
#21864=ORIENTED_EDGE('',*,*,#14979,.F.);
#21865=ORIENTED_EDGE('',*,*,#15727,.T.);
#21866=ORIENTED_EDGE('',*,*,#15276,.F.);
#21867=ORIENTED_EDGE('',*,*,#15728,.F.);
#21868=ORIENTED_EDGE('',*,*,#14980,.F.);
#21869=ORIENTED_EDGE('',*,*,#15728,.T.);
#21870=ORIENTED_EDGE('',*,*,#15275,.F.);
#21871=ORIENTED_EDGE('',*,*,#15729,.F.);
#21872=ORIENTED_EDGE('',*,*,#14981,.F.);
#21873=ORIENTED_EDGE('',*,*,#15729,.T.);
#21874=ORIENTED_EDGE('',*,*,#15274,.F.);
#21875=ORIENTED_EDGE('',*,*,#15730,.F.);
#21876=ORIENTED_EDGE('',*,*,#14982,.F.);
#21877=ORIENTED_EDGE('',*,*,#15730,.T.);
#21878=ORIENTED_EDGE('',*,*,#15273,.F.);
#21879=ORIENTED_EDGE('',*,*,#15731,.F.);
#21880=ORIENTED_EDGE('',*,*,#14983,.F.);
#21881=ORIENTED_EDGE('',*,*,#15731,.T.);
#21882=ORIENTED_EDGE('',*,*,#15272,.F.);
#21883=ORIENTED_EDGE('',*,*,#15732,.F.);
#21884=ORIENTED_EDGE('',*,*,#14984,.F.);
#21885=ORIENTED_EDGE('',*,*,#15732,.T.);
#21886=ORIENTED_EDGE('',*,*,#15271,.F.);
#21887=ORIENTED_EDGE('',*,*,#15733,.F.);
#21888=ORIENTED_EDGE('',*,*,#14985,.F.);
#21889=ORIENTED_EDGE('',*,*,#15733,.T.);
#21890=ORIENTED_EDGE('',*,*,#15270,.F.);
#21891=ORIENTED_EDGE('',*,*,#15734,.F.);
#21892=ORIENTED_EDGE('',*,*,#14986,.F.);
#21893=ORIENTED_EDGE('',*,*,#15734,.T.);
#21894=ORIENTED_EDGE('',*,*,#15269,.F.);
#21895=ORIENTED_EDGE('',*,*,#15735,.F.);
#21896=ORIENTED_EDGE('',*,*,#14987,.F.);
#21897=ORIENTED_EDGE('',*,*,#15735,.T.);
#21898=ORIENTED_EDGE('',*,*,#15268,.F.);
#21899=ORIENTED_EDGE('',*,*,#15736,.F.);
#21900=ORIENTED_EDGE('',*,*,#14988,.F.);
#21901=ORIENTED_EDGE('',*,*,#15736,.T.);
#21902=ORIENTED_EDGE('',*,*,#15267,.F.);
#21903=ORIENTED_EDGE('',*,*,#15737,.F.);
#21904=ORIENTED_EDGE('',*,*,#15133,.F.);
#21905=ORIENTED_EDGE('',*,*,#14989,.F.);
#21906=ORIENTED_EDGE('',*,*,#15737,.T.);
#21907=ORIENTED_EDGE('',*,*,#15266,.F.);
#21908=ORIENTED_EDGE('',*,*,#15532,.F.);
#21909=ORIENTED_EDGE('',*,*,#15738,.F.);
#21910=ORIENTED_EDGE('',*,*,#15134,.F.);
#21911=ORIENTED_EDGE('',*,*,#15738,.T.);
#21912=ORIENTED_EDGE('',*,*,#15534,.F.);
#21913=ORIENTED_EDGE('',*,*,#15138,.F.);
#21914=ORIENTED_EDGE('',*,*,#14991,.F.);
#21915=ORIENTED_EDGE('',*,*,#15132,.F.);
#21916=ORIENTED_EDGE('',*,*,#15137,.T.);
#21917=ORIENTED_EDGE('',*,*,#15533,.F.);
#21918=ORIENTED_EDGE('',*,*,#15264,.F.);
#21919=ORIENTED_EDGE('',*,*,#15739,.F.);
#21920=ORIENTED_EDGE('',*,*,#14753,.F.);
#21921=ORIENTED_EDGE('',*,*,#15739,.T.);
#21922=ORIENTED_EDGE('',*,*,#15263,.F.);
#21923=ORIENTED_EDGE('',*,*,#15537,.F.);
#21924=ORIENTED_EDGE('',*,*,#15740,.F.);
#21925=ORIENTED_EDGE('',*,*,#14749,.F.);
#21926=ORIENTED_EDGE('',*,*,#14750,.F.);
#21927=ORIENTED_EDGE('',*,*,#15740,.T.);
#21928=ORIENTED_EDGE('',*,*,#15536,.F.);
#21929=ORIENTED_EDGE('',*,*,#15741,.F.);
#21930=ORIENTED_EDGE('',*,*,#14751,.F.);
#21931=ORIENTED_EDGE('',*,*,#15741,.T.);
#21932=ORIENTED_EDGE('',*,*,#15535,.F.);
#21933=ORIENTED_EDGE('',*,*,#14997,.F.);
#21934=ORIENTED_EDGE('',*,*,#14755,.F.);
#21935=ORIENTED_EDGE('',*,*,#14996,.T.);
#21936=ORIENTED_EDGE('',*,*,#15261,.F.);
#21937=ORIENTED_EDGE('',*,*,#15742,.F.);
#21938=ORIENTED_EDGE('',*,*,#14756,.F.);
#21939=ORIENTED_EDGE('',*,*,#15742,.T.);
#21940=ORIENTED_EDGE('',*,*,#15260,.F.);
#21941=ORIENTED_EDGE('',*,*,#15743,.F.);
#21942=ORIENTED_EDGE('',*,*,#14757,.F.);
#21943=ORIENTED_EDGE('',*,*,#15743,.T.);
#21944=ORIENTED_EDGE('',*,*,#15259,.F.);
#21945=ORIENTED_EDGE('',*,*,#15744,.F.);
#21946=ORIENTED_EDGE('',*,*,#14758,.F.);
#21947=ORIENTED_EDGE('',*,*,#15744,.T.);
#21948=ORIENTED_EDGE('',*,*,#15258,.F.);
#21949=ORIENTED_EDGE('',*,*,#15745,.F.);
#21950=ORIENTED_EDGE('',*,*,#14759,.F.);
#21951=ORIENTED_EDGE('',*,*,#15745,.T.);
#21952=ORIENTED_EDGE('',*,*,#15257,.F.);
#21953=ORIENTED_EDGE('',*,*,#15746,.F.);
#21954=ORIENTED_EDGE('',*,*,#14760,.F.);
#21955=ORIENTED_EDGE('',*,*,#15746,.T.);
#21956=ORIENTED_EDGE('',*,*,#15256,.F.);
#21957=ORIENTED_EDGE('',*,*,#15747,.F.);
#21958=ORIENTED_EDGE('',*,*,#14761,.F.);
#21959=ORIENTED_EDGE('',*,*,#15747,.T.);
#21960=ORIENTED_EDGE('',*,*,#15255,.F.);
#21961=ORIENTED_EDGE('',*,*,#15748,.F.);
#21962=ORIENTED_EDGE('',*,*,#14762,.F.);
#21963=ORIENTED_EDGE('',*,*,#15748,.T.);
#21964=ORIENTED_EDGE('',*,*,#15254,.F.);
#21965=ORIENTED_EDGE('',*,*,#15749,.F.);
#21966=ORIENTED_EDGE('',*,*,#14763,.F.);
#21967=ORIENTED_EDGE('',*,*,#15749,.T.);
#21968=ORIENTED_EDGE('',*,*,#15253,.F.);
#21969=ORIENTED_EDGE('',*,*,#15750,.F.);
#21970=ORIENTED_EDGE('',*,*,#14764,.F.);
#21971=ORIENTED_EDGE('',*,*,#15750,.T.);
#21972=ORIENTED_EDGE('',*,*,#15252,.F.);
#21973=ORIENTED_EDGE('',*,*,#15751,.F.);
#21974=ORIENTED_EDGE('',*,*,#14765,.F.);
#21975=ORIENTED_EDGE('',*,*,#15751,.T.);
#21976=ORIENTED_EDGE('',*,*,#15251,.F.);
#21977=ORIENTED_EDGE('',*,*,#15752,.F.);
#21978=ORIENTED_EDGE('',*,*,#14766,.F.);
#21979=ORIENTED_EDGE('',*,*,#15752,.T.);
#21980=ORIENTED_EDGE('',*,*,#15250,.F.);
#21981=ORIENTED_EDGE('',*,*,#15753,.F.);
#21982=ORIENTED_EDGE('',*,*,#14767,.F.);
#21983=ORIENTED_EDGE('',*,*,#15753,.T.);
#21984=ORIENTED_EDGE('',*,*,#15249,.F.);
#21985=ORIENTED_EDGE('',*,*,#15754,.F.);
#21986=ORIENTED_EDGE('',*,*,#14768,.F.);
#21987=ORIENTED_EDGE('',*,*,#15754,.T.);
#21988=ORIENTED_EDGE('',*,*,#15248,.F.);
#21989=ORIENTED_EDGE('',*,*,#15755,.F.);
#21990=ORIENTED_EDGE('',*,*,#15123,.F.);
#21991=ORIENTED_EDGE('',*,*,#14769,.F.);
#21992=ORIENTED_EDGE('',*,*,#15755,.T.);
#21993=ORIENTED_EDGE('',*,*,#15247,.F.);
#21994=ORIENTED_EDGE('',*,*,#15538,.F.);
#21995=ORIENTED_EDGE('',*,*,#15756,.F.);
#21996=ORIENTED_EDGE('',*,*,#15124,.F.);
#21997=ORIENTED_EDGE('',*,*,#15756,.T.);
#21998=ORIENTED_EDGE('',*,*,#15540,.F.);
#21999=ORIENTED_EDGE('',*,*,#15128,.F.);
#22000=ORIENTED_EDGE('',*,*,#14771,.F.);
#22001=ORIENTED_EDGE('',*,*,#15122,.F.);
#22002=ORIENTED_EDGE('',*,*,#15127,.T.);
#22003=ORIENTED_EDGE('',*,*,#15539,.F.);
#22004=ORIENTED_EDGE('',*,*,#15245,.F.);
#22005=ORIENTED_EDGE('',*,*,#15541,.F.);
#22006=ORIENTED_EDGE('',*,*,#14992,.T.);
#22007=ORIENTED_EDGE('',*,*,#15757,.T.);
#22008=ORIENTED_EDGE('',*,*,#15758,.T.);
#22009=ORIENTED_EDGE('',*,*,#15757,.F.);
#22010=ORIENTED_EDGE('',*,*,#15758,.F.);
#22011=ORIENTED_EDGE('',*,*,#15759,.F.);
#22012=ORIENTED_EDGE('',*,*,#15760,.T.);
#22013=ORIENTED_EDGE('',*,*,#15471,.T.);
#22014=ORIENTED_EDGE('',*,*,#15760,.F.);
#22015=ORIENTED_EDGE('',*,*,#15759,.T.);
#24261=ADVANCED_FACE('',(#2402),#1160,.T.);
#24262=ADVANCED_FACE('',(#2403,#649),#1161,.F.);
#24263=ADVANCED_FACE('',(#2404),#1162,.T.);
#24264=ADVANCED_FACE('',(#2405),#1163,.T.);
#24265=ADVANCED_FACE('',(#2406),#1164,.T.);
#24266=ADVANCED_FACE('',(#2407),#1165,.T.);
#24267=ADVANCED_FACE('',(#2408),#1166,.T.);
#24268=ADVANCED_FACE('',(#2409),#1167,.T.);
#24269=ADVANCED_FACE('',(#2410),#1168,.T.);
#24270=ADVANCED_FACE('',(#2411),#1169,.T.);
#24271=ADVANCED_FACE('',(#2412),#1170,.T.);
#24272=ADVANCED_FACE('',(#2413),#1171,.T.);
#24273=ADVANCED_FACE('',(#2414),#1172,.T.);
#24274=ADVANCED_FACE('',(#2415),#1173,.T.);
#24275=ADVANCED_FACE('',(#2416),#1174,.T.);
#24276=ADVANCED_FACE('',(#2417),#1175,.T.);
#24277=ADVANCED_FACE('',(#2418),#1176,.T.);
#24278=ADVANCED_FACE('',(#2419),#1177,.T.);
#24279=ADVANCED_FACE('',(#2420),#1178,.T.);
#24280=ADVANCED_FACE('',(#2421),#1179,.T.);
#24281=ADVANCED_FACE('',(#2422),#1180,.T.);
#24282=ADVANCED_FACE('',(#2423),#1181,.T.);
#24283=ADVANCED_FACE('',(#2424),#1182,.T.);
#24284=ADVANCED_FACE('',(#2425),#1183,.T.);
#24285=ADVANCED_FACE('',(#2426),#1184,.T.);
#24286=ADVANCED_FACE('',(#2427),#1185,.T.);
#24287=ADVANCED_FACE('',(#2428),#1186,.T.);
#24288=ADVANCED_FACE('',(#2429),#1187,.T.);
#24289=ADVANCED_FACE('',(#2430),#1188,.T.);
#24290=ADVANCED_FACE('',(#2431),#1189,.T.);
#24291=ADVANCED_FACE('',(#2432),#1190,.T.);
#24292=ADVANCED_FACE('',(#2433),#1191,.T.);
#24293=ADVANCED_FACE('',(#2434),#1192,.T.);
#24294=ADVANCED_FACE('',(#2435),#1193,.T.);
#24295=ADVANCED_FACE('',(#2436),#1194,.T.);
#24296=ADVANCED_FACE('',(#2437),#1195,.T.);
#24297=ADVANCED_FACE('',(#2438),#1196,.T.);
#24298=ADVANCED_FACE('',(#2439),#1197,.T.);
#24299=ADVANCED_FACE('',(#2440),#1198,.T.);
#24300=ADVANCED_FACE('',(#2441),#1199,.T.);
#24301=ADVANCED_FACE('',(#2442),#1200,.T.);
#24302=ADVANCED_FACE('',(#2443),#1201,.T.);
#24303=ADVANCED_FACE('',(#2444),#1202,.T.);
#24304=ADVANCED_FACE('',(#2445),#1203,.T.);
#24305=ADVANCED_FACE('',(#2446),#1204,.T.);
#24306=ADVANCED_FACE('',(#2447),#1205,.T.);
#24307=ADVANCED_FACE('',(#2448),#1206,.T.);
#24308=ADVANCED_FACE('',(#2449),#1207,.T.);
#24309=ADVANCED_FACE('',(#2450),#1208,.T.);
#24310=ADVANCED_FACE('',(#2451),#1209,.T.);
#24311=ADVANCED_FACE('',(#2452),#1210,.T.);
#24312=ADVANCED_FACE('',(#2453),#1211,.T.);
#24313=ADVANCED_FACE('',(#2454),#1212,.T.);
#24314=ADVANCED_FACE('',(#2455),#1213,.T.);
#24315=ADVANCED_FACE('',(#2456),#1214,.T.);
#24316=ADVANCED_FACE('',(#2457),#1215,.T.);
#24317=ADVANCED_FACE('',(#2458),#1216,.T.);
#24318=ADVANCED_FACE('',(#2459),#1217,.T.);
#24319=ADVANCED_FACE('',(#2460),#1218,.T.);
#24320=ADVANCED_FACE('',(#2461),#1219,.T.);
#24321=ADVANCED_FACE('',(#2462),#1220,.T.);
#24322=ADVANCED_FACE('',(#2463),#1221,.T.);
#24323=ADVANCED_FACE('',(#2464),#1222,.T.);
#24324=ADVANCED_FACE('',(#2465),#1223,.T.);
#24325=ADVANCED_FACE('',(#2466),#1224,.T.);
#24326=ADVANCED_FACE('',(#2467),#1225,.T.);
#24327=ADVANCED_FACE('',(#2468),#1226,.T.);
#24328=ADVANCED_FACE('',(#2469),#1227,.T.);
#24329=ADVANCED_FACE('',(#2470),#1228,.T.);
#24330=ADVANCED_FACE('',(#2471),#1229,.T.);
#24331=ADVANCED_FACE('',(#2472),#1230,.T.);
#24332=ADVANCED_FACE('',(#2473),#1231,.T.);
#24333=ADVANCED_FACE('',(#2474),#1232,.T.);
#24334=ADVANCED_FACE('',(#2475),#1233,.T.);
#24335=ADVANCED_FACE('',(#2476,#650),#1234,.T.);
#24336=ADVANCED_FACE('',(#2477),#1235,.T.);
#24337=ADVANCED_FACE('',(#2478),#1236,.T.);
#24338=ADVANCED_FACE('',(#2479),#1237,.T.);
#24339=ADVANCED_FACE('',(#2480),#1238,.T.);
#24340=ADVANCED_FACE('',(#2481),#1239,.T.);
#24341=ADVANCED_FACE('',(#2482),#1240,.T.);
#24342=ADVANCED_FACE('',(#2483),#1241,.T.);
#24343=ADVANCED_FACE('',(#2484),#1242,.T.);
#24344=ADVANCED_FACE('',(#2485),#1243,.T.);
#24345=ADVANCED_FACE('',(#2486),#1244,.T.);
#24346=ADVANCED_FACE('',(#2487),#1245,.T.);
#24347=ADVANCED_FACE('',(#2488),#1246,.T.);
#24348=ADVANCED_FACE('',(#2489),#1247,.T.);
#24349=ADVANCED_FACE('',(#2490),#1248,.T.);
#24350=ADVANCED_FACE('',(#2491),#1249,.T.);
#24351=ADVANCED_FACE('',(#2492),#1250,.T.);
#24352=ADVANCED_FACE('',(#2493),#1251,.T.);
#24353=ADVANCED_FACE('',(#2494),#1252,.T.);
#24354=ADVANCED_FACE('',(#2495),#1253,.T.);
#24355=ADVANCED_FACE('',(#2496),#1254,.T.);
#24356=ADVANCED_FACE('',(#2497),#1255,.T.);
#24357=ADVANCED_FACE('',(#2498),#1256,.T.);
#24358=ADVANCED_FACE('',(#2499),#1257,.T.);
#24359=ADVANCED_FACE('',(#2500),#1258,.T.);
#24360=ADVANCED_FACE('',(#2501),#1259,.T.);
#24361=ADVANCED_FACE('',(#2502),#1260,.T.);
#24362=ADVANCED_FACE('',(#2503),#1261,.T.);
#24363=ADVANCED_FACE('',(#2504),#1262,.T.);
#24364=ADVANCED_FACE('',(#2505),#1263,.T.);
#24365=ADVANCED_FACE('',(#2506),#1264,.T.);
#24366=ADVANCED_FACE('',(#2507),#1265,.T.);
#24367=ADVANCED_FACE('',(#2508),#1266,.T.);
#24368=ADVANCED_FACE('',(#2509),#1267,.T.);
#24369=ADVANCED_FACE('',(#2510),#1268,.T.);
#24370=ADVANCED_FACE('',(#2511),#1269,.T.);
#24371=ADVANCED_FACE('',(#2512),#1270,.T.);
#24372=ADVANCED_FACE('',(#2513),#1271,.T.);
#24373=ADVANCED_FACE('',(#2514),#1272,.T.);
#24374=ADVANCED_FACE('',(#2515),#1273,.T.);
#24375=ADVANCED_FACE('',(#2516),#1274,.T.);
#24376=ADVANCED_FACE('',(#2517),#1275,.T.);
#24377=ADVANCED_FACE('',(#2518),#1276,.T.);
#24378=ADVANCED_FACE('',(#2519),#1277,.T.);
#24379=ADVANCED_FACE('',(#2520),#1278,.T.);
#24380=ADVANCED_FACE('',(#2521),#1279,.T.);
#24381=ADVANCED_FACE('',(#2522),#1280,.T.);
#24382=ADVANCED_FACE('',(#2523),#1281,.T.);
#24383=ADVANCED_FACE('',(#2524),#1282,.T.);
#24384=ADVANCED_FACE('',(#2525),#1283,.T.);
#24385=ADVANCED_FACE('',(#2526),#1284,.T.);
#24386=ADVANCED_FACE('',(#2527),#1285,.T.);
#24387=ADVANCED_FACE('',(#2528),#1286,.T.);
#24388=ADVANCED_FACE('',(#2529),#1287,.T.);
#24389=ADVANCED_FACE('',(#2530),#1288,.T.);
#24390=ADVANCED_FACE('',(#2531),#1289,.T.);
#24391=ADVANCED_FACE('',(#2532),#1290,.T.);
#24392=ADVANCED_FACE('',(#2533),#1291,.T.);
#24393=ADVANCED_FACE('',(#2534),#1292,.T.);
#24394=ADVANCED_FACE('',(#2535),#1293,.T.);
#24395=ADVANCED_FACE('',(#2536),#1294,.T.);
#24396=ADVANCED_FACE('',(#2537),#1295,.T.);
#24397=ADVANCED_FACE('',(#2538),#1296,.T.);
#24398=ADVANCED_FACE('',(#2539),#1297,.T.);
#24399=ADVANCED_FACE('',(#2540),#1298,.T.);
#24400=ADVANCED_FACE('',(#2541),#1299,.T.);
#24401=ADVANCED_FACE('',(#2542),#1300,.T.);
#24402=ADVANCED_FACE('',(#2543),#1301,.T.);
#24403=ADVANCED_FACE('',(#2544),#1302,.T.);
#24404=ADVANCED_FACE('',(#2545),#1303,.T.);
#24405=ADVANCED_FACE('',(#2546),#1304,.T.);
#24406=ADVANCED_FACE('',(#2547),#1305,.T.);
#24407=ADVANCED_FACE('',(#2548),#1306,.T.);
#24408=ADVANCED_FACE('',(#2549),#1307,.T.);
#24409=ADVANCED_FACE('',(#2550),#1308,.T.);
#24410=ADVANCED_FACE('',(#2551),#1309,.T.);
#24411=ADVANCED_FACE('',(#2552),#1310,.T.);
#24412=ADVANCED_FACE('',(#2553),#1311,.T.);
#24413=ADVANCED_FACE('',(#2554),#1312,.T.);
#24414=ADVANCED_FACE('',(#2555),#1313,.T.);
#24415=ADVANCED_FACE('',(#2556),#1314,.T.);
#24416=ADVANCED_FACE('',(#2557),#1315,.T.);
#24417=ADVANCED_FACE('',(#2558),#1316,.T.);
#24418=ADVANCED_FACE('',(#2559),#1317,.T.);
#24419=ADVANCED_FACE('',(#2560),#1318,.T.);
#24420=ADVANCED_FACE('',(#2561),#1319,.T.);
#24421=ADVANCED_FACE('',(#2562),#1320,.T.);
#24422=ADVANCED_FACE('',(#2563),#1321,.T.);
#24423=ADVANCED_FACE('',(#2564),#1322,.T.);
#24424=ADVANCED_FACE('',(#2565),#1323,.T.);
#24425=ADVANCED_FACE('',(#2566),#1324,.T.);
#24426=ADVANCED_FACE('',(#2567),#1325,.T.);
#24427=ADVANCED_FACE('',(#2568),#1326,.T.);
#24428=ADVANCED_FACE('',(#2569),#1327,.T.);
#24429=ADVANCED_FACE('',(#2570),#1328,.T.);
#24430=ADVANCED_FACE('',(#2571),#1329,.T.);
#24431=ADVANCED_FACE('',(#2572),#1330,.T.);
#24432=ADVANCED_FACE('',(#2573),#1331,.T.);
#24433=ADVANCED_FACE('',(#2574),#1332,.T.);
#24434=ADVANCED_FACE('',(#2575),#1333,.T.);
#24435=ADVANCED_FACE('',(#2576),#1334,.T.);
#24436=ADVANCED_FACE('',(#2577),#1335,.T.);
#24437=ADVANCED_FACE('',(#2578),#1336,.T.);
#24438=ADVANCED_FACE('',(#2579),#1337,.T.);
#24439=ADVANCED_FACE('',(#2580),#1338,.T.);
#24440=ADVANCED_FACE('',(#2581),#1339,.T.);
#24441=ADVANCED_FACE('',(#2582),#1340,.T.);
#24442=ADVANCED_FACE('',(#2583),#1341,.T.);
#24443=ADVANCED_FACE('',(#2584),#1342,.T.);
#24444=ADVANCED_FACE('',(#2585),#1343,.T.);
#24445=ADVANCED_FACE('',(#2586),#1344,.T.);
#24446=ADVANCED_FACE('',(#2587),#1345,.T.);
#24447=ADVANCED_FACE('',(#2588),#1346,.T.);
#24448=ADVANCED_FACE('',(#2589),#1347,.T.);
#24449=ADVANCED_FACE('',(#2590),#1348,.T.);
#24450=ADVANCED_FACE('',(#2591),#1349,.T.);
#24451=ADVANCED_FACE('',(#2592),#1350,.T.);
#24452=ADVANCED_FACE('',(#2593),#1351,.T.);
#24453=ADVANCED_FACE('',(#2594),#1352,.T.);
#24454=ADVANCED_FACE('',(#2595),#1353,.T.);
#24455=ADVANCED_FACE('',(#2596),#1354,.T.);
#24456=ADVANCED_FACE('',(#2597),#1355,.T.);
#24457=ADVANCED_FACE('',(#2598),#1356,.T.);
#24458=ADVANCED_FACE('',(#2599),#1357,.T.);
#24459=ADVANCED_FACE('',(#2600),#1358,.T.);
#24460=ADVANCED_FACE('',(#2601),#1359,.T.);
#24461=ADVANCED_FACE('',(#2602),#1360,.T.);
#24462=ADVANCED_FACE('',(#2603),#1361,.T.);
#24463=ADVANCED_FACE('',(#2604),#1362,.T.);
#24464=ADVANCED_FACE('',(#2605),#1363,.T.);
#24465=ADVANCED_FACE('',(#2606),#1364,.T.);
#24466=ADVANCED_FACE('',(#2607),#1365,.T.);
#24467=ADVANCED_FACE('',(#2608),#1366,.T.);
#24468=ADVANCED_FACE('',(#2609),#1367,.T.);
#24469=ADVANCED_FACE('',(#2610),#1368,.T.);
#24470=ADVANCED_FACE('',(#2611),#1369,.T.);
#24471=ADVANCED_FACE('',(#2612),#1370,.T.);
#24472=ADVANCED_FACE('',(#2613),#1371,.T.);
#24473=ADVANCED_FACE('',(#2614),#1372,.T.);
#24474=ADVANCED_FACE('',(#2615),#1373,.T.);
#24475=ADVANCED_FACE('',(#2616),#1374,.T.);
#24476=ADVANCED_FACE('',(#2617),#1375,.T.);
#24477=ADVANCED_FACE('',(#2618),#1376,.T.);
#24478=ADVANCED_FACE('',(#2619),#1377,.T.);
#24479=ADVANCED_FACE('',(#2620),#1378,.T.);
#24480=ADVANCED_FACE('',(#2621),#1379,.T.);
#24481=ADVANCED_FACE('',(#2622),#1380,.T.);
#24482=ADVANCED_FACE('',(#2623),#1381,.T.);
#24483=ADVANCED_FACE('',(#2624),#1382,.T.);
#24484=ADVANCED_FACE('',(#2625),#1383,.T.);
#24485=ADVANCED_FACE('',(#2626),#1384,.T.);
#24486=ADVANCED_FACE('',(#2627),#1385,.T.);
#24487=ADVANCED_FACE('',(#2628),#1386,.T.);
#24488=ADVANCED_FACE('',(#2629),#1387,.T.);
#24489=ADVANCED_FACE('',(#2630),#1388,.T.);
#24490=ADVANCED_FACE('',(#2631),#1389,.T.);
#24491=ADVANCED_FACE('',(#2632),#1390,.T.);
#24492=ADVANCED_FACE('',(#2633),#1391,.T.);
#24493=ADVANCED_FACE('',(#2634),#1392,.T.);
#24494=ADVANCED_FACE('',(#2635),#1393,.T.);
#24495=ADVANCED_FACE('',(#2636),#1394,.T.);
#24496=ADVANCED_FACE('',(#2637),#1395,.T.);
#24497=ADVANCED_FACE('',(#2638),#1396,.T.);
#24498=ADVANCED_FACE('',(#2639),#1397,.T.);
#24499=ADVANCED_FACE('',(#2640),#1398,.T.);
#24500=ADVANCED_FACE('',(#2641),#1399,.T.);
#24501=ADVANCED_FACE('',(#2642),#1400,.T.);
#24502=ADVANCED_FACE('',(#2643),#1401,.T.);
#24503=ADVANCED_FACE('',(#2644),#1402,.T.);
#24504=ADVANCED_FACE('',(#2645),#1403,.T.);
#24505=ADVANCED_FACE('',(#2646),#1404,.T.);
#24506=ADVANCED_FACE('',(#2647),#1405,.T.);
#24507=ADVANCED_FACE('',(#2648),#1406,.T.);
#24508=ADVANCED_FACE('',(#2649),#1407,.T.);
#24509=ADVANCED_FACE('',(#2650),#1408,.T.);
#24510=ADVANCED_FACE('',(#2651),#1409,.T.);
#24511=ADVANCED_FACE('',(#2652),#1410,.T.);
#24512=ADVANCED_FACE('',(#2653),#1411,.T.);
#24513=ADVANCED_FACE('',(#2654),#1412,.T.);
#24514=ADVANCED_FACE('',(#2655),#1413,.T.);
#24515=ADVANCED_FACE('',(#2656),#1414,.T.);
#24516=ADVANCED_FACE('',(#2657),#1415,.T.);
#24517=ADVANCED_FACE('',(#2658),#1416,.T.);
#24518=ADVANCED_FACE('',(#2659),#1417,.T.);
#24519=ADVANCED_FACE('',(#2660),#1418,.T.);
#24520=ADVANCED_FACE('',(#2661),#1419,.T.);
#24521=ADVANCED_FACE('',(#2662),#1420,.T.);
#24522=ADVANCED_FACE('',(#2663),#1421,.T.);
#24523=ADVANCED_FACE('',(#2664),#1422,.T.);
#24524=ADVANCED_FACE('',(#2665),#1423,.T.);
#24525=ADVANCED_FACE('',(#2666),#1424,.T.);
#24526=ADVANCED_FACE('',(#2667),#1425,.T.);
#24527=ADVANCED_FACE('',(#2668),#1426,.T.);
#24528=ADVANCED_FACE('',(#2669),#1427,.T.);
#24529=ADVANCED_FACE('',(#2670),#1428,.T.);
#24530=ADVANCED_FACE('',(#2671),#1429,.T.);
#24531=ADVANCED_FACE('',(#2672),#1430,.T.);
#24532=ADVANCED_FACE('',(#2673),#1431,.T.);
#24533=ADVANCED_FACE('',(#2674),#1432,.T.);
#24534=ADVANCED_FACE('',(#2675),#1433,.T.);
#24535=ADVANCED_FACE('',(#2676),#1434,.T.);
#24536=ADVANCED_FACE('',(#2677),#1435,.T.);
#24537=ADVANCED_FACE('',(#2678),#1436,.T.);
#24538=ADVANCED_FACE('',(#2679),#1437,.T.);
#24539=ADVANCED_FACE('',(#2680),#1438,.T.);
#24540=ADVANCED_FACE('',(#2681),#1439,.T.);
#24541=ADVANCED_FACE('',(#2682),#1440,.T.);
#24542=ADVANCED_FACE('',(#2683),#1441,.T.);
#24543=ADVANCED_FACE('',(#2684),#1442,.T.);
#24544=ADVANCED_FACE('',(#2685),#1443,.T.);
#24545=ADVANCED_FACE('',(#2686),#1444,.T.);
#24546=ADVANCED_FACE('',(#2687),#1445,.T.);
#24547=ADVANCED_FACE('',(#2688),#1446,.T.);
#24548=ADVANCED_FACE('',(#2689),#1447,.T.);
#24549=ADVANCED_FACE('',(#2690),#1448,.T.);
#24550=ADVANCED_FACE('',(#2691),#1449,.T.);
#24551=ADVANCED_FACE('',(#2692),#1450,.T.);
#24552=ADVANCED_FACE('',(#2693),#1451,.T.);
#24553=ADVANCED_FACE('',(#2694),#1452,.T.);
#24554=ADVANCED_FACE('',(#2695),#1453,.T.);
#24555=ADVANCED_FACE('',(#2696),#1454,.T.);
#24556=ADVANCED_FACE('',(#2697),#1455,.T.);
#24557=ADVANCED_FACE('',(#2698),#1456,.T.);
#24558=ADVANCED_FACE('',(#2699),#1457,.T.);
#24559=ADVANCED_FACE('',(#2700),#1458,.T.);
#24560=ADVANCED_FACE('',(#2701),#1459,.T.);
#24561=ADVANCED_FACE('',(#2702),#1460,.T.);
#24562=ADVANCED_FACE('',(#2703),#1461,.T.);
#24563=ADVANCED_FACE('',(#2704),#1462,.T.);
#24564=ADVANCED_FACE('',(#2705),#1463,.T.);
#24565=ADVANCED_FACE('',(#2706),#1464,.T.);
#24566=ADVANCED_FACE('',(#2707),#1465,.T.);
#24567=ADVANCED_FACE('',(#2708),#1466,.T.);
#24568=ADVANCED_FACE('',(#2709),#1467,.T.);
#24569=ADVANCED_FACE('',(#2710),#1468,.T.);
#24570=ADVANCED_FACE('',(#2711),#1469,.T.);
#24571=ADVANCED_FACE('',(#2712),#1470,.T.);
#24572=ADVANCED_FACE('',(#2713),#1471,.T.);
#24573=ADVANCED_FACE('',(#2714),#1472,.T.);
#24574=ADVANCED_FACE('',(#2715),#1473,.T.);
#24575=ADVANCED_FACE('',(#2716),#1474,.T.);
#24576=ADVANCED_FACE('',(#2717),#1475,.T.);
#24577=ADVANCED_FACE('',(#2718),#1476,.T.);
#24578=ADVANCED_FACE('',(#2719),#1477,.T.);
#24579=ADVANCED_FACE('',(#2720),#1478,.T.);
#24580=ADVANCED_FACE('',(#2721),#1479,.T.);
#24581=ADVANCED_FACE('',(#2722),#1480,.T.);
#24582=ADVANCED_FACE('',(#2723),#1481,.T.);
#24583=ADVANCED_FACE('',(#2724),#1482,.T.);
#24584=ADVANCED_FACE('',(#2725),#1483,.T.);
#24585=ADVANCED_FACE('',(#2726),#1484,.T.);
#24586=ADVANCED_FACE('',(#2727),#1485,.T.);
#24587=ADVANCED_FACE('',(#2728),#1486,.T.);
#24588=ADVANCED_FACE('',(#2729),#1487,.T.);
#24589=ADVANCED_FACE('',(#2730),#1488,.T.);
#24590=ADVANCED_FACE('',(#2731),#1489,.T.);
#24591=ADVANCED_FACE('',(#2732),#1490,.T.);
#24592=ADVANCED_FACE('',(#2733),#1491,.T.);
#24593=ADVANCED_FACE('',(#2734),#1492,.T.);
#24594=ADVANCED_FACE('',(#2735),#1493,.T.);
#24595=ADVANCED_FACE('',(#2736),#1494,.T.);
#24596=ADVANCED_FACE('',(#2737),#1495,.T.);
#24597=ADVANCED_FACE('',(#2738),#1496,.T.);
#24598=ADVANCED_FACE('',(#2739),#1497,.T.);
#24599=ADVANCED_FACE('',(#2740),#517,.T.);
#24600=ADVANCED_FACE('',(#2741),#1498,.T.);
#24601=ADVANCED_FACE('',(#2742),#518,.T.);
#24602=ADVANCED_FACE('',(#2743),#1499,.T.);
#24941=CLOSED_SHELL('',(#24261,#24262,#24263,#24264,#24265,#24266,#24267,
#24268,#24269,#24270,#24271,#24272,#24273,#24274,#24275,#24276,#24277,#24278,
#24279,#24280,#24281,#24282,#24283,#24284,#24285,#24286,#24287,#24288,#24289,
#24290,#24291,#24292,#24293,#24294,#24295,#24296,#24297,#24298,#24299,#24300,
#24301,#24302,#24303,#24304,#24305,#24306,#24307,#24308,#24309,#24310,#24311,
#24312,#24313,#24314,#24315,#24316,#24317,#24318,#24319,#24320,#24321,#24322,
#24323,#24324,#24325,#24326,#24327,#24328,#24329,#24330,#24331,#24332,#24333,
#24334,#24335,#24336,#24337,#24338,#24339,#24340,#24341,#24342,#24343,#24344,
#24345,#24346,#24347,#24348,#24349,#24350,#24351,#24352,#24353,#24354,#24355,
#24356,#24357,#24358,#24359,#24360,#24361,#24362,#24363,#24364,#24365,#24366,
#24367,#24368,#24369,#24370,#24371,#24372,#24373,#24374,#24375,#24376,#24377,
#24378,#24379,#24380,#24381,#24382,#24383,#24384,#24385,#24386,#24387,#24388,
#24389,#24390,#24391,#24392,#24393,#24394,#24395,#24396,#24397,#24398,#24399,
#24400,#24401,#24402,#24403,#24404,#24405,#24406,#24407,#24408,#24409,#24410,
#24411,#24412,#24413,#24414,#24415,#24416,#24417,#24418,#24419,#24420,#24421,
#24422,#24423,#24424,#24425,#24426,#24427,#24428,#24429,#24430,#24431,#24432,
#24433,#24434,#24435,#24436,#24437,#24438,#24439,#24440,#24441,#24442,#24443,
#24444,#24445,#24446,#24447,#24448,#24449,#24450,#24451,#24452,#24453,#24454,
#24455,#24456,#24457,#24458,#24459,#24460,#24461,#24462,#24463,#24464,#24465,
#24466,#24467,#24468,#24469,#24470,#24471,#24472,#24473,#24474,#24475,#24476,
#24477,#24478,#24479,#24480,#24481,#24482,#24483,#24484,#24485,#24486,#24487,
#24488,#24489,#24490,#24491,#24492,#24493,#24494,#24495,#24496,#24497,#24498,
#24499,#24500,#24501,#24502,#24503,#24504,#24505,#24506,#24507,#24508,#24509,
#24510,#24511,#24512,#24513,#24514,#24515,#24516,#24517,#24518,#24519,#24520,
#24521,#24522,#24523,#24524,#24525,#24526,#24527,#24528,#24529,#24530,#24531,
#24532,#24533,#24534,#24535,#24536,#24537,#24538,#24539,#24540,#24541,#24542,
#24543,#24544,#24545,#24546,#24547,#24548,#24549,#24550,#24551,#24552,#24553,
#24554,#24555,#24556,#24557,#24558,#24559,#24560,#24561,#24562,#24563,#24564,
#24565,#24566,#24567,#24568,#24569,#24570,#24571,#24572,#24573,#24574,#24575,
#24576,#24577,#24578,#24579,#24580,#24581,#24582,#24583,#24584,#24585,#24586,
#24587,#24588,#24589,#24590,#24591,#24592,#24593,#24594,#24595,#24596,#24597,
#24598,#24599,#24600,#24601,#24602));
#26063=AXIS2_PLACEMENT_3D('',#38096,#30202,#30203);
#26064=AXIS2_PLACEMENT_3D('',#38097,#30204,#30205);
#26065=AXIS2_PLACEMENT_3D('',#38110,#30212,#30213);
#26066=AXIS2_PLACEMENT_3D('',#38589,#30453,#30454);
#26067=AXIS2_PLACEMENT_3D('',#38590,#30455,#30456);
#26068=AXIS2_PLACEMENT_3D('',#38598,#30461,#30462);
#26069=AXIS2_PLACEMENT_3D('',#38602,#30465,#30466);
#26070=AXIS2_PLACEMENT_3D('',#38612,#30472,#30473);
#26071=AXIS2_PLACEMENT_3D('',#38620,#30478,#30479);
#26072=AXIS2_PLACEMENT_3D('',#38624,#30482,#30483);
#26073=AXIS2_PLACEMENT_3D('',#38634,#30489,#30490);
#26074=AXIS2_PLACEMENT_3D('',#38642,#30495,#30496);
#26075=AXIS2_PLACEMENT_3D('',#38646,#30499,#30500);
#26076=AXIS2_PLACEMENT_3D('',#38656,#30506,#30507);
#26077=AXIS2_PLACEMENT_3D('',#38664,#30512,#30513);
#26078=AXIS2_PLACEMENT_3D('',#38668,#30516,#30517);
#26079=AXIS2_PLACEMENT_3D('',#38678,#30523,#30524);
#26080=AXIS2_PLACEMENT_3D('',#38686,#30529,#30530);
#26081=AXIS2_PLACEMENT_3D('',#38690,#30533,#30534);
#26082=AXIS2_PLACEMENT_3D('',#38700,#30540,#30541);
#26083=AXIS2_PLACEMENT_3D('',#38708,#30546,#30547);
#26084=AXIS2_PLACEMENT_3D('',#38712,#30550,#30551);
#26085=AXIS2_PLACEMENT_3D('',#38722,#30557,#30558);
#26086=AXIS2_PLACEMENT_3D('',#38730,#30563,#30564);
#26087=AXIS2_PLACEMENT_3D('',#38734,#30567,#30568);
#26088=AXIS2_PLACEMENT_3D('',#38744,#30574,#30575);
#26089=AXIS2_PLACEMENT_3D('',#38752,#30580,#30581);
#26090=AXIS2_PLACEMENT_3D('',#38756,#30584,#30585);
#26091=AXIS2_PLACEMENT_3D('',#38766,#30591,#30592);
#26092=AXIS2_PLACEMENT_3D('',#38774,#30597,#30598);
#26093=AXIS2_PLACEMENT_3D('',#38778,#30601,#30602);
#26094=AXIS2_PLACEMENT_3D('',#38788,#30608,#30609);
#26095=AXIS2_PLACEMENT_3D('',#38796,#30614,#30615);
#26096=AXIS2_PLACEMENT_3D('',#38800,#30618,#30619);
#26097=AXIS2_PLACEMENT_3D('',#38810,#30625,#30626);
#26098=AXIS2_PLACEMENT_3D('',#38818,#30631,#30632);
#26099=AXIS2_PLACEMENT_3D('',#38822,#30635,#30636);
#26100=AXIS2_PLACEMENT_3D('',#38832,#30642,#30643);
#26101=AXIS2_PLACEMENT_3D('',#38840,#30648,#30649);
#26102=AXIS2_PLACEMENT_3D('',#38844,#30652,#30653);
#26103=AXIS2_PLACEMENT_3D('',#38854,#30659,#30660);
#26104=AXIS2_PLACEMENT_3D('',#38860,#30664,#30665);
#26105=AXIS2_PLACEMENT_3D('',#38864,#30668,#30669);
#26106=AXIS2_PLACEMENT_3D('',#38874,#30675,#30676);
#26107=AXIS2_PLACEMENT_3D('',#38880,#30680,#30681);
#26108=AXIS2_PLACEMENT_3D('',#38884,#30684,#30685);
#26109=AXIS2_PLACEMENT_3D('',#38894,#30691,#30692);
#26110=AXIS2_PLACEMENT_3D('',#38900,#30696,#30697);
#26111=AXIS2_PLACEMENT_3D('',#38904,#30700,#30701);
#26112=AXIS2_PLACEMENT_3D('',#38914,#30707,#30708);
#26113=AXIS2_PLACEMENT_3D('',#38920,#30712,#30713);
#26114=AXIS2_PLACEMENT_3D('',#38924,#30716,#30717);
#26115=AXIS2_PLACEMENT_3D('',#38934,#30723,#30724);
#26116=AXIS2_PLACEMENT_3D('',#38940,#30728,#30729);
#26117=AXIS2_PLACEMENT_3D('',#38944,#30732,#30733);
#26118=AXIS2_PLACEMENT_3D('',#38954,#30739,#30740);
#26119=AXIS2_PLACEMENT_3D('',#38960,#30744,#30745);
#26120=AXIS2_PLACEMENT_3D('',#38964,#30748,#30749);
#26121=AXIS2_PLACEMENT_3D('',#38974,#30755,#30756);
#26122=AXIS2_PLACEMENT_3D('',#38980,#30760,#30761);
#26123=AXIS2_PLACEMENT_3D('',#38984,#30764,#30765);
#26124=AXIS2_PLACEMENT_3D('',#38994,#30771,#30772);
#26125=AXIS2_PLACEMENT_3D('',#39000,#30776,#30777);
#26126=AXIS2_PLACEMENT_3D('',#39004,#30780,#30781);
#26127=AXIS2_PLACEMENT_3D('',#39014,#30787,#30788);
#26128=AXIS2_PLACEMENT_3D('',#39020,#30792,#30793);
#26129=AXIS2_PLACEMENT_3D('',#39024,#30796,#30797);
#26130=AXIS2_PLACEMENT_3D('',#39034,#30803,#30804);
#26131=AXIS2_PLACEMENT_3D('',#39040,#30808,#30809);
#26132=AXIS2_PLACEMENT_3D('',#39044,#30812,#30813);
#26133=AXIS2_PLACEMENT_3D('',#39054,#30819,#30820);
#26134=AXIS2_PLACEMENT_3D('',#39060,#30824,#30825);
#26135=AXIS2_PLACEMENT_3D('',#39064,#30828,#30829);
#26136=AXIS2_PLACEMENT_3D('',#39074,#30835,#30836);
#26137=AXIS2_PLACEMENT_3D('',#39080,#30840,#30841);
#26138=AXIS2_PLACEMENT_3D('',#39084,#30844,#30845);
#26139=AXIS2_PLACEMENT_3D('',#39092,#30850,#30851);
#26140=AXIS2_PLACEMENT_3D('',#39536,#31079,#31080);
#26141=AXIS2_PLACEMENT_3D('',#39537,#31081,#31082);
#26142=AXIS2_PLACEMENT_3D('',#39542,#31086,#31087);
#26143=AXIS2_PLACEMENT_3D('',#39548,#31091,#31092);
#26144=AXIS2_PLACEMENT_3D('',#39553,#31096,#31097);
#26145=AXIS2_PLACEMENT_3D('',#39559,#31101,#31102);
#26146=AXIS2_PLACEMENT_3D('',#39564,#31106,#31107);
#26147=AXIS2_PLACEMENT_3D('',#39570,#31111,#31112);
#26148=AXIS2_PLACEMENT_3D('',#39575,#31116,#31117);
#26149=AXIS2_PLACEMENT_3D('',#39581,#31121,#31122);
#26150=AXIS2_PLACEMENT_3D('',#39586,#31126,#31127);
#26151=AXIS2_PLACEMENT_3D('',#39592,#31131,#31132);
#26152=AXIS2_PLACEMENT_3D('',#39597,#31136,#31137);
#26153=AXIS2_PLACEMENT_3D('',#39603,#31141,#31142);
#26154=AXIS2_PLACEMENT_3D('',#39608,#31146,#31147);
#26155=AXIS2_PLACEMENT_3D('',#39614,#31151,#31152);
#26156=AXIS2_PLACEMENT_3D('',#39619,#31156,#31157);
#26157=AXIS2_PLACEMENT_3D('',#39625,#31161,#31162);
#26158=AXIS2_PLACEMENT_3D('',#39630,#31166,#31167);
#26159=AXIS2_PLACEMENT_3D('',#39636,#31171,#31172);
#26160=AXIS2_PLACEMENT_3D('',#39641,#31176,#31177);
#26161=AXIS2_PLACEMENT_3D('',#39647,#31181,#31182);
#26162=AXIS2_PLACEMENT_3D('',#39652,#31186,#31187);
#26163=AXIS2_PLACEMENT_3D('',#39658,#31191,#31192);
#26164=AXIS2_PLACEMENT_3D('',#39663,#31196,#31197);
#26165=AXIS2_PLACEMENT_3D('',#39666,#31200,#31201);
#26166=AXIS2_PLACEMENT_3D('',#39668,#31203,#31204);
#26167=AXIS2_PLACEMENT_3D('',#39669,#31205,#31206);
#26168=AXIS2_PLACEMENT_3D('',#39671,#31208,#31209);
#26169=AXIS2_PLACEMENT_3D('',#39673,#31211,#31212);
#26170=AXIS2_PLACEMENT_3D('',#39675,#31214,#31215);
#26171=AXIS2_PLACEMENT_3D('',#39677,#31217,#31218);
#26172=AXIS2_PLACEMENT_3D('',#39679,#31220,#31221);
#26173=AXIS2_PLACEMENT_3D('',#39681,#31223,#31224);
#26174=AXIS2_PLACEMENT_3D('',#39683,#31226,#31227);
#26175=AXIS2_PLACEMENT_3D('',#39685,#31229,#31230);
#26176=AXIS2_PLACEMENT_3D('',#39687,#31232,#31233);
#26177=AXIS2_PLACEMENT_3D('',#39689,#31235,#31236);
#26178=AXIS2_PLACEMENT_3D('',#39691,#31238,#31239);
#26179=AXIS2_PLACEMENT_3D('',#39693,#31241,#31242);
#26180=AXIS2_PLACEMENT_3D('',#39695,#31244,#31245);
#26181=AXIS2_PLACEMENT_3D('',#39697,#31247,#31248);
#26182=AXIS2_PLACEMENT_3D('',#39699,#31250,#31251);
#26183=AXIS2_PLACEMENT_3D('',#39700,#31252,#31253);
#26184=AXIS2_PLACEMENT_3D('',#39702,#31255,#31256);
#26185=AXIS2_PLACEMENT_3D('',#39704,#31258,#31259);
#26186=AXIS2_PLACEMENT_3D('',#39706,#31261,#31262);
#26187=AXIS2_PLACEMENT_3D('',#39707,#31263,#31264);
#26188=AXIS2_PLACEMENT_3D('',#39709,#31266,#31267);
#26189=AXIS2_PLACEMENT_3D('',#39711,#31269,#31270);
#26190=AXIS2_PLACEMENT_3D('',#39713,#31272,#31273);
#26191=AXIS2_PLACEMENT_3D('',#39715,#31275,#31276);
#26192=AXIS2_PLACEMENT_3D('',#39717,#31278,#31279);
#26193=AXIS2_PLACEMENT_3D('',#39719,#31281,#31282);
#26194=AXIS2_PLACEMENT_3D('',#39721,#31284,#31285);
#26195=AXIS2_PLACEMENT_3D('',#39723,#31287,#31288);
#26196=AXIS2_PLACEMENT_3D('',#39725,#31290,#31291);
#26197=AXIS2_PLACEMENT_3D('',#39727,#31293,#31294);
#26198=AXIS2_PLACEMENT_3D('',#39729,#31296,#31297);
#26199=AXIS2_PLACEMENT_3D('',#39731,#31299,#31300);
#26200=AXIS2_PLACEMENT_3D('',#39733,#31302,#31303);
#26201=AXIS2_PLACEMENT_3D('',#39735,#31305,#31306);
#26202=AXIS2_PLACEMENT_3D('',#39737,#31308,#31309);
#26203=AXIS2_PLACEMENT_3D('',#39738,#31310,#31311);
#26204=AXIS2_PLACEMENT_3D('',#39740,#31313,#31314);
#26205=AXIS2_PLACEMENT_3D('',#39742,#31316,#31317);
#26206=AXIS2_PLACEMENT_3D('',#39744,#31319,#31320);
#26207=AXIS2_PLACEMENT_3D('',#39745,#31321,#31322);
#26208=AXIS2_PLACEMENT_3D('',#39747,#31324,#31325);
#26209=AXIS2_PLACEMENT_3D('',#39749,#31327,#31328);
#26210=AXIS2_PLACEMENT_3D('',#39751,#31330,#31331);
#26211=AXIS2_PLACEMENT_3D('',#39753,#31333,#31334);
#26212=AXIS2_PLACEMENT_3D('',#39755,#31336,#31337);
#26213=AXIS2_PLACEMENT_3D('',#39757,#31339,#31340);
#26214=AXIS2_PLACEMENT_3D('',#39759,#31342,#31343);
#26215=AXIS2_PLACEMENT_3D('',#39761,#31345,#31346);
#26216=AXIS2_PLACEMENT_3D('',#39763,#31348,#31349);
#26217=AXIS2_PLACEMENT_3D('',#39765,#31351,#31352);
#26218=AXIS2_PLACEMENT_3D('',#39767,#31354,#31355);
#26219=AXIS2_PLACEMENT_3D('',#39769,#31357,#31358);
#26220=AXIS2_PLACEMENT_3D('',#39771,#31360,#31361);
#26221=AXIS2_PLACEMENT_3D('',#39773,#31363,#31364);
#26222=AXIS2_PLACEMENT_3D('',#39775,#31366,#31367);
#26223=AXIS2_PLACEMENT_3D('',#39776,#31368,#31369);
#26224=AXIS2_PLACEMENT_3D('',#39778,#31371,#31372);
#26225=AXIS2_PLACEMENT_3D('',#39780,#31374,#31375);
#26226=AXIS2_PLACEMENT_3D('',#39782,#31377,#31378);
#26227=AXIS2_PLACEMENT_3D('',#39783,#31379,#31380);
#26228=AXIS2_PLACEMENT_3D('',#39785,#31382,#31383);
#26229=AXIS2_PLACEMENT_3D('',#39787,#31385,#31386);
#26230=AXIS2_PLACEMENT_3D('',#39789,#31388,#31389);
#26231=AXIS2_PLACEMENT_3D('',#39791,#31391,#31392);
#26232=AXIS2_PLACEMENT_3D('',#39793,#31394,#31395);
#26233=AXIS2_PLACEMENT_3D('',#39795,#31397,#31398);
#26234=AXIS2_PLACEMENT_3D('',#39797,#31400,#31401);
#26235=AXIS2_PLACEMENT_3D('',#39799,#31403,#31404);
#26236=AXIS2_PLACEMENT_3D('',#39801,#31406,#31407);
#26237=AXIS2_PLACEMENT_3D('',#39803,#31409,#31410);
#26238=AXIS2_PLACEMENT_3D('',#39805,#31412,#31413);
#26239=AXIS2_PLACEMENT_3D('',#39807,#31415,#31416);
#26240=AXIS2_PLACEMENT_3D('',#39809,#31418,#31419);
#26241=AXIS2_PLACEMENT_3D('',#39811,#31421,#31422);
#26242=AXIS2_PLACEMENT_3D('',#39813,#31424,#31425);
#26243=AXIS2_PLACEMENT_3D('',#39814,#31426,#31427);
#26244=AXIS2_PLACEMENT_3D('',#39816,#31429,#31430);
#26245=AXIS2_PLACEMENT_3D('',#39818,#31432,#31433);
#26246=AXIS2_PLACEMENT_3D('',#39820,#31435,#31436);
#26247=AXIS2_PLACEMENT_3D('',#39821,#31437,#31438);
#26248=AXIS2_PLACEMENT_3D('',#39823,#31440,#31441);
#26249=AXIS2_PLACEMENT_3D('',#39825,#31443,#31444);
#26250=AXIS2_PLACEMENT_3D('',#39827,#31446,#31447);
#26251=AXIS2_PLACEMENT_3D('',#39829,#31449,#31450);
#26252=AXIS2_PLACEMENT_3D('',#39831,#31452,#31453);
#26253=AXIS2_PLACEMENT_3D('',#39833,#31455,#31456);
#26254=AXIS2_PLACEMENT_3D('',#39835,#31458,#31459);
#26255=AXIS2_PLACEMENT_3D('',#39837,#31461,#31462);
#26256=AXIS2_PLACEMENT_3D('',#39839,#31464,#31465);
#26257=AXIS2_PLACEMENT_3D('',#39841,#31467,#31468);
#26258=AXIS2_PLACEMENT_3D('',#39843,#31470,#31471);
#26259=AXIS2_PLACEMENT_3D('',#39845,#31473,#31474);
#26260=AXIS2_PLACEMENT_3D('',#39847,#31476,#31477);
#26261=AXIS2_PLACEMENT_3D('',#39849,#31479,#31480);
#26262=AXIS2_PLACEMENT_3D('',#39851,#31482,#31483);
#26263=AXIS2_PLACEMENT_3D('',#39852,#31484,#31485);
#26264=AXIS2_PLACEMENT_3D('',#39854,#31487,#31488);
#26265=AXIS2_PLACEMENT_3D('',#39856,#31490,#31491);
#26266=AXIS2_PLACEMENT_3D('',#39858,#31493,#31494);
#26267=AXIS2_PLACEMENT_3D('',#39859,#31495,#31496);
#26268=AXIS2_PLACEMENT_3D('',#39861,#31498,#31499);
#26269=AXIS2_PLACEMENT_3D('',#39863,#31501,#31502);
#26270=AXIS2_PLACEMENT_3D('',#39865,#31504,#31505);
#26271=AXIS2_PLACEMENT_3D('',#39867,#31507,#31508);
#26272=AXIS2_PLACEMENT_3D('',#39869,#31510,#31511);
#26273=AXIS2_PLACEMENT_3D('',#39871,#31513,#31514);
#26274=AXIS2_PLACEMENT_3D('',#39873,#31516,#31517);
#26275=AXIS2_PLACEMENT_3D('',#39875,#31519,#31520);
#26276=AXIS2_PLACEMENT_3D('',#39877,#31522,#31523);
#26277=AXIS2_PLACEMENT_3D('',#39879,#31525,#31526);
#26278=AXIS2_PLACEMENT_3D('',#39881,#31528,#31529);
#26279=AXIS2_PLACEMENT_3D('',#39883,#31531,#31532);
#26280=AXIS2_PLACEMENT_3D('',#39885,#31534,#31535);
#26281=AXIS2_PLACEMENT_3D('',#39887,#31537,#31538);
#26282=AXIS2_PLACEMENT_3D('',#39889,#31540,#31541);
#26283=AXIS2_PLACEMENT_3D('',#39890,#31542,#31543);
#26284=AXIS2_PLACEMENT_3D('',#39892,#31545,#31546);
#26285=AXIS2_PLACEMENT_3D('',#39894,#31548,#31549);
#26286=AXIS2_PLACEMENT_3D('',#39896,#31551,#31552);
#26287=AXIS2_PLACEMENT_3D('',#39897,#31553,#31554);
#26288=AXIS2_PLACEMENT_3D('',#39899,#31556,#31557);
#26289=AXIS2_PLACEMENT_3D('',#39901,#31559,#31560);
#26290=AXIS2_PLACEMENT_3D('',#39903,#31562,#31563);
#26291=AXIS2_PLACEMENT_3D('',#39905,#31565,#31566);
#26292=AXIS2_PLACEMENT_3D('',#39907,#31568,#31569);
#26293=AXIS2_PLACEMENT_3D('',#39909,#31571,#31572);
#26294=AXIS2_PLACEMENT_3D('',#39911,#31574,#31575);
#26295=AXIS2_PLACEMENT_3D('',#39913,#31577,#31578);
#26296=AXIS2_PLACEMENT_3D('',#39915,#31580,#31581);
#26297=AXIS2_PLACEMENT_3D('',#39917,#31583,#31584);
#26298=AXIS2_PLACEMENT_3D('',#39919,#31586,#31587);
#26299=AXIS2_PLACEMENT_3D('',#39921,#31589,#31590);
#26300=AXIS2_PLACEMENT_3D('',#39923,#31592,#31593);
#26301=AXIS2_PLACEMENT_3D('',#39925,#31595,#31596);
#26302=AXIS2_PLACEMENT_3D('',#39927,#31598,#31599);
#26303=AXIS2_PLACEMENT_3D('',#39928,#31600,#31601);
#26304=AXIS2_PLACEMENT_3D('',#39930,#31603,#31604);
#26305=AXIS2_PLACEMENT_3D('',#39932,#31606,#31607);
#26306=AXIS2_PLACEMENT_3D('',#39934,#31609,#31610);
#26307=AXIS2_PLACEMENT_3D('',#39935,#31611,#31612);
#26308=AXIS2_PLACEMENT_3D('',#39937,#31614,#31615);
#26309=AXIS2_PLACEMENT_3D('',#39939,#31617,#31618);
#26310=AXIS2_PLACEMENT_3D('',#39941,#31620,#31621);
#26311=AXIS2_PLACEMENT_3D('',#39943,#31623,#31624);
#26312=AXIS2_PLACEMENT_3D('',#39945,#31626,#31627);
#26313=AXIS2_PLACEMENT_3D('',#39947,#31629,#31630);
#26314=AXIS2_PLACEMENT_3D('',#39949,#31632,#31633);
#26315=AXIS2_PLACEMENT_3D('',#39951,#31635,#31636);
#26316=AXIS2_PLACEMENT_3D('',#39953,#31638,#31639);
#26317=AXIS2_PLACEMENT_3D('',#39955,#31641,#31642);
#26318=AXIS2_PLACEMENT_3D('',#39957,#31644,#31645);
#26319=AXIS2_PLACEMENT_3D('',#39959,#31647,#31648);
#26320=AXIS2_PLACEMENT_3D('',#39961,#31650,#31651);
#26321=AXIS2_PLACEMENT_3D('',#39963,#31653,#31654);
#26322=AXIS2_PLACEMENT_3D('',#39965,#31656,#31657);
#26323=AXIS2_PLACEMENT_3D('',#39966,#31658,#31659);
#26324=AXIS2_PLACEMENT_3D('',#39968,#31661,#31662);
#26325=AXIS2_PLACEMENT_3D('',#39970,#31664,#31665);
#26326=AXIS2_PLACEMENT_3D('',#39972,#31667,#31668);
#26327=AXIS2_PLACEMENT_3D('',#39973,#31669,#31670);
#26328=AXIS2_PLACEMENT_3D('',#39975,#31672,#31673);
#26329=AXIS2_PLACEMENT_3D('',#39977,#31675,#31676);
#26330=AXIS2_PLACEMENT_3D('',#39979,#31678,#31679);
#26331=AXIS2_PLACEMENT_3D('',#39981,#31681,#31682);
#26332=AXIS2_PLACEMENT_3D('',#39983,#31684,#31685);
#26333=AXIS2_PLACEMENT_3D('',#39985,#31687,#31688);
#26334=AXIS2_PLACEMENT_3D('',#39987,#31690,#31691);
#26335=AXIS2_PLACEMENT_3D('',#39989,#31693,#31694);
#26336=AXIS2_PLACEMENT_3D('',#39991,#31696,#31697);
#26337=AXIS2_PLACEMENT_3D('',#39993,#31699,#31700);
#26338=AXIS2_PLACEMENT_3D('',#39995,#31702,#31703);
#26339=AXIS2_PLACEMENT_3D('',#39997,#31705,#31706);
#26340=AXIS2_PLACEMENT_3D('',#39999,#31708,#31709);
#26341=AXIS2_PLACEMENT_3D('',#40001,#31711,#31712);
#26342=AXIS2_PLACEMENT_3D('',#40003,#31714,#31715);
#26343=AXIS2_PLACEMENT_3D('',#40004,#31716,#31717);
#26344=AXIS2_PLACEMENT_3D('',#40006,#31719,#31720);
#26345=AXIS2_PLACEMENT_3D('',#40008,#31722,#31723);
#26346=AXIS2_PLACEMENT_3D('',#40010,#31725,#31726);
#26347=AXIS2_PLACEMENT_3D('',#40011,#31727,#31728);
#26348=AXIS2_PLACEMENT_3D('',#40013,#31730,#31731);
#26349=AXIS2_PLACEMENT_3D('',#40015,#31733,#31734);
#26350=AXIS2_PLACEMENT_3D('',#40017,#31736,#31737);
#26351=AXIS2_PLACEMENT_3D('',#40019,#31739,#31740);
#26352=AXIS2_PLACEMENT_3D('',#40021,#31742,#31743);
#26353=AXIS2_PLACEMENT_3D('',#40023,#31745,#31746);
#26354=AXIS2_PLACEMENT_3D('',#40025,#31748,#31749);
#26355=AXIS2_PLACEMENT_3D('',#40027,#31751,#31752);
#26356=AXIS2_PLACEMENT_3D('',#40029,#31754,#31755);
#26357=AXIS2_PLACEMENT_3D('',#40031,#31757,#31758);
#26358=AXIS2_PLACEMENT_3D('',#40033,#31760,#31761);
#26359=AXIS2_PLACEMENT_3D('',#40035,#31763,#31764);
#26360=AXIS2_PLACEMENT_3D('',#40037,#31766,#31767);
#26361=AXIS2_PLACEMENT_3D('',#40039,#31769,#31770);
#26362=AXIS2_PLACEMENT_3D('',#40041,#31772,#31773);
#26363=AXIS2_PLACEMENT_3D('',#40042,#31774,#31775);
#26364=AXIS2_PLACEMENT_3D('',#40044,#31777,#31778);
#26365=AXIS2_PLACEMENT_3D('',#40046,#31780,#31781);
#26366=AXIS2_PLACEMENT_3D('',#40048,#31783,#31784);
#26367=AXIS2_PLACEMENT_3D('',#40049,#31785,#31786);
#26368=AXIS2_PLACEMENT_3D('',#40051,#31788,#31789);
#26369=AXIS2_PLACEMENT_3D('',#40053,#31791,#31792);
#26370=AXIS2_PLACEMENT_3D('',#40055,#31794,#31795);
#26371=AXIS2_PLACEMENT_3D('',#40057,#31797,#31798);
#26372=AXIS2_PLACEMENT_3D('',#40059,#31800,#31801);
#26373=AXIS2_PLACEMENT_3D('',#40061,#31803,#31804);
#26374=AXIS2_PLACEMENT_3D('',#40063,#31806,#31807);
#26375=AXIS2_PLACEMENT_3D('',#40065,#31809,#31810);
#26376=AXIS2_PLACEMENT_3D('',#40067,#31812,#31813);
#26377=AXIS2_PLACEMENT_3D('',#40069,#31815,#31816);
#26378=AXIS2_PLACEMENT_3D('',#40071,#31818,#31819);
#26379=AXIS2_PLACEMENT_3D('',#40073,#31821,#31822);
#26380=AXIS2_PLACEMENT_3D('',#40075,#31824,#31825);
#26381=AXIS2_PLACEMENT_3D('',#40077,#31827,#31828);
#26382=AXIS2_PLACEMENT_3D('',#40079,#31830,#31831);
#26383=AXIS2_PLACEMENT_3D('',#40080,#31832,#31833);
#26384=AXIS2_PLACEMENT_3D('',#40082,#31835,#31836);
#26385=AXIS2_PLACEMENT_3D('',#40084,#31838,#31839);
#26386=AXIS2_PLACEMENT_3D('',#40086,#31841,#31842);
#26387=AXIS2_PLACEMENT_3D('',#40087,#31843,#31844);
#26388=AXIS2_PLACEMENT_3D('',#40089,#31846,#31847);
#26389=AXIS2_PLACEMENT_3D('',#40091,#31849,#31850);
#26390=AXIS2_PLACEMENT_3D('',#40093,#31852,#31853);
#26391=AXIS2_PLACEMENT_3D('',#40095,#31855,#31856);
#26392=AXIS2_PLACEMENT_3D('',#40097,#31858,#31859);
#26393=AXIS2_PLACEMENT_3D('',#40099,#31861,#31862);
#26394=AXIS2_PLACEMENT_3D('',#40101,#31864,#31865);
#26395=AXIS2_PLACEMENT_3D('',#40103,#31867,#31868);
#26396=AXIS2_PLACEMENT_3D('',#40105,#31870,#31871);
#26397=AXIS2_PLACEMENT_3D('',#40107,#31873,#31874);
#26398=AXIS2_PLACEMENT_3D('',#40109,#31876,#31877);
#26399=AXIS2_PLACEMENT_3D('',#40111,#31879,#31880);
#26400=AXIS2_PLACEMENT_3D('',#40113,#31882,#31883);
#26401=AXIS2_PLACEMENT_3D('',#40115,#31885,#31886);
#26402=AXIS2_PLACEMENT_3D('',#40117,#31888,#31889);
#26403=AXIS2_PLACEMENT_3D('',#40118,#31890,#31891);
#26404=AXIS2_PLACEMENT_3D('',#40119,#31892,#31893);
#26405=AXIS2_PLACEMENT_3D('',#40122,#31895,#31896);
#26406=AXIS2_PLACEMENT_3D('',#40123,#31897,#31898);
#26407=AXIS2_PLACEMENT_3D('',#40124,#31899,#31900);
#26408=AXIS2_PLACEMENT_3D('',#40126,#31901,#31902);
#26409=AXIS2_PLACEMENT_3D('',#40128,#31904,#31905);
#30202=DIRECTION('axis',(0.,0.,1.));
#30203=DIRECTION('refdir',(1.,0.,0.));
#30204=DIRECTION('center_axis',(0.414495032230687,-0.707106781186548,-0.572882071857796));
#30205=DIRECTION('ref_axis',(-0.810177595661694,0.,-0.586184496116911));
#30206=DIRECTION('',(0.451594888615274,-0.386714295024759,0.80406101173982));
#30207=DIRECTION('',(-0.810177595661694,0.,-0.586184496116911));
#30208=DIRECTION('',(-0.384785213588102,-0.706639907076676,0.593801634496425));
#30209=DIRECTION('',(0.810177595661694,0.,0.586184496116911));
#30210=DIRECTION('',(0.681078899711059,-0.1764913880685,0.710621082086668));
#30211=DIRECTION('',(0.547096153529848,-0.309436927624307,0.777775408852244));
#30212=DIRECTION('center_axis',(0.,1.,0.));
#30213=DIRECTION('ref_axis',(1.,0.,0.));
#30214=DIRECTION('',(-0.54380964897583,0.,0.839208594856359));
#30215=DIRECTION('',(0.48969323063785,0.,0.871894798623931));
#30216=DIRECTION('',(0.414834765185058,0.,0.909896762052629));
#30217=DIRECTION('',(0.346203891732264,0.,0.938159296361463));
#30218=DIRECTION('',(0.281816316675586,0.,0.959468375536894));
#30219=DIRECTION('',(0.220607484589178,0.,0.975362669853237));
#30220=DIRECTION('',(0.161938741065869,0.,0.986800812799626));
#30221=DIRECTION('',(-0.691221298772304,0.,0.722643145766656));
#30222=DIRECTION('',(-0.701850027448819,0.,0.712324742635051));
#30223=DIRECTION('',(-0.712324742635051,0.,0.701850027448819));
#30224=DIRECTION('',(-0.722643145766653,0.,0.691221298772308));
#30225=DIRECTION('',(-0.986800812799626,0.,-0.161938741065865));
#30226=DIRECTION('',(-0.975362669853236,0.,-0.220607484589183));
#30227=DIRECTION('',(-0.959468375536896,0.,-0.28181631667558));
#30228=DIRECTION('',(-0.938159296361463,0.,-0.346203891732262));
#30229=DIRECTION('',(-0.909896762052626,0.,-0.414834765185062));
#30230=DIRECTION('',(-0.87189479862393,0.,-0.489693230637852));
#30231=DIRECTION('',(0.58618449611691,0.,0.810177595661694));
#30232=DIRECTION('',(-0.839208594856358,0.,0.543809648975832));
#30233=DIRECTION('',(-0.890557268264346,0.,0.454871137731935));
#30234=DIRECTION('',(-0.408542131361568,0.,-0.912739462772673));
#30235=DIRECTION('',(-0.011860621518292,0.,0.999929660354767));
#30236=DIRECTION('',(-0.0956909360031075,0.,0.995411093351309));
#30237=DIRECTION('',(-0.169258283051556,0.,0.985571729311692));
#30238=DIRECTION('',(-0.235674098326445,0.,0.971832145680527));
#30239=DIRECTION('',(-0.296629649007403,0.,0.954992592290508));
#30240=DIRECTION('',(-0.353157342779898,0.,0.935563942892543));
#30241=DIRECTION('',(-0.959936777257016,0.,0.280216672718478));
#30242=DIRECTION('',(-0.963982324735009,0.,0.265966309141754));
#30243=DIRECTION('',(-0.967816336590576,0.,0.251657582099957));
#30244=DIRECTION('',(-0.971437971490777,0.,0.237293631490364));
#30245=DIRECTION('',(-0.773625201826672,0.,-0.633643470019727));
#30246=DIRECTION('',(-0.734385107701324,0.,-0.678733020845837));
#30247=DIRECTION('',(-0.690015829004958,0.,-0.723794277210452));
#30248=DIRECTION('',(-0.639367837579427,0.,-0.768901013309911));
#30249=DIRECTION('',(-0.580576328166257,0.,-0.814205826049523));
#30250=DIRECTION('',(-0.510236429716897,0.,-0.860034177105627));
#30251=DIRECTION('',(0.10256186711098,0.,0.99472662747848));
#30252=DIRECTION('',(-0.998680786707765,0.,0.0513486734079894));
#30253=DIRECTION('',(-0.998680786707765,0.,-0.0513486734079893));
#30254=DIRECTION('',(0.10256186711098,0.,-0.99472662747848));
#30255=DIRECTION('',(-0.510236429716897,0.,0.860034177105627));
#30256=DIRECTION('',(-0.580576328166257,0.,0.814205826049523));
#30257=DIRECTION('',(-0.639367837579427,0.,0.768901013309911));
#30258=DIRECTION('',(-0.690015829004958,0.,0.723794277210452));
#30259=DIRECTION('',(-0.734385107701324,0.,0.678733020845836));
#30260=DIRECTION('',(-0.773625201826672,0.,0.633643470019727));
#30261=DIRECTION('',(-0.971437971490777,0.,-0.237293631490364));
#30262=DIRECTION('',(-0.967816336590576,0.,-0.251657582099957));
#30263=DIRECTION('',(-0.963982324735007,0.,-0.265966309141762));
#30264=DIRECTION('',(-0.959936777257018,0.,-0.28021667271847));
#30265=DIRECTION('',(-0.353157342779898,0.,-0.935563942892543));
#30266=DIRECTION('',(-0.296629649007399,0.,-0.954992592290509));
#30267=DIRECTION('',(-0.235674098326447,0.,-0.971832145680527));
#30268=DIRECTION('',(-0.169258283051554,0.,-0.985571729311692));
#30269=DIRECTION('',(-0.0956909360031101,0.,-0.995411093351309));
#30270=DIRECTION('',(-0.0118606215182901,0.,-0.999929660354767));
#30271=DIRECTION('',(-0.408542131361568,0.,0.912739462772673));
#30272=DIRECTION('',(-0.890557268264346,0.,-0.454871137731935));
#30273=DIRECTION('',(-0.839208594856359,0.,-0.54380964897583));
#30274=DIRECTION('',(0.586184496116912,0.,-0.810177595661693));
#30275=DIRECTION('',(-0.871894798623918,0.,0.489693230637874));
#30276=DIRECTION('',(-0.909896762052635,0.,0.414834765185043));
#30277=DIRECTION('',(-0.938159296361459,0.,0.346203891732275));
#30278=DIRECTION('',(-0.9594683755369,0.,0.281816316675565));
#30279=DIRECTION('',(-0.975362669853236,0.,0.220607484589184));
#30280=DIRECTION('',(-0.986800812799626,0.,0.161938741065868));
#30281=DIRECTION('',(-0.722643145766652,0.,-0.691221298772308));
#30282=DIRECTION('',(-0.712324742635051,0.,-0.701850027448819));
#30283=DIRECTION('',(-0.701850027448815,0.,-0.712324742635055));
#30284=DIRECTION('',(-0.691221298772312,0.,-0.722643145766649));
#30285=DIRECTION('',(0.161938741065865,0.,-0.986800812799626));
#30286=DIRECTION('',(0.220607484589187,0.,-0.975362669853235));
#30287=DIRECTION('',(0.281816316675565,0.,-0.9594683755369));
#30288=DIRECTION('',(0.346203891732272,0.,-0.93815929636146));
#30289=DIRECTION('',(0.414834765185049,0.,-0.909896762052633));
#30290=DIRECTION('',(0.489693230637868,0.,-0.871894798623921));
#30291=DIRECTION('',(-0.810177595661692,0.,0.586184496116913));
#30292=DIRECTION('',(-0.543809648975831,0.,-0.839208594856358));
#30293=DIRECTION('',(-0.454871137731934,0.,-0.890557268264347));
#30294=DIRECTION('',(0.912739462772673,0.,-0.408542131361568));
#30295=DIRECTION('',(-0.999929660354767,0.,-0.0118606215182919));
#30296=DIRECTION('',(-0.995411093351309,0.,-0.0956909360031137));
#30297=DIRECTION('',(-0.985571729311693,0.,-0.169258283051549));
#30298=DIRECTION('',(-0.971832145680526,0.,-0.235674098326448));
#30299=DIRECTION('',(-0.954992592290512,0.,-0.296629649007392));
#30300=DIRECTION('',(-0.93556394289254,0.,-0.353157342779906));
#30301=DIRECTION('',(-0.280216672718464,0.,-0.95993677725702));
#30302=DIRECTION('',(-0.265966309141754,0.,-0.963982324735009));
#30303=DIRECTION('',(-0.251657582099958,0.,-0.967816336590576));
#30304=DIRECTION('',(-0.237293631490368,0.,-0.971437971490776));
#30305=DIRECTION('',(0.633643470019724,0.,-0.773625201826675));
#30306=DIRECTION('',(0.678733020845843,0.,-0.734385107701318));
#30307=DIRECTION('',(0.723794277210445,0.,-0.690015829004965));
#30308=DIRECTION('',(0.768901013309918,0.,-0.639367837579419));
#30309=DIRECTION('',(0.814205826049519,0.,-0.580576328166263));
#30310=DIRECTION('',(0.86003417710563,0.,-0.510236429716893));
#30311=DIRECTION('',(-0.99472662747848,0.,0.102561867110979));
#30312=DIRECTION('',(-0.0513486734079878,0.,-0.998680786707765));
#30313=DIRECTION('',(0.0513486734079878,0.,-0.998680786707765));
#30314=DIRECTION('',(0.99472662747848,0.,0.102561867110979));
#30315=DIRECTION('',(-0.86003417710563,0.,-0.510236429716893));
#30316=DIRECTION('',(-0.814205826049522,0.,-0.580576328166259));
#30317=DIRECTION('',(-0.768901013309911,0.,-0.639367837579427));
#30318=DIRECTION('',(-0.723794277210454,0.,-0.690015829004956));
#30319=DIRECTION('',(-0.678733020845838,0.,-0.734385107701322));
#30320=DIRECTION('',(-0.63364347001972,0.,-0.773625201826678));
#30321=DIRECTION('',(0.237293631490357,0.,-0.971437971490779));
#30322=DIRECTION('',(0.251657582099958,0.,-0.967816336590576));
#30323=DIRECTION('',(0.265966309141754,0.,-0.963982324735009));
#30324=DIRECTION('',(0.280216672718478,0.,-0.959936777257016));
#30325=DIRECTION('',(0.935563942892542,0.,-0.3531573427799));
#30326=DIRECTION('',(0.95499259229051,0.,-0.296629649007398));
#30327=DIRECTION('',(0.971832145680524,0.,-0.235674098326456));
#30328=DIRECTION('',(0.985571729311695,0.,-0.169258283051542));
#30329=DIRECTION('',(0.99541109335131,0.,-0.0956909360031057));
#30330=DIRECTION('',(0.999929660354767,0.,-0.011860621518292));
#30331=DIRECTION('',(-0.912739462772673,0.,-0.408542131361568));
#30332=DIRECTION('',(0.454871137731933,0.,-0.890557268264347));
#30333=DIRECTION('',(0.543809648975832,0.,-0.839208594856358));
#30334=DIRECTION('',(0.810177595661692,0.,0.586184496116913));
#30335=DIRECTION('',(-0.489693230637875,0.,-0.871894798623917));
#30336=DIRECTION('',(-0.414834765185046,0.,-0.909896762052634));
#30337=DIRECTION('',(-0.346203891732269,0.,-0.938159296361461));
#30338=DIRECTION('',(-0.281816316675564,0.,-0.9594683755369));
#30339=DIRECTION('',(-0.22060748458919,0.,-0.975362669853235));
#30340=DIRECTION('',(-0.161938741065865,0.,-0.986800812799626));
#30341=DIRECTION('',(0.691221298772293,0.,-0.722643145766667));
#30342=DIRECTION('',(0.701850027448823,0.,-0.712324742635048));
#30343=DIRECTION('',(0.71232474263504,0.,-0.701850027448831));
#30344=DIRECTION('',(0.722643145766668,0.,-0.691221298772292));
#30345=DIRECTION('',(0.986800812799626,0.,0.161938741065863));
#30346=DIRECTION('',(0.975362669853233,0.,0.2206074845892));
#30347=DIRECTION('',(0.959468375536898,0.,0.281816316675571));
#30348=DIRECTION('',(0.938159296361463,0.,0.346203891732263));
#30349=DIRECTION('',(0.909896762052627,0.,0.414834765185061));
#30350=DIRECTION('',(0.871894798623937,0.,0.48969323063784));
#30351=DIRECTION('',(-0.586184496116911,0.,-0.810177595661694));
#30352=DIRECTION('',(0.839208594856358,0.,-0.543809648975832));
#30353=DIRECTION('',(0.890557268264346,0.,-0.454871137731935));
#30354=DIRECTION('',(0.408542131361568,0.,0.912739462772673));
#30355=DIRECTION('',(0.0118606215182939,0.,-0.999929660354767));
#30356=DIRECTION('',(0.0956909360031021,0.,-0.99541109335131));
#30357=DIRECTION('',(0.169258283051555,0.,-0.985571729311692));
#30358=DIRECTION('',(0.235674098326432,0.,-0.97183214568053));
#30359=DIRECTION('',(0.296629649007409,0.,-0.954992592290506));
#30360=DIRECTION('',(0.3531573427799,0.,-0.935563942892542));
#30361=DIRECTION('',(0.959936777257014,0.,-0.280216672718486));
#30362=DIRECTION('',(0.963982324735007,0.,-0.265966309141761));
#30363=DIRECTION('',(0.967816336590582,0.,-0.251657582099936));
#30364=DIRECTION('',(0.971437971490773,0.,-0.237293631490379));
#30365=DIRECTION('',(0.773625201826676,0.,0.633643470019722));
#30366=DIRECTION('',(0.734385107701325,0.,0.678733020845836));
#30367=DIRECTION('',(0.69001582900495,0.,0.723794277210459));
#30368=DIRECTION('',(0.639367837579431,0.,0.768901013309907));
#30369=DIRECTION('',(0.580576328166246,0.,0.814205826049531));
#30370=DIRECTION('',(0.510236429716899,0.,0.860034177105626));
#30371=DIRECTION('',(-0.10256186711098,0.,-0.99472662747848));
#30372=DIRECTION('',(0.998680786707765,0.,-0.0513486734079864));
#30373=DIRECTION('',(0.998680786707765,0.,0.0513486734079863));
#30374=DIRECTION('',(-0.102561867110979,0.,0.99472662747848));
#30375=DIRECTION('',(0.5102364297169,0.,-0.860034177105626));
#30376=DIRECTION('',(0.580576328166246,0.,-0.814205826049532));
#30377=DIRECTION('',(0.639367837579431,0.,-0.768901013309908));
#30378=DIRECTION('',(0.69001582900495,0.,-0.723794277210459));
#30379=DIRECTION('',(0.734385107701325,0.,-0.678733020845836));
#30380=DIRECTION('',(0.77362520182667,0.,-0.63364347001973));
#30381=DIRECTION('',(0.971437971490766,0.,0.237293631490407));
#30382=DIRECTION('',(0.967816336590582,0.,0.251657582099936));
#30383=DIRECTION('',(0.963982324735007,0.,0.265966309141763));
#30384=DIRECTION('',(0.959936777257023,0.,0.280216672718455));
#30385=DIRECTION('',(0.353157342779899,0.,0.935563942892543));
#30386=DIRECTION('',(0.296629649007407,0.,0.954992592290507));
#30387=DIRECTION('',(0.235674098326432,0.,0.97183214568053));
#30388=DIRECTION('',(0.169258283051555,0.,0.985571729311692));
#30389=DIRECTION('',(0.0956909360031021,0.,0.99541109335131));
#30390=DIRECTION('',(0.0118606215182939,0.,0.999929660354767));
#30391=DIRECTION('',(0.408542131361567,0.,-0.912739462772673));
#30392=DIRECTION('',(0.890557268264349,0.,0.45487113773193));
#30393=DIRECTION('',(0.839208594856358,0.,0.543809648975832));
#30394=DIRECTION('',(-0.586184496116913,0.,0.810177595661693));
#30395=DIRECTION('',(0.87189479862393,0.,-0.489693230637852));
#30396=DIRECTION('',(0.909896762052632,0.,-0.41483476518505));
#30397=DIRECTION('',(0.938159296361463,0.,-0.346203891732262));
#30398=DIRECTION('',(0.95946837553689,0.,-0.2818163166756));
#30399=DIRECTION('',(0.975362669853239,0.,-0.220607484589173));
#30400=DIRECTION('',(0.986800812799624,0.,-0.161938741065875));
#30401=DIRECTION('',(0.722643145766637,0.,0.691221298772324));
#30402=DIRECTION('',(0.712324742635063,0.,0.701850027448807));
#30403=DIRECTION('',(0.701850027448807,0.,0.712324742635063));
#30404=DIRECTION('',(0.691221298772316,0.,0.722643145766645));
#30405=DIRECTION('',(-0.161938741065862,0.,0.986800812799627));
#30406=DIRECTION('',(-0.220607484589184,0.,0.975362669853236));
#30407=DIRECTION('',(-0.281816316675577,0.,0.959468375536896));
#30408=DIRECTION('',(-0.346203891732263,0.,0.938159296361463));
#30409=DIRECTION('',(-0.414834765185061,0.,0.909896762052627));
#30410=DIRECTION('',(-0.48969323063785,0.,0.871894798623931));
#30411=DIRECTION('',(0.810177595661695,0.,-0.58618449611691));
#30412=DIRECTION('',(0.543809648975831,0.,0.839208594856359));
#30413=DIRECTION('',(0.454871137731933,0.,0.890557268264347));
#30414=DIRECTION('',(-0.912739462772673,0.,0.408542131361568));
#30415=DIRECTION('',(0.999929660354767,0.,0.0118606215182843));
#30416=DIRECTION('',(0.99541109335131,0.,0.0956909360030991));
#30417=DIRECTION('',(0.98557172931169,0.,0.169258283051569));
#30418=DIRECTION('',(0.971832145680534,0.,0.235674098326418));
#30419=DIRECTION('',(0.954992592290506,0.,0.29662964900741));
#30420=DIRECTION('',(0.935563942892542,0.,0.3531573427799));
#30421=DIRECTION('',(0.280216672718472,0.,0.959936777257017));
#30422=DIRECTION('',(0.265966309141757,0.,0.963982324735009));
#30423=DIRECTION('',(0.251657582099955,0.,0.967816336590577));
#30424=DIRECTION('',(0.237293631490361,0.,0.971437971490778));
#30425=DIRECTION('',(-0.633643470019724,0.,0.773625201826675));
#30426=DIRECTION('',(-0.678733020845831,0.,0.734385107701329));
#30427=DIRECTION('',(-0.723794277210464,0.,0.690015829004945));
#30428=DIRECTION('',(-0.768901013309907,0.,0.639367837579431));
#30429=DIRECTION('',(-0.814205826049529,0.,0.580576328166249));
#30430=DIRECTION('',(-0.860034177105627,0.,0.510236429716898));
#30431=DIRECTION('',(0.99472662747848,0.,-0.102561867110979));
#30432=DIRECTION('',(0.0513486734079878,0.,0.998680786707765));
#30433=DIRECTION('',(-0.0513486734079865,0.,0.998680786707765));
#30434=DIRECTION('',(-0.99472662747848,0.,-0.102561867110979));
#30435=DIRECTION('',(0.860034177105627,0.,0.510236429716898));
#30436=DIRECTION('',(0.814205826049526,0.,0.580576328166254));
#30437=DIRECTION('',(0.768901013309911,0.,0.639367837579427));
#30438=DIRECTION('',(0.723794277210468,0.,0.690015829004942));
#30439=DIRECTION('',(0.678733020845828,0.,0.734385107701332));
#30440=DIRECTION('',(0.633643470019728,0.,0.773625201826672));
#30441=DIRECTION('',(-0.237293631490364,0.,0.971437971490777));
#30442=DIRECTION('',(-0.251657582099965,0.,0.967816336590574));
#30443=DIRECTION('',(-0.265966309141746,0.,0.963982324735012));
#30444=DIRECTION('',(-0.280216672718472,0.,0.959936777257017));
#30445=DIRECTION('',(-0.93556394289254,0.,0.353157342779907));
#30446=DIRECTION('',(-0.954992592290506,0.,0.29662964900741));
#30447=DIRECTION('',(-0.971832145680531,0.,0.235674098326429));
#30448=DIRECTION('',(-0.985571729311693,0.,0.169258283051549));
#30449=DIRECTION('',(-0.995411093351309,0.,0.0956909360031064));
#30450=DIRECTION('',(-0.999929660354767,0.,0.0118606215182996));
#30451=DIRECTION('',(0.912739462772674,0.,0.408542131361566));
#30452=DIRECTION('',(-0.454871137731933,0.,0.890557268264347));
#30453=DIRECTION('center_axis',(0.,-1.,0.));
#30454=DIRECTION('ref_axis',(0.,0.,1.));
#30455=DIRECTION('center_axis',(0.871894798623931,0.,-0.48969323063785));
#30456=DIRECTION('ref_axis',(-0.48969323063785,0.,-0.871894798623931));
#30457=DIRECTION('',(0.,1.,0.));
#30458=DIRECTION('',(-0.451594888615274,-0.386714295024759,-0.80406101173982));
#30459=DIRECTION('',(-0.48969323063785,0.,-0.871894798623931));
#30460=DIRECTION('',(0.,1.,0.));
#30461=DIRECTION('center_axis',(0.817918893329126,0.,-0.575333541465521));
#30462=DIRECTION('ref_axis',(-0.575333541465521,0.,-0.817918893329126));
#30463=DIRECTION('',(0.,1.,0.));
#30464=DIRECTION('',(-0.547096153529848,-0.309436927624307,-0.777775408852244));
#30465=DIRECTION('center_axis',(0.0725221917253267,-0.70710678118655,-0.703377943716856));
#30466=DIRECTION('ref_axis',(-0.99472662747848,0.,-0.102561867110979));
#30467=DIRECTION('',(0.793123151629957,-0.386714295024742,0.470539818051651));
#30468=DIRECTION('',(-0.0363329527197043,-0.706639907076674,0.706639907076678));
#30469=DIRECTION('',(0.99472662747848,0.,0.102561867110979));
#30470=DIRECTION('',(0.945142170174665,-0.176491388068499,0.274876459696312));
#30471=DIRECTION('',(0.862686871695709,-0.309436927624321,0.400025185739962));
#30472=DIRECTION('center_axis',(0.510236429716898,0.,-0.860034177105627));
#30473=DIRECTION('ref_axis',(-0.860034177105627,0.,-0.510236429716898));
#30474=DIRECTION('',(0.,1.,0.));
#30475=DIRECTION('',(-0.793123151629957,-0.386714295024742,-0.470539818051651));
#30476=DIRECTION('',(-0.860034177105627,0.,-0.510236429716898));
#30477=DIRECTION('',(0.,1.,0.));
#30478=DIRECTION('center_axis',(0.420671769125535,0.,-0.907212909222963));
#30479=DIRECTION('ref_axis',(-0.907212909222963,0.,-0.420671769125535));
#30480=DIRECTION('',(0.,1.,0.));
#30481=DIRECTION('',(-0.862686871695709,-0.309436927624321,-0.400025185739962));
#30482=DIRECTION('center_axis',(-0.28888291148617,-0.707106781186549,-0.645404263583122));
#30483=DIRECTION('ref_axis',(-0.912739462772673,0.,0.408542131361568));
#30484=DIRECTION('',(0.922134706666949,-0.386714295024736,0.0109378601098506));
#30485=DIRECTION('',(0.321854693488575,-0.706639907076675,0.630134587216131));
#30486=DIRECTION('',(0.912739462772673,0.,-0.408542131361568));
#30487=DIRECTION('',(0.955955359407371,-0.176491388068498,-0.234521088087999));
#30488=DIRECTION('',(0.94712133926979,-0.309436927624331,-0.0849114628434474));
#30489=DIRECTION('center_axis',(0.0118606215182843,0.,-0.999929660354767));
#30490=DIRECTION('ref_axis',(-0.999929660354767,0.,-0.0118606215182843));
#30491=DIRECTION('',(0.,1.,0.));
#30492=DIRECTION('',(-0.922134706666949,-0.386714295024736,-0.0109378601098506));
#30493=DIRECTION('',(-0.999929660354767,0.,-0.0118606215182843));
#30494=DIRECTION('',(0.,1.,0.));
#30495=DIRECTION('center_axis',(-0.0892940158938145,0.,-0.996005310591041));
#30496=DIRECTION('ref_axis',(-0.996005310591041,0.,0.0892940158938145));
#30497=DIRECTION('',(0.,1.,0.));
#30498=DIRECTION('',(-0.94712133926979,-0.309436927624331,0.0849114628434474));
#30499=DIRECTION('center_axis',(-0.572882071857796,-0.707106781186548,-0.414495032230688));
#30500=DIRECTION('ref_axis',(-0.586184496116912,0.,0.810177595661693));
#30501=DIRECTION('',(0.804061011739819,-0.386714295024756,-0.451594888615276));
#30502=DIRECTION('',(0.593801634496424,-0.706639907076676,0.384785213588103));
#30503=DIRECTION('',(0.586184496116913,0.,-0.810177595661693));
#30504=DIRECTION('',(0.710621082086668,-0.176491388068499,-0.681078899711059));
#30505=DIRECTION('',(0.777775408852244,-0.309436927624306,-0.547096153529848));
#30506=DIRECTION('center_axis',(-0.489693230637852,0.,-0.87189479862393));
#30507=DIRECTION('ref_axis',(-0.87189479862393,0.,0.489693230637852));
#30508=DIRECTION('',(0.,1.,0.));
#30509=DIRECTION('',(-0.804061011739819,-0.386714295024756,0.451594888615276));
#30510=DIRECTION('',(-0.87189479862393,0.,0.489693230637852));
#30511=DIRECTION('',(0.,1.,0.));
#30512=DIRECTION('center_axis',(-0.575333541465521,0.,-0.817918893329126));
#30513=DIRECTION('ref_axis',(-0.817918893329126,0.,0.57533354146552));
#30514=DIRECTION('',(0.,1.,0.));
#30515=DIRECTION('',(-0.777775408852244,-0.309436927624306,0.547096153529848));
#30516=DIRECTION('center_axis',(-0.703377943716856,-0.707106781186549,-0.0725221917253265));
#30517=DIRECTION('ref_axis',(-0.102561867110979,0.,0.99472662747848));
#30518=DIRECTION('',(0.470539818051652,-0.386714295024744,-0.793123151629956));
#30519=DIRECTION('',(0.706639907076678,-0.706639907076675,0.0363329527197041));
#30520=DIRECTION('',(0.102561867110979,0.,-0.99472662747848));
#30521=DIRECTION('',(0.274876459696313,-0.176491388068501,-0.945142170174665));
#30522=DIRECTION('',(0.400025185739966,-0.309436927624327,-0.862686871695706));
#30523=DIRECTION('center_axis',(-0.860034177105626,0.,-0.5102364297169));
#30524=DIRECTION('ref_axis',(-0.5102364297169,0.,0.860034177105626));
#30525=DIRECTION('',(0.,1.,0.));
#30526=DIRECTION('',(-0.470539818051652,-0.386714295024744,0.793123151629956));
#30527=DIRECTION('',(-0.5102364297169,0.,0.860034177105626));
#30528=DIRECTION('',(0.,1.,0.));
#30529=DIRECTION('center_axis',(-0.907212909222961,0.,-0.42067176912554));
#30530=DIRECTION('ref_axis',(-0.42067176912554,0.,0.907212909222961));
#30531=DIRECTION('',(0.,1.,0.));
#30532=DIRECTION('',(-0.400025185739966,-0.309436927624327,0.862686871695706));
#30533=DIRECTION('center_axis',(-0.645404263583122,-0.707106781186549,0.288882911486169));
#30534=DIRECTION('ref_axis',(0.408542131361568,0.,0.912739462772673));
#30535=DIRECTION('',(0.0109378601098593,-0.386714295024742,-0.922134706666946));
#30536=DIRECTION('',(0.630134587216131,-0.706639907076675,-0.321854693488576));
#30537=DIRECTION('',(-0.408542131361568,0.,-0.912739462772673));
#30538=DIRECTION('',(-0.234521088087998,-0.176491388068499,-0.955955359407371));
#30539=DIRECTION('',(-0.0849114628434554,-0.309436927624324,-0.947121339269791));
#30540=DIRECTION('center_axis',(-0.999929660354767,0.,-0.0118606215182939));
#30541=DIRECTION('ref_axis',(-0.0118606215182939,0.,0.999929660354767));
#30542=DIRECTION('',(0.,1.,0.));
#30543=DIRECTION('',(-0.0109378601098593,-0.386714295024742,0.922134706666946));
#30544=DIRECTION('',(-0.0118606215182939,0.,0.999929660354767));
#30545=DIRECTION('',(0.,1.,0.));
#30546=DIRECTION('center_axis',(-0.99600531059104,0.,0.0892940158938226));
#30547=DIRECTION('ref_axis',(0.0892940158938226,0.,0.99600531059104));
#30548=DIRECTION('',(0.,1.,0.));
#30549=DIRECTION('',(0.0849114628434554,-0.309436927624324,0.947121339269791));
#30550=DIRECTION('center_axis',(-0.414495032230688,-0.707106781186549,0.572882071857795));
#30551=DIRECTION('ref_axis',(0.810177595661692,0.,0.586184496116913));
#30552=DIRECTION('',(-0.451594888615301,-0.386714295024736,-0.804061011739815));
#30553=DIRECTION('',(0.384785213588103,-0.706639907076675,-0.593801634496425));
#30554=DIRECTION('',(-0.810177595661692,0.,-0.586184496116913));
#30555=DIRECTION('',(-0.681078899711046,-0.176491388068513,-0.710621082086678));
#30556=DIRECTION('',(-0.547096153529855,-0.309436927624298,-0.777775408852242));
#30557=DIRECTION('center_axis',(-0.871894798623917,0.,0.489693230637875));
#30558=DIRECTION('ref_axis',(0.489693230637875,0.,0.871894798623917));
#30559=DIRECTION('',(0.,1.,0.));
#30560=DIRECTION('',(0.451594888615301,-0.386714295024736,0.804061011739815));
#30561=DIRECTION('',(0.489693230637875,0.,0.871894798623917));
#30562=DIRECTION('',(0.,1.,0.));
#30563=DIRECTION('center_axis',(-0.817918893329121,0.,0.575333541465527));
#30564=DIRECTION('ref_axis',(0.575333541465527,0.,0.817918893329121));
#30565=DIRECTION('',(0.,1.,0.));
#30566=DIRECTION('',(0.547096153529855,-0.309436927624298,0.777775408852242));
#30567=DIRECTION('center_axis',(-0.0725221917253267,-0.70710678118655,0.703377943716856));
#30568=DIRECTION('ref_axis',(0.99472662747848,0.,0.102561867110979));
#30569=DIRECTION('',(-0.793123151629962,-0.386714295024737,-0.470539818051647));
#30570=DIRECTION('',(0.0363329527197052,-0.706639907076674,-0.706639907076678));
#30571=DIRECTION('',(-0.99472662747848,0.,-0.102561867110979));
#30572=DIRECTION('',(-0.945142170174656,-0.17649138806852,-0.274876459696332));
#30573=DIRECTION('',(-0.862686871695723,-0.309436927624304,-0.400025185739946));
#30574=DIRECTION('center_axis',(-0.510236429716893,0.,0.86003417710563));
#30575=DIRECTION('ref_axis',(0.86003417710563,0.,0.510236429716893));
#30576=DIRECTION('',(0.,1.,0.));
#30577=DIRECTION('',(0.793123151629962,-0.386714295024737,0.470539818051647));
#30578=DIRECTION('',(0.86003417710563,0.,0.510236429716893));
#30579=DIRECTION('',(0.,1.,0.));
#30580=DIRECTION('center_axis',(-0.420671769125515,0.,0.907212909222972));
#30581=DIRECTION('ref_axis',(0.907212909222972,0.,0.420671769125515));
#30582=DIRECTION('',(0.,1.,0.));
#30583=DIRECTION('',(0.862686871695723,-0.309436927624304,0.400025185739946));
#30584=DIRECTION('center_axis',(0.28888291148617,-0.707106781186549,0.645404263583122));
#30585=DIRECTION('ref_axis',(0.912739462772673,0.,-0.408542131361568));
#30586=DIRECTION('',(-0.922134706666946,-0.386714295024741,-0.0109378601098575));
#30587=DIRECTION('',(-0.321854693488575,-0.706639907076675,-0.630134587216131));
#30588=DIRECTION('',(-0.912739462772673,0.,0.408542131361568));
#30589=DIRECTION('',(-0.955955359407372,-0.176491388068506,0.23452108808799));
#30590=DIRECTION('',(-0.947121339269795,-0.309436927624305,0.0849114628434785));
#30591=DIRECTION('center_axis',(-0.0118606215182919,0.,0.999929660354767));
#30592=DIRECTION('ref_axis',(0.999929660354767,0.,0.0118606215182919));
#30593=DIRECTION('',(0.,1.,0.));
#30594=DIRECTION('',(0.922134706666946,-0.386714295024741,0.0109378601098575));
#30595=DIRECTION('',(0.999929660354767,0.,0.0118606215182919));
#30596=DIRECTION('',(0.,1.,0.));
#30597=DIRECTION('center_axis',(0.0892940158938463,0.,0.996005310591038));
#30598=DIRECTION('ref_axis',(0.996005310591038,0.,-0.0892940158938463));
#30599=DIRECTION('',(0.,1.,0.));
#30600=DIRECTION('',(0.947121339269795,-0.309436927624305,-0.0849114628434785));
#30601=DIRECTION('center_axis',(0.572882071857795,-0.707106781186549,0.414495032230687));
#30602=DIRECTION('ref_axis',(0.586184496116912,0.,-0.810177595661693));
#30603=DIRECTION('',(-0.804061011739815,-0.386714295024737,0.4515948886153));
#30604=DIRECTION('',(-0.593801634496426,-0.706639907076675,-0.384785213588102));
#30605=DIRECTION('',(-0.586184496116912,0.,0.810177595661693));
#30606=DIRECTION('',(-0.710621082086674,-0.176491388068508,0.681078899711051));
#30607=DIRECTION('',(-0.777775408852245,-0.309436927624309,0.547096153529844));
#30608=DIRECTION('center_axis',(0.489693230637874,0.,0.871894798623917));
#30609=DIRECTION('ref_axis',(0.871894798623918,0.,-0.489693230637874));
#30610=DIRECTION('',(0.,1.,0.));
#30611=DIRECTION('',(0.804061011739815,-0.386714295024737,-0.4515948886153));
#30612=DIRECTION('',(0.871894798623918,0.,-0.489693230637874));
#30613=DIRECTION('',(0.,1.,0.));
#30614=DIRECTION('center_axis',(0.575333541465517,0.,0.817918893329128));
#30615=DIRECTION('ref_axis',(0.817918893329128,0.,-0.575333541465517));
#30616=DIRECTION('',(0.,1.,0.));
#30617=DIRECTION('',(0.777775408852245,-0.309436927624309,-0.547096153529844));
#30618=DIRECTION('center_axis',(0.703377943716856,-0.707106781186549,0.0725221917253273));
#30619=DIRECTION('ref_axis',(0.10256186711098,0.,-0.99472662747848));
#30620=DIRECTION('',(-0.470539818051651,-0.386714295024741,0.793123151629958));
#30621=DIRECTION('',(-0.706639907076678,-0.706639907076675,-0.0363329527197062));
#30622=DIRECTION('',(-0.10256186711098,0.,0.99472662747848));
#30623=DIRECTION('',(-0.27487645969631,-0.176491388068497,0.945142170174666));
#30624=DIRECTION('',(-0.400025185739954,-0.309436927624312,0.862686871695717));
#30625=DIRECTION('center_axis',(0.860034177105628,0.,0.510236429716897));
#30626=DIRECTION('ref_axis',(0.510236429716897,0.,-0.860034177105627));
#30627=DIRECTION('',(0.,1.,0.));
#30628=DIRECTION('',(0.470539818051651,-0.386714295024741,-0.793123151629958));
#30629=DIRECTION('',(0.510236429716897,0.,-0.860034177105627));
#30630=DIRECTION('',(0.,1.,0.));
#30631=DIRECTION('center_axis',(0.907212909222968,0.,0.420671769125525));
#30632=DIRECTION('ref_axis',(0.420671769125525,0.,-0.907212909222968));
#30633=DIRECTION('',(0.,1.,0.));
#30634=DIRECTION('',(0.400025185739954,-0.309436927624312,-0.862686871695717));
#30635=DIRECTION('center_axis',(0.645404263583121,-0.70710678118655,-0.288882911486169));
#30636=DIRECTION('ref_axis',(-0.408542131361568,0.,-0.912739462772673));
#30637=DIRECTION('',(-0.0109378601098576,-0.38671429502474,0.922134706666947));
#30638=DIRECTION('',(-0.630134587216131,-0.706639907076674,0.321854693488576));
#30639=DIRECTION('',(0.408542131361568,0.,0.912739462772673));
#30640=DIRECTION('',(0.234521088088,-0.176491388068496,0.955955359407371));
#30641=DIRECTION('',(0.0849114628434721,-0.30943692762431,0.947121339269795));
#30642=DIRECTION('center_axis',(0.999929660354767,0.,0.011860621518292));
#30643=DIRECTION('ref_axis',(0.011860621518292,0.,-0.999929660354767));
#30644=DIRECTION('',(0.,1.,0.));
#30645=DIRECTION('',(0.0109378601098576,-0.38671429502474,-0.922134706666947));
#30646=DIRECTION('',(0.011860621518292,0.,-0.999929660354767));
#30647=DIRECTION('',(0.,1.,0.));
#30648=DIRECTION('center_axis',(0.996005310591038,0.,-0.0892940158938398));
#30649=DIRECTION('ref_axis',(-0.0892940158938398,0.,-0.996005310591038));
#30650=DIRECTION('',(0.,1.,0.));
#30651=DIRECTION('',(-0.0849114628434721,-0.30943692762431,-0.947121339269795));
#30652=DIRECTION('center_axis',(-0.572882071857796,-0.707106781186548,0.414495032230686));
#30653=DIRECTION('ref_axis',(0.58618449611691,0.,0.810177595661694));
#30654=DIRECTION('',(-0.710621082086669,0.176491388068502,-0.681078899711058));
#30655=DIRECTION('',(-0.58618449611691,0.,-0.810177595661694));
#30656=DIRECTION('',(-0.593801634496424,0.706639907076676,0.384785213588103));
#30657=DIRECTION('',(-0.804061011739819,0.386714295024758,-0.451594888615275));
#30658=DIRECTION('',(-0.777775408852245,0.309436927624312,-0.547096153529842));
#30659=DIRECTION('center_axis',(-0.810177595661694,0.,0.58618449611691));
#30660=DIRECTION('ref_axis',(0.58618449611691,0.,0.810177595661694));
#30661=DIRECTION('',(0.,1.,0.));
#30662=DIRECTION('',(0.58618449611691,0.,0.810177595661694));
#30663=DIRECTION('',(0.,1.,0.));
#30664=DIRECTION('center_axis',(-0.691940859832156,0.,0.721954185869669));
#30665=DIRECTION('ref_axis',(0.721954185869669,0.,0.691940859832156));
#30666=DIRECTION('',(0.,1.,0.));
#30667=DIRECTION('',(0.710621082086669,0.176491388068502,0.681078899711058));
#30668=DIRECTION('center_axis',(-0.288882911486168,-0.707106781186549,0.645404263583123));
#30669=DIRECTION('ref_axis',(0.912739462772674,0.,0.408542131361566));
#30670=DIRECTION('',(-0.955955359407371,0.176491388068495,-0.234521088088));
#30671=DIRECTION('',(-0.912739462772674,0.,-0.408542131361566));
#30672=DIRECTION('',(-0.321854693488574,0.706639907076675,0.630134587216131));
#30673=DIRECTION('',(-0.922134706666944,0.386714295024745,0.0109378601098646));
#30674=DIRECTION('',(-0.947121339269793,0.309436927624317,-0.0849114628434623));
#30675=DIRECTION('center_axis',(-0.408542131361566,0.,0.912739462772674));
#30676=DIRECTION('ref_axis',(0.912739462772674,0.,0.408542131361566));
#30677=DIRECTION('',(0.,1.,0.));
#30678=DIRECTION('',(0.912739462772674,0.,0.408542131361566));
#30679=DIRECTION('',(0.,1.,0.));
#30680=DIRECTION('center_axis',(-0.238261269596264,0.,0.971201095247723));
#30681=DIRECTION('ref_axis',(0.971201095247723,0.,0.238261269596264));
#30682=DIRECTION('',(0.,1.,0.));
#30683=DIRECTION('',(0.955955359407371,0.176491388068495,0.234521088088));
#30684=DIRECTION('center_axis',(0.0725221917253267,-0.70710678118655,0.703377943716856));
#30685=DIRECTION('ref_axis',(0.99472662747848,0.,-0.102561867110979));
#30686=DIRECTION('',(-0.945142170174669,0.176491388068491,0.274876459696304));
#30687=DIRECTION('',(-0.99472662747848,0.,0.102561867110979));
#30688=DIRECTION('',(0.0363329527197052,0.706639907076674,0.706639907076678));
#30689=DIRECTION('',(-0.793123151629957,0.386714295024742,0.470539818051651));
#30690=DIRECTION('',(-0.8626868716957,0.309436927624333,0.400025185739973));
#30691=DIRECTION('center_axis',(0.102561867110979,0.,0.99472662747848));
#30692=DIRECTION('ref_axis',(0.99472662747848,0.,-0.102561867110979));
#30693=DIRECTION('',(0.,1.,0.));
#30694=DIRECTION('',(0.99472662747848,0.,-0.102561867110979));
#30695=DIRECTION('',(0.,1.,0.));
#30696=DIRECTION('center_axis',(0.279260235415558,0.,0.960215455465932));
#30697=DIRECTION('ref_axis',(0.960215455465932,0.,-0.279260235415558));
#30698=DIRECTION('',(0.,1.,0.));
#30699=DIRECTION('',(0.945142170174669,0.176491388068491,-0.274876459696304));
#30700=DIRECTION('center_axis',(0.414495032230686,-0.707106781186548,0.572882071857796));
#30701=DIRECTION('ref_axis',(0.810177595661695,0.,-0.58618449611691));
#30702=DIRECTION('',(-0.681078899711047,0.176491388068514,0.710621082086676));
#30703=DIRECTION('',(-0.810177595661695,0.,0.58618449611691));
#30704=DIRECTION('',(0.384785213588102,0.706639907076676,0.593801634496425));
#30705=DIRECTION('',(-0.451594888615274,0.386714295024759,0.804061011739819));
#30706=DIRECTION('',(-0.547096153529855,0.309436927624302,0.777775408852241));
#30707=DIRECTION('center_axis',(0.58618449611691,0.,0.810177595661695));
#30708=DIRECTION('ref_axis',(0.810177595661695,0.,-0.58618449611691));
#30709=DIRECTION('',(0.,1.,0.));
#30710=DIRECTION('',(0.810177595661695,0.,-0.58618449611691));
#30711=DIRECTION('',(0.,1.,0.));
#30712=DIRECTION('center_axis',(0.721954185869678,0.,0.691940859832147));
#30713=DIRECTION('ref_axis',(0.691940859832147,0.,-0.721954185869678));
#30714=DIRECTION('',(0.,1.,0.));
#30715=DIRECTION('',(0.681078899711047,0.176491388068514,-0.710621082086676));
#30716=DIRECTION('center_axis',(0.64540426358312,-0.707106781186551,0.288882911486168));
#30717=DIRECTION('ref_axis',(0.408542131361567,0.,-0.912739462772673));
#30718=DIRECTION('',(-0.234521088087998,0.176491388068497,0.955955359407371));
#30719=DIRECTION('',(-0.408542131361567,0.,0.912739462772673));
#30720=DIRECTION('',(0.630134587216134,0.706639907076673,0.321854693488573));
#30721=DIRECTION('',(0.0109378601098593,0.38671429502474,0.922134706666947));
#30722=DIRECTION('',(-0.0849114628434554,0.309436927624323,0.947121339269792));
#30723=DIRECTION('center_axis',(0.912739462772673,0.,0.408542131361567));
#30724=DIRECTION('ref_axis',(0.408542131361567,0.,-0.912739462772673));
#30725=DIRECTION('',(0.,1.,0.));
#30726=DIRECTION('',(0.408542131361567,0.,-0.912739462772673));
#30727=DIRECTION('',(0.,1.,0.));
#30728=DIRECTION('center_axis',(0.971201095247723,0.,0.238261269596262));
#30729=DIRECTION('ref_axis',(0.238261269596262,0.,-0.971201095247723));
#30730=DIRECTION('',(0.,1.,0.));
#30731=DIRECTION('',(0.234521088087998,0.176491388068497,-0.955955359407371));
#30732=DIRECTION('center_axis',(0.703377943716856,-0.707106781186549,-0.0725221917253273));
#30733=DIRECTION('ref_axis',(-0.10256186711098,0.,-0.99472662747848));
#30734=DIRECTION('',(0.27487645969631,0.176491388068496,0.945142170174667));
#30735=DIRECTION('',(0.10256186711098,0.,0.99472662747848));
#30736=DIRECTION('',(0.706639907076678,0.706639907076675,-0.0363329527197042));
#30737=DIRECTION('',(0.470539818051652,0.386714295024743,0.793123151629956));
#30738=DIRECTION('',(0.400025185739966,0.309436927624326,0.862686871695706));
#30739=DIRECTION('center_axis',(0.99472662747848,0.,-0.10256186711098));
#30740=DIRECTION('ref_axis',(-0.10256186711098,0.,-0.99472662747848));
#30741=DIRECTION('',(0.,1.,0.));
#30742=DIRECTION('',(-0.10256186711098,0.,-0.99472662747848));
#30743=DIRECTION('',(0.,1.,0.));
#30744=DIRECTION('center_axis',(0.96021545546593,0.,-0.279260235415564));
#30745=DIRECTION('ref_axis',(-0.279260235415564,0.,-0.96021545546593));
#30746=DIRECTION('',(0.,1.,0.));
#30747=DIRECTION('',(-0.27487645969631,0.176491388068496,-0.945142170174667));
#30748=DIRECTION('center_axis',(0.572882071857795,-0.707106781186549,-0.414495032230686));
#30749=DIRECTION('ref_axis',(-0.586184496116911,0.,-0.810177595661694));
#30750=DIRECTION('',(0.710621082086668,0.1764913880685,0.681078899711059));
#30751=DIRECTION('',(0.586184496116911,0.,0.810177595661694));
#30752=DIRECTION('',(0.593801634496425,0.706639907076675,-0.384785213588104));
#30753=DIRECTION('',(0.804061011739822,0.386714295024766,0.451594888615263));
#30754=DIRECTION('',(0.777775408852243,0.309436927624306,0.547096153529849));
#30755=DIRECTION('center_axis',(0.810177595661694,0.,-0.586184496116911));
#30756=DIRECTION('ref_axis',(-0.586184496116911,0.,-0.810177595661694));
#30757=DIRECTION('',(0.,1.,0.));
#30758=DIRECTION('',(-0.586184496116911,0.,-0.810177595661694));
#30759=DIRECTION('',(0.,1.,0.));
#30760=DIRECTION('center_axis',(0.691940859832157,0.,-0.721954185869668));
#30761=DIRECTION('ref_axis',(-0.721954185869668,0.,-0.691940859832157));
#30762=DIRECTION('',(0.,1.,0.));
#30763=DIRECTION('',(-0.710621082086668,0.1764913880685,-0.681078899711059));
#30764=DIRECTION('center_axis',(0.28888291148617,-0.707106781186549,-0.645404263583122));
#30765=DIRECTION('ref_axis',(-0.912739462772673,0.,-0.408542131361568));
#30766=DIRECTION('',(0.955955359407372,0.176491388068506,0.234521088087991));
#30767=DIRECTION('',(0.912739462772673,0.,0.408542131361568));
#30768=DIRECTION('',(0.321854693488575,0.706639907076675,-0.630134587216131));
#30769=DIRECTION('',(0.922134706666946,0.386714295024741,-0.0109378601098576));
#30770=DIRECTION('',(0.947121339269794,0.309436927624312,0.0849114628434706));
#30771=DIRECTION('center_axis',(0.408542131361568,0.,-0.912739462772673));
#30772=DIRECTION('ref_axis',(-0.912739462772673,0.,-0.408542131361568));
#30773=DIRECTION('',(0.,1.,0.));
#30774=DIRECTION('',(-0.912739462772673,0.,-0.408542131361568));
#30775=DIRECTION('',(0.,1.,0.));
#30776=DIRECTION('center_axis',(0.238261269596255,0.,-0.971201095247725));
#30777=DIRECTION('ref_axis',(-0.971201095247725,0.,-0.238261269596255));
#30778=DIRECTION('',(0.,1.,0.));
#30779=DIRECTION('',(-0.955955359407372,0.176491388068506,-0.234521088087991));
#30780=DIRECTION('center_axis',(-0.0725221917253267,-0.70710678118655,-0.703377943716856));
#30781=DIRECTION('ref_axis',(-0.99472662747848,0.,0.102561867110979));
#30782=DIRECTION('',(0.945142170174659,0.176491388068513,-0.274876459696325));
#30783=DIRECTION('',(0.99472662747848,0.,-0.102561867110979));
#30784=DIRECTION('',(-0.0363329527197052,0.706639907076674,-0.706639907076678));
#30785=DIRECTION('',(0.793123151629962,0.386714295024737,-0.470539818051647));
#30786=DIRECTION('',(0.862686871695719,0.30943692762431,-0.400025185739951));
#30787=DIRECTION('center_axis',(-0.102561867110979,0.,-0.99472662747848));
#30788=DIRECTION('ref_axis',(-0.99472662747848,0.,0.102561867110979));
#30789=DIRECTION('',(0.,1.,0.));
#30790=DIRECTION('',(-0.99472662747848,0.,0.102561867110979));
#30791=DIRECTION('',(0.,1.,0.));
#30792=DIRECTION('center_axis',(-0.279260235415581,0.,-0.960215455465925));
#30793=DIRECTION('ref_axis',(-0.960215455465925,0.,0.279260235415581));
#30794=DIRECTION('',(0.,1.,0.));
#30795=DIRECTION('',(-0.945142170174659,0.176491388068513,0.274876459696325));
#30796=DIRECTION('center_axis',(-0.414495032230688,-0.707106781186549,-0.572882071857795));
#30797=DIRECTION('ref_axis',(-0.810177595661692,0.,0.586184496116913));
#30798=DIRECTION('',(0.681078899711057,0.1764913880685,-0.71062108208667));
#30799=DIRECTION('',(0.810177595661692,0.,-0.586184496116913));
#30800=DIRECTION('',(-0.384785213588103,0.706639907076675,-0.593801634496425));
#30801=DIRECTION('',(0.451594888615294,0.386714295024742,-0.804061011739817));
#30802=DIRECTION('',(0.547096153529844,0.309436927624308,-0.777775408852246));
#30803=DIRECTION('center_axis',(-0.586184496116913,0.,-0.810177595661692));
#30804=DIRECTION('ref_axis',(-0.810177595661692,0.,0.586184496116913));
#30805=DIRECTION('',(0.,1.,0.));
#30806=DIRECTION('',(-0.810177595661692,0.,0.586184496116913));
#30807=DIRECTION('',(0.,1.,0.));
#30808=DIRECTION('center_axis',(-0.72195418586967,0.,-0.691940859832155));
#30809=DIRECTION('ref_axis',(-0.691940859832155,0.,0.72195418586967));
#30810=DIRECTION('',(0.,1.,0.));
#30811=DIRECTION('',(-0.681078899711057,0.1764913880685,0.71062108208667));
#30812=DIRECTION('center_axis',(-0.645404263583121,-0.70710678118655,-0.288882911486169));
#30813=DIRECTION('ref_axis',(-0.408542131361568,0.,0.912739462772673));
#30814=DIRECTION('',(0.234521088087999,0.176491388068497,-0.955955359407371));
#30815=DIRECTION('',(0.408542131361568,0.,-0.912739462772673));
#30816=DIRECTION('',(-0.630134587216131,0.706639907076674,-0.321854693488577));
#30817=DIRECTION('',(-0.0109378601098559,0.386714295024739,-0.922134706666947));
#30818=DIRECTION('',(0.0849114628434702,0.309436927624312,-0.947121339269794));
#30819=DIRECTION('center_axis',(-0.912739462772673,0.,-0.408542131361568));
#30820=DIRECTION('ref_axis',(-0.408542131361568,0.,0.912739462772673));
#30821=DIRECTION('',(0.,1.,0.));
#30822=DIRECTION('',(-0.408542131361568,0.,0.912739462772673));
#30823=DIRECTION('',(0.,1.,0.));
#30824=DIRECTION('center_axis',(-0.971201095247723,0.,-0.238261269596264));
#30825=DIRECTION('ref_axis',(-0.238261269596264,0.,0.971201095247723));
#30826=DIRECTION('',(0.,1.,0.));
#30827=DIRECTION('',(-0.234521088087999,0.176491388068497,0.955955359407371));
#30828=DIRECTION('center_axis',(-0.703377943716856,-0.707106781186549,0.0725221917253272));
#30829=DIRECTION('ref_axis',(0.10256186711098,0.,0.99472662747848));
#30830=DIRECTION('',(-0.27487645969631,0.176491388068497,-0.945142170174666));
#30831=DIRECTION('',(-0.10256186711098,0.,-0.99472662747848));
#30832=DIRECTION('',(-0.706639907076678,0.706639907076675,0.0363329527197063));
#30833=DIRECTION('',(-0.47053981805165,0.386714295024741,-0.793123151629958));
#30834=DIRECTION('',(-0.400025185739953,0.309436927624312,-0.862686871695717));
#30835=DIRECTION('center_axis',(-0.99472662747848,0.,0.10256186711098));
#30836=DIRECTION('ref_axis',(0.10256186711098,0.,0.99472662747848));
#30837=DIRECTION('',(0.,1.,0.));
#30838=DIRECTION('',(0.10256186711098,0.,0.99472662747848));
#30839=DIRECTION('',(0.,1.,0.));
#30840=DIRECTION('center_axis',(-0.96021545546593,0.,0.279260235415565));
#30841=DIRECTION('ref_axis',(0.279260235415565,0.,0.96021545546593));
#30842=DIRECTION('',(0.,1.,0.));
#30843=DIRECTION('',(0.27487645969631,0.176491388068497,0.945142170174666));
#30844=DIRECTION('center_axis',(0.645404263583121,0.70710678118655,-0.288882911486169));
#30845=DIRECTION('ref_axis',(-0.408542131361568,0.,-0.912739462772673));
#30846=DIRECTION('',(-0.234521088088,-0.176491388068496,-0.955955359407371));
#30847=DIRECTION('',(-0.408542131361568,0.,-0.912739462772673));
#30848=DIRECTION('',(0.630134587216131,-0.706639907076674,-0.321854693488576));
#30849=DIRECTION('',(0.408542131361568,0.,0.912739462772673));
#30850=DIRECTION('center_axis',(0.,1.,0.));
#30851=DIRECTION('ref_axis',(0.,0.,1.));
#30852=DIRECTION('',(0.890557268264346,0.,-0.454871137731935));
#30853=DIRECTION('',(0.839208594856358,0.,-0.543809648975832));
#30854=DIRECTION('',(-0.58618449611691,0.,-0.810177595661694));
#30855=DIRECTION('',(0.87189479862393,0.,0.489693230637852));
#30856=DIRECTION('',(0.909896762052626,0.,0.414834765185062));
#30857=DIRECTION('',(0.938159296361463,0.,0.346203891732262));
#30858=DIRECTION('',(0.959468375536896,0.,0.28181631667558));
#30859=DIRECTION('',(0.975362669853236,0.,0.220607484589183));
#30860=DIRECTION('',(0.986800812799626,0.,0.161938741065865));
#30861=DIRECTION('',(0.722643145766653,0.,-0.691221298772308));
#30862=DIRECTION('',(0.712324742635051,0.,-0.701850027448819));
#30863=DIRECTION('',(0.701850027448819,0.,-0.712324742635051));
#30864=DIRECTION('',(0.691221298772304,0.,-0.722643145766656));
#30865=DIRECTION('',(-0.161938741065869,0.,-0.986800812799626));
#30866=DIRECTION('',(-0.220607484589178,0.,-0.975362669853237));
#30867=DIRECTION('',(-0.281816316675586,0.,-0.959468375536894));
#30868=DIRECTION('',(-0.346203891732264,0.,-0.938159296361463));
#30869=DIRECTION('',(-0.414834765185058,0.,-0.909896762052629));
#30870=DIRECTION('',(0.810177595661694,0.,0.586184496116911));
#30871=DIRECTION('',(0.54380964897583,0.,-0.839208594856359));
#30872=DIRECTION('',(0.454871137731933,0.,-0.890557268264347));
#30873=DIRECTION('',(-0.912739462772674,0.,-0.408542131361566));
#30874=DIRECTION('',(0.999929660354767,0.,-0.0118606215182996));
#30875=DIRECTION('',(0.995411093351309,0.,-0.0956909360031064));
#30876=DIRECTION('',(0.985571729311693,0.,-0.169258283051549));
#30877=DIRECTION('',(0.971832145680531,0.,-0.235674098326429));
#30878=DIRECTION('',(0.954992592290506,0.,-0.29662964900741));
#30879=DIRECTION('',(0.93556394289254,0.,-0.353157342779907));
#30880=DIRECTION('',(0.280216672718472,0.,-0.959936777257017));
#30881=DIRECTION('',(0.265966309141746,0.,-0.963982324735012));
#30882=DIRECTION('',(0.251657582099965,0.,-0.967816336590574));
#30883=DIRECTION('',(0.237293631490364,0.,-0.971437971490777));
#30884=DIRECTION('',(-0.633643470019728,0.,-0.773625201826672));
#30885=DIRECTION('',(-0.678733020845828,0.,-0.734385107701332));
#30886=DIRECTION('',(-0.723794277210468,0.,-0.690015829004942));
#30887=DIRECTION('',(-0.768901013309911,0.,-0.639367837579427));
#30888=DIRECTION('',(-0.814205826049526,0.,-0.580576328166254));
#30889=DIRECTION('',(0.99472662747848,0.,0.102561867110979));
#30890=DIRECTION('',(0.0513486734079865,0.,-0.998680786707765));
#30891=DIRECTION('',(-0.0513486734079878,0.,-0.998680786707765));
#30892=DIRECTION('',(-0.99472662747848,0.,0.102561867110979));
#30893=DIRECTION('',(0.860034177105627,0.,-0.510236429716898));
#30894=DIRECTION('',(0.814205826049529,0.,-0.580576328166249));
#30895=DIRECTION('',(0.768901013309907,0.,-0.639367837579431));
#30896=DIRECTION('',(0.723794277210464,0.,-0.690015829004945));
#30897=DIRECTION('',(0.678733020845831,0.,-0.734385107701329));
#30898=DIRECTION('',(0.633643470019724,0.,-0.773625201826675));
#30899=DIRECTION('',(-0.237293631490361,0.,-0.971437971490778));
#30900=DIRECTION('',(-0.251657582099955,0.,-0.967816336590577));
#30901=DIRECTION('',(-0.265966309141757,0.,-0.963982324735009));
#30902=DIRECTION('',(-0.280216672718472,0.,-0.959936777257017));
#30903=DIRECTION('',(-0.935563942892542,0.,-0.3531573427799));
#30904=DIRECTION('',(-0.954992592290506,0.,-0.29662964900741));
#30905=DIRECTION('',(-0.971832145680534,0.,-0.235674098326418));
#30906=DIRECTION('',(-0.98557172931169,0.,-0.169258283051569));
#30907=DIRECTION('',(-0.99541109335131,0.,-0.0956909360030991));
#30908=DIRECTION('',(0.912739462772673,0.,-0.408542131361568));
#30909=DIRECTION('',(-0.454871137731933,0.,-0.890557268264347));
#30910=DIRECTION('',(-0.543809648975831,0.,-0.839208594856359));
#30911=DIRECTION('',(-0.810177595661695,0.,0.58618449611691));
#30912=DIRECTION('',(0.48969323063785,0.,-0.871894798623931));
#30913=DIRECTION('',(0.414834765185061,0.,-0.909896762052627));
#30914=DIRECTION('',(0.346203891732263,0.,-0.938159296361463));
#30915=DIRECTION('',(0.281816316675577,0.,-0.959468375536896));
#30916=DIRECTION('',(0.220607484589184,0.,-0.975362669853236));
#30917=DIRECTION('',(0.161938741065862,0.,-0.986800812799627));
#30918=DIRECTION('',(-0.691221298772316,0.,-0.722643145766645));
#30919=DIRECTION('',(-0.701850027448807,0.,-0.712324742635063));
#30920=DIRECTION('',(-0.712324742635063,0.,-0.701850027448807));
#30921=DIRECTION('',(-0.722643145766637,0.,-0.691221298772324));
#30922=DIRECTION('',(-0.986800812799624,0.,0.161938741065875));
#30923=DIRECTION('',(-0.975362669853239,0.,0.220607484589173));
#30924=DIRECTION('',(-0.95946837553689,0.,0.2818163166756));
#30925=DIRECTION('',(-0.938159296361463,0.,0.346203891732262));
#30926=DIRECTION('',(-0.909896762052632,0.,0.41483476518505));
#30927=DIRECTION('',(0.586184496116913,0.,-0.810177595661693));
#30928=DIRECTION('',(-0.839208594856358,0.,-0.543809648975832));
#30929=DIRECTION('',(-0.890557268264349,0.,-0.45487113773193));
#30930=DIRECTION('',(-0.408542131361567,0.,0.912739462772673));
#30931=DIRECTION('',(-0.0118606215182939,0.,-0.999929660354767));
#30932=DIRECTION('',(-0.0956909360031021,0.,-0.99541109335131));
#30933=DIRECTION('',(-0.169258283051555,0.,-0.985571729311692));
#30934=DIRECTION('',(-0.235674098326432,0.,-0.97183214568053));
#30935=DIRECTION('',(-0.296629649007407,0.,-0.954992592290507));
#30936=DIRECTION('',(-0.353157342779899,0.,-0.935563942892543));
#30937=DIRECTION('',(-0.959936777257023,0.,-0.280216672718455));
#30938=DIRECTION('',(-0.963982324735007,0.,-0.265966309141763));
#30939=DIRECTION('',(-0.967816336590582,0.,-0.251657582099936));
#30940=DIRECTION('',(-0.971437971490766,0.,-0.237293631490407));
#30941=DIRECTION('',(-0.77362520182667,0.,0.63364347001973));
#30942=DIRECTION('',(-0.734385107701325,0.,0.678733020845836));
#30943=DIRECTION('',(-0.69001582900495,0.,0.723794277210459));
#30944=DIRECTION('',(-0.639367837579431,0.,0.768901013309908));
#30945=DIRECTION('',(-0.580576328166246,0.,0.814205826049532));
#30946=DIRECTION('',(0.102561867110979,0.,-0.99472662747848));
#30947=DIRECTION('',(-0.998680786707765,0.,-0.0513486734079863));
#30948=DIRECTION('',(-0.998680786707765,0.,0.0513486734079864));
#30949=DIRECTION('',(0.10256186711098,0.,0.99472662747848));
#30950=DIRECTION('',(-0.510236429716899,0.,-0.860034177105626));
#30951=DIRECTION('',(-0.580576328166246,0.,-0.814205826049531));
#30952=DIRECTION('',(-0.639367837579431,0.,-0.768901013309907));
#30953=DIRECTION('',(-0.69001582900495,0.,-0.723794277210459));
#30954=DIRECTION('',(-0.734385107701325,0.,-0.678733020845836));
#30955=DIRECTION('',(-0.773625201826676,0.,-0.633643470019722));
#30956=DIRECTION('',(-0.971437971490773,0.,0.237293631490379));
#30957=DIRECTION('',(-0.967816336590582,0.,0.251657582099936));
#30958=DIRECTION('',(-0.963982324735007,0.,0.265966309141761));
#30959=DIRECTION('',(-0.959936777257014,0.,0.280216672718486));
#30960=DIRECTION('',(-0.3531573427799,0.,0.935563942892542));
#30961=DIRECTION('',(-0.296629649007409,0.,0.954992592290506));
#30962=DIRECTION('',(-0.235674098326432,0.,0.97183214568053));
#30963=DIRECTION('',(-0.169258283051555,0.,0.985571729311692));
#30964=DIRECTION('',(-0.0956909360031021,0.,0.99541109335131));
#30965=DIRECTION('',(-0.408542131361568,0.,-0.912739462772673));
#30966=DIRECTION('',(-0.890557268264346,0.,0.454871137731935));
#30967=DIRECTION('',(-0.839208594856358,0.,0.543809648975832));
#30968=DIRECTION('',(0.586184496116911,0.,0.810177595661694));
#30969=DIRECTION('',(-0.871894798623937,0.,-0.48969323063784));
#30970=DIRECTION('',(-0.909896762052627,0.,-0.414834765185061));
#30971=DIRECTION('',(-0.938159296361463,0.,-0.346203891732263));
#30972=DIRECTION('',(-0.959468375536898,0.,-0.281816316675571));
#30973=DIRECTION('',(-0.975362669853233,0.,-0.2206074845892));
#30974=DIRECTION('',(-0.986800812799626,0.,-0.161938741065863));
#30975=DIRECTION('',(-0.722643145766668,0.,0.691221298772292));
#30976=DIRECTION('',(-0.71232474263504,0.,0.701850027448831));
#30977=DIRECTION('',(-0.701850027448823,0.,0.712324742635048));
#30978=DIRECTION('',(-0.691221298772293,0.,0.722643145766667));
#30979=DIRECTION('',(0.161938741065865,0.,0.986800812799626));
#30980=DIRECTION('',(0.22060748458919,0.,0.975362669853235));
#30981=DIRECTION('',(0.281816316675564,0.,0.9594683755369));
#30982=DIRECTION('',(0.346203891732269,0.,0.938159296361461));
#30983=DIRECTION('',(0.414834765185046,0.,0.909896762052634));
#30984=DIRECTION('',(-0.810177595661692,0.,-0.586184496116913));
#30985=DIRECTION('',(-0.543809648975832,0.,0.839208594856358));
#30986=DIRECTION('',(-0.454871137731933,0.,0.890557268264347));
#30987=DIRECTION('',(0.912739462772673,0.,0.408542131361568));
#30988=DIRECTION('',(-0.999929660354767,0.,0.011860621518292));
#30989=DIRECTION('',(-0.99541109335131,0.,0.0956909360031057));
#30990=DIRECTION('',(-0.985571729311695,0.,0.169258283051542));
#30991=DIRECTION('',(-0.971832145680524,0.,0.235674098326456));
#30992=DIRECTION('',(-0.95499259229051,0.,0.296629649007398));
#30993=DIRECTION('',(-0.935563942892542,0.,0.3531573427799));
#30994=DIRECTION('',(-0.280216672718478,0.,0.959936777257016));
#30995=DIRECTION('',(-0.265966309141754,0.,0.963982324735009));
#30996=DIRECTION('',(-0.251657582099958,0.,0.967816336590576));
#30997=DIRECTION('',(-0.237293631490357,0.,0.971437971490779));
#30998=DIRECTION('',(0.63364347001972,0.,0.773625201826678));
#30999=DIRECTION('',(0.678733020845838,0.,0.734385107701322));
#31000=DIRECTION('',(0.723794277210454,0.,0.690015829004956));
#31001=DIRECTION('',(0.768901013309911,0.,0.639367837579427));
#31002=DIRECTION('',(0.814205826049522,0.,0.580576328166259));
#31003=DIRECTION('',(-0.99472662747848,0.,-0.102561867110979));
#31004=DIRECTION('',(-0.0513486734079878,0.,0.998680786707765));
#31005=DIRECTION('',(0.0513486734079878,0.,0.998680786707765));
#31006=DIRECTION('',(0.99472662747848,0.,-0.102561867110979));
#31007=DIRECTION('',(-0.86003417710563,0.,0.510236429716893));
#31008=DIRECTION('',(-0.814205826049519,0.,0.580576328166263));
#31009=DIRECTION('',(-0.768901013309918,0.,0.639367837579419));
#31010=DIRECTION('',(-0.723794277210445,0.,0.690015829004965));
#31011=DIRECTION('',(-0.678733020845843,0.,0.734385107701318));
#31012=DIRECTION('',(-0.633643470019724,0.,0.773625201826675));
#31013=DIRECTION('',(0.237293631490368,0.,0.971437971490776));
#31014=DIRECTION('',(0.251657582099958,0.,0.967816336590576));
#31015=DIRECTION('',(0.265966309141754,0.,0.963982324735009));
#31016=DIRECTION('',(0.280216672718464,0.,0.95993677725702));
#31017=DIRECTION('',(0.93556394289254,0.,0.353157342779906));
#31018=DIRECTION('',(0.954992592290512,0.,0.296629649007392));
#31019=DIRECTION('',(0.971832145680526,0.,0.235674098326448));
#31020=DIRECTION('',(0.985571729311693,0.,0.169258283051549));
#31021=DIRECTION('',(0.995411093351309,0.,0.0956909360031137));
#31022=DIRECTION('',(-0.912739462772673,0.,0.408542131361568));
#31023=DIRECTION('',(0.454871137731934,0.,0.890557268264347));
#31024=DIRECTION('',(0.543809648975831,0.,0.839208594856358));
#31025=DIRECTION('',(0.810177595661692,0.,-0.586184496116913));
#31026=DIRECTION('',(-0.489693230637868,0.,0.871894798623921));
#31027=DIRECTION('',(-0.414834765185049,0.,0.909896762052633));
#31028=DIRECTION('',(-0.346203891732272,0.,0.93815929636146));
#31029=DIRECTION('',(-0.281816316675565,0.,0.9594683755369));
#31030=DIRECTION('',(-0.220607484589187,0.,0.975362669853235));
#31031=DIRECTION('',(-0.161938741065865,0.,0.986800812799626));
#31032=DIRECTION('',(0.691221298772312,0.,0.722643145766649));
#31033=DIRECTION('',(0.701850027448815,0.,0.712324742635055));
#31034=DIRECTION('',(0.712324742635051,0.,0.701850027448819));
#31035=DIRECTION('',(0.722643145766652,0.,0.691221298772308));
#31036=DIRECTION('',(0.986800812799626,0.,-0.161938741065868));
#31037=DIRECTION('',(0.975362669853236,0.,-0.220607484589184));
#31038=DIRECTION('',(0.9594683755369,0.,-0.281816316675565));
#31039=DIRECTION('',(0.938159296361459,0.,-0.346203891732275));
#31040=DIRECTION('',(0.909896762052635,0.,-0.414834765185043));
#31041=DIRECTION('',(-0.586184496116912,0.,0.810177595661693));
#31042=DIRECTION('',(0.839208594856359,0.,0.54380964897583));
#31043=DIRECTION('',(0.890557268264346,0.,0.454871137731935));
#31044=DIRECTION('',(0.408542131361568,0.,-0.912739462772673));
#31045=DIRECTION('',(0.0118606215182901,0.,0.999929660354767));
#31046=DIRECTION('',(0.0956909360031101,0.,0.995411093351309));
#31047=DIRECTION('',(0.169258283051554,0.,0.985571729311692));
#31048=DIRECTION('',(0.235674098326447,0.,0.971832145680527));
#31049=DIRECTION('',(0.296629649007399,0.,0.954992592290509));
#31050=DIRECTION('',(0.353157342779898,0.,0.935563942892543));
#31051=DIRECTION('',(0.959936777257018,0.,0.28021667271847));
#31052=DIRECTION('',(0.963982324735007,0.,0.265966309141762));
#31053=DIRECTION('',(0.967816336590576,0.,0.251657582099957));
#31054=DIRECTION('',(0.971437971490777,0.,0.237293631490364));
#31055=DIRECTION('',(0.773625201826672,0.,-0.633643470019727));
#31056=DIRECTION('',(0.734385107701324,0.,-0.678733020845836));
#31057=DIRECTION('',(0.690015829004958,0.,-0.723794277210452));
#31058=DIRECTION('',(0.639367837579427,0.,-0.768901013309911));
#31059=DIRECTION('',(0.580576328166257,0.,-0.814205826049523));
#31060=DIRECTION('',(-0.10256186711098,0.,0.99472662747848));
#31061=DIRECTION('',(0.998680786707765,0.,0.0513486734079893));
#31062=DIRECTION('',(0.998680786707765,0.,-0.0513486734079894));
#31063=DIRECTION('',(-0.10256186711098,0.,-0.99472662747848));
#31064=DIRECTION('',(0.510236429716897,0.,0.860034177105627));
#31065=DIRECTION('',(0.580576328166257,0.,0.814205826049523));
#31066=DIRECTION('',(0.639367837579427,0.,0.768901013309911));
#31067=DIRECTION('',(0.690015829004958,0.,0.723794277210452));
#31068=DIRECTION('',(0.734385107701324,0.,0.678733020845837));
#31069=DIRECTION('',(0.773625201826672,0.,0.633643470019727));
#31070=DIRECTION('',(0.971437971490777,0.,-0.237293631490364));
#31071=DIRECTION('',(0.967816336590576,0.,-0.251657582099957));
#31072=DIRECTION('',(0.963982324735009,0.,-0.265966309141754));
#31073=DIRECTION('',(0.959936777257016,0.,-0.280216672718478));
#31074=DIRECTION('',(0.353157342779898,0.,-0.935563942892543));
#31075=DIRECTION('',(0.296629649007403,0.,-0.954992592290508));
#31076=DIRECTION('',(0.235674098326445,0.,-0.971832145680527));
#31077=DIRECTION('',(0.169258283051556,0.,-0.985571729311692));
#31078=DIRECTION('',(0.0956909360031075,0.,-0.995411093351309));
#31079=DIRECTION('center_axis',(0.,1.,0.));
#31080=DIRECTION('ref_axis',(0.,0.,1.));
#31081=DIRECTION('center_axis',(-0.703377943716856,0.707106781186549,0.0725221917253272));
#31082=DIRECTION('ref_axis',(0.10256186711098,0.,0.99472662747848));
#31083=DIRECTION('',(0.47053981805165,0.386714295024741,0.793123151629958));
#31084=DIRECTION('',(0.706639907076678,0.706639907076675,-0.0363329527197063));
#31085=DIRECTION('',(0.400025185739953,0.309436927624312,0.862686871695717));
#31086=DIRECTION('center_axis',(0.703377943716856,0.707106781186549,0.0725221917253273));
#31087=DIRECTION('ref_axis',(0.10256186711098,0.,-0.99472662747848));
#31088=DIRECTION('',(0.27487645969631,-0.176491388068497,-0.945142170174666));
#31089=DIRECTION('',(0.10256186711098,0.,-0.99472662747848));
#31090=DIRECTION('',(0.706639907076678,-0.706639907076675,0.0363329527197062));
#31091=DIRECTION('center_axis',(-0.645404263583121,0.70710678118655,-0.288882911486169));
#31092=DIRECTION('ref_axis',(-0.408542131361568,0.,0.912739462772673));
#31093=DIRECTION('',(0.0109378601098559,0.386714295024739,0.922134706666947));
#31094=DIRECTION('',(0.630134587216131,0.706639907076674,0.321854693488577));
#31095=DIRECTION('',(-0.0849114628434702,0.309436927624312,0.947121339269794));
#31096=DIRECTION('center_axis',(0.572882071857795,0.707106781186549,0.414495032230687));
#31097=DIRECTION('ref_axis',(0.586184496116912,0.,-0.810177595661693));
#31098=DIRECTION('',(0.710621082086674,-0.176491388068508,-0.681078899711051));
#31099=DIRECTION('',(0.586184496116912,0.,-0.810177595661693));
#31100=DIRECTION('',(0.593801634496426,-0.706639907076675,0.384785213588102));
#31101=DIRECTION('center_axis',(-0.414495032230688,0.707106781186549,-0.572882071857795));
#31102=DIRECTION('ref_axis',(-0.810177595661692,0.,0.586184496116913));
#31103=DIRECTION('',(-0.451594888615294,0.386714295024742,0.804061011739817));
#31104=DIRECTION('',(0.384785213588103,0.706639907076675,0.593801634496425));
#31105=DIRECTION('',(-0.547096153529844,0.309436927624308,0.777775408852246));
#31106=DIRECTION('center_axis',(0.28888291148617,0.707106781186549,0.645404263583122));
#31107=DIRECTION('ref_axis',(0.912739462772673,0.,-0.408542131361568));
#31108=DIRECTION('',(0.955955359407372,-0.176491388068506,-0.23452108808799));
#31109=DIRECTION('',(0.912739462772673,0.,-0.408542131361568));
#31110=DIRECTION('',(0.321854693488575,-0.706639907076675,0.630134587216131));
#31111=DIRECTION('center_axis',(-0.0725221917253267,0.70710678118655,-0.703377943716856));
#31112=DIRECTION('ref_axis',(-0.99472662747848,0.,0.102561867110979));
#31113=DIRECTION('',(-0.793123151629962,0.386714295024737,0.470539818051647));
#31114=DIRECTION('',(0.0363329527197052,0.706639907076674,0.706639907076678));
#31115=DIRECTION('',(-0.862686871695719,0.30943692762431,0.400025185739951));
#31116=DIRECTION('center_axis',(-0.0725221917253267,0.70710678118655,0.703377943716856));
#31117=DIRECTION('ref_axis',(0.99472662747848,0.,0.102561867110979));
#31118=DIRECTION('',(0.945142170174656,-0.17649138806852,0.274876459696332));
#31119=DIRECTION('',(0.99472662747848,0.,0.102561867110979));
#31120=DIRECTION('',(-0.0363329527197052,-0.706639907076674,0.706639907076678));
#31121=DIRECTION('center_axis',(0.28888291148617,0.707106781186549,-0.645404263583122));
#31122=DIRECTION('ref_axis',(-0.912739462772673,0.,-0.408542131361568));
#31123=DIRECTION('',(-0.922134706666946,0.386714295024741,0.0109378601098576));
#31124=DIRECTION('',(-0.321854693488575,0.706639907076675,0.630134587216131));
#31125=DIRECTION('',(-0.947121339269794,0.309436927624312,-0.0849114628434706));
#31126=DIRECTION('center_axis',(-0.414495032230688,0.707106781186549,0.572882071857795));
#31127=DIRECTION('ref_axis',(0.810177595661692,0.,0.586184496116913));
#31128=DIRECTION('',(0.681078899711046,-0.176491388068513,0.710621082086678));
#31129=DIRECTION('',(0.810177595661692,0.,0.586184496116913));
#31130=DIRECTION('',(-0.384785213588103,-0.706639907076675,0.593801634496425));
#31131=DIRECTION('center_axis',(0.572882071857795,0.707106781186549,-0.414495032230686));
#31132=DIRECTION('ref_axis',(-0.586184496116911,0.,-0.810177595661694));
#31133=DIRECTION('',(-0.804061011739822,0.386714295024766,-0.451594888615263));
#31134=DIRECTION('',(-0.593801634496425,0.706639907076675,0.384785213588104));
#31135=DIRECTION('',(-0.777775408852243,0.309436927624306,-0.547096153529849));
#31136=DIRECTION('center_axis',(-0.645404263583122,0.707106781186549,0.288882911486169));
#31137=DIRECTION('ref_axis',(0.408542131361568,0.,0.912739462772673));
#31138=DIRECTION('',(0.234521088087998,-0.176491388068499,0.955955359407371));
#31139=DIRECTION('',(0.408542131361568,0.,0.912739462772673));
#31140=DIRECTION('',(-0.630134587216131,-0.706639907076675,0.321854693488576));
#31141=DIRECTION('center_axis',(0.703377943716856,0.707106781186549,-0.0725221917253273));
#31142=DIRECTION('ref_axis',(-0.10256186711098,0.,-0.99472662747848));
#31143=DIRECTION('',(-0.470539818051652,0.386714295024743,-0.793123151629956));
#31144=DIRECTION('',(-0.706639907076678,0.706639907076675,0.0363329527197042));
#31145=DIRECTION('',(-0.400025185739966,0.309436927624326,-0.862686871695706));
#31146=DIRECTION('center_axis',(-0.703377943716856,0.707106781186549,-0.0725221917253265));
#31147=DIRECTION('ref_axis',(-0.102561867110979,0.,0.99472662747848));
#31148=DIRECTION('',(-0.274876459696313,-0.176491388068501,0.945142170174665));
#31149=DIRECTION('',(-0.102561867110979,0.,0.99472662747848));
#31150=DIRECTION('',(-0.706639907076678,-0.706639907076675,-0.0363329527197041));
#31151=DIRECTION('center_axis',(0.64540426358312,0.707106781186551,0.288882911486168));
#31152=DIRECTION('ref_axis',(0.408542131361567,0.,-0.912739462772673));
#31153=DIRECTION('',(-0.0109378601098593,0.38671429502474,-0.922134706666947));
#31154=DIRECTION('',(-0.630134587216134,0.706639907076673,-0.321854693488573));
#31155=DIRECTION('',(0.0849114628434554,0.309436927624323,-0.947121339269792));
#31156=DIRECTION('center_axis',(-0.572882071857796,0.707106781186548,-0.414495032230688));
#31157=DIRECTION('ref_axis',(-0.586184496116912,0.,0.810177595661693));
#31158=DIRECTION('',(-0.710621082086668,-0.176491388068499,0.681078899711059));
#31159=DIRECTION('',(-0.586184496116913,0.,0.810177595661693));
#31160=DIRECTION('',(-0.593801634496424,-0.706639907076676,-0.384785213588103));
#31161=DIRECTION('center_axis',(0.414495032230686,0.707106781186548,0.572882071857796));
#31162=DIRECTION('ref_axis',(0.810177595661695,0.,-0.58618449611691));
#31163=DIRECTION('',(0.451594888615274,0.386714295024759,-0.804061011739819));
#31164=DIRECTION('',(-0.384785213588102,0.706639907076676,-0.593801634496425));
#31165=DIRECTION('',(0.547096153529855,0.309436927624302,-0.777775408852241));
#31166=DIRECTION('center_axis',(-0.28888291148617,0.707106781186549,-0.645404263583122));
#31167=DIRECTION('ref_axis',(-0.912739462772673,0.,0.408542131361568));
#31168=DIRECTION('',(-0.955955359407371,-0.176491388068498,0.234521088087999));
#31169=DIRECTION('',(-0.912739462772673,0.,0.408542131361568));
#31170=DIRECTION('',(-0.321854693488575,-0.706639907076675,-0.630134587216131));
#31171=DIRECTION('center_axis',(0.0725221917253267,0.70710678118655,0.703377943716856));
#31172=DIRECTION('ref_axis',(0.99472662747848,0.,-0.102561867110979));
#31173=DIRECTION('',(0.793123151629957,0.386714295024742,-0.470539818051651));
#31174=DIRECTION('',(-0.0363329527197052,0.706639907076674,-0.706639907076678));
#31175=DIRECTION('',(0.8626868716957,0.309436927624333,-0.400025185739973));
#31176=DIRECTION('center_axis',(0.0725221917253267,0.70710678118655,-0.703377943716856));
#31177=DIRECTION('ref_axis',(-0.99472662747848,0.,-0.102561867110979));
#31178=DIRECTION('',(-0.945142170174665,-0.176491388068499,-0.274876459696312));
#31179=DIRECTION('',(-0.99472662747848,0.,-0.102561867110979));
#31180=DIRECTION('',(0.0363329527197043,-0.706639907076674,-0.706639907076678));
#31181=DIRECTION('center_axis',(-0.288882911486168,0.707106781186549,0.645404263583123));
#31182=DIRECTION('ref_axis',(0.912739462772674,0.,0.408542131361566));
#31183=DIRECTION('',(0.922134706666944,0.386714295024745,-0.0109378601098646));
#31184=DIRECTION('',(0.321854693488574,0.706639907076675,-0.630134587216131));
#31185=DIRECTION('',(0.947121339269793,0.309436927624317,0.0849114628434623));
#31186=DIRECTION('center_axis',(0.414495032230687,0.707106781186548,-0.572882071857796));
#31187=DIRECTION('ref_axis',(-0.810177595661694,0.,-0.586184496116911));
#31188=DIRECTION('',(-0.681078899711059,-0.1764913880685,-0.710621082086668));
#31189=DIRECTION('',(-0.810177595661694,0.,-0.586184496116911));
#31190=DIRECTION('',(0.384785213588102,-0.706639907076676,-0.593801634496425));
#31191=DIRECTION('center_axis',(-0.572882071857796,0.707106781186548,0.414495032230686));
#31192=DIRECTION('ref_axis',(0.58618449611691,0.,0.810177595661694));
#31193=DIRECTION('',(0.804061011739819,0.386714295024758,0.451594888615275));
#31194=DIRECTION('',(0.593801634496424,0.706639907076676,-0.384785213588103));
#31195=DIRECTION('',(0.777775408852245,0.309436927624312,0.547096153529842));
#31196=DIRECTION('center_axis',(0.454871137731935,0.,0.890557268264346));
#31197=DIRECTION('ref_axis',(0.890557268264346,0.,-0.454871137731935));
#31198=DIRECTION('',(0.,1.,0.));
#31199=DIRECTION('',(0.,1.,0.));
#31200=DIRECTION('center_axis',(0.912739462772673,0.,-0.408542131361568));
#31201=DIRECTION('ref_axis',(-0.408542131361568,0.,-0.912739462772673));
#31202=DIRECTION('',(0.,1.,0.));
#31203=DIRECTION('center_axis',(0.971201095247723,0.,-0.238261269596264));
#31204=DIRECTION('ref_axis',(-0.238261269596264,0.,-0.971201095247723));
#31205=DIRECTION('center_axis',(0.995411093351309,0.,0.0956909360031075));
#31206=DIRECTION('ref_axis',(0.0956909360031075,0.,-0.995411093351309));
#31207=DIRECTION('',(0.,1.,0.));
#31208=DIRECTION('center_axis',(0.985571729311692,0.,0.169258283051556));
#31209=DIRECTION('ref_axis',(0.169258283051556,0.,-0.985571729311692));
#31210=DIRECTION('',(0.,1.,0.));
#31211=DIRECTION('center_axis',(0.971832145680527,0.,0.235674098326445));
#31212=DIRECTION('ref_axis',(0.235674098326445,0.,-0.971832145680527));
#31213=DIRECTION('',(0.,1.,0.));
#31214=DIRECTION('center_axis',(0.954992592290508,0.,0.296629649007403));
#31215=DIRECTION('ref_axis',(0.296629649007403,0.,-0.954992592290508));
#31216=DIRECTION('',(0.,1.,0.));
#31217=DIRECTION('center_axis',(0.935563942892543,0.,0.353157342779898));
#31218=DIRECTION('ref_axis',(0.353157342779898,0.,-0.935563942892543));
#31219=DIRECTION('',(0.,1.,0.));
#31220=DIRECTION('center_axis',(0.280216672718478,0.,0.959936777257016));
#31221=DIRECTION('ref_axis',(0.959936777257016,0.,-0.280216672718478));
#31222=DIRECTION('',(0.,1.,0.));
#31223=DIRECTION('center_axis',(0.265966309141754,0.,0.963982324735009));
#31224=DIRECTION('ref_axis',(0.963982324735009,0.,-0.265966309141754));
#31225=DIRECTION('',(0.,1.,0.));
#31226=DIRECTION('center_axis',(0.251657582099958,0.,0.967816336590576));
#31227=DIRECTION('ref_axis',(0.967816336590576,0.,-0.251657582099958));
#31228=DIRECTION('',(0.,1.,0.));
#31229=DIRECTION('center_axis',(0.237293631490364,0.,0.971437971490777));
#31230=DIRECTION('ref_axis',(0.971437971490777,0.,-0.237293631490364));
#31231=DIRECTION('',(0.,1.,0.));
#31232=DIRECTION('center_axis',(-0.633643470019727,0.,0.773625201826672));
#31233=DIRECTION('ref_axis',(0.773625201826672,0.,0.633643470019727));
#31234=DIRECTION('',(0.,1.,0.));
#31235=DIRECTION('center_axis',(-0.678733020845837,0.,0.734385107701324));
#31236=DIRECTION('ref_axis',(0.734385107701324,0.,0.678733020845837));
#31237=DIRECTION('',(0.,1.,0.));
#31238=DIRECTION('center_axis',(-0.723794277210452,0.,0.690015829004958));
#31239=DIRECTION('ref_axis',(0.690015829004958,0.,0.723794277210452));
#31240=DIRECTION('',(0.,1.,0.));
#31241=DIRECTION('center_axis',(-0.768901013309911,0.,0.639367837579427));
#31242=DIRECTION('ref_axis',(0.639367837579427,0.,0.768901013309911));
#31243=DIRECTION('',(0.,1.,0.));
#31244=DIRECTION('center_axis',(-0.814205826049523,0.,0.580576328166257));
#31245=DIRECTION('ref_axis',(0.580576328166257,0.,0.814205826049523));
#31246=DIRECTION('',(0.,1.,0.));
#31247=DIRECTION('center_axis',(-0.860034177105628,0.,0.510236429716897));
#31248=DIRECTION('ref_axis',(0.510236429716897,0.,0.860034177105627));
#31249=DIRECTION('',(0.,1.,0.));
#31250=DIRECTION('center_axis',(-0.907212909222968,0.,0.420671769125524));
#31251=DIRECTION('ref_axis',(0.420671769125524,0.,0.907212909222968));
#31252=DIRECTION('center_axis',(0.0513486734079894,0.,0.998680786707765));
#31253=DIRECTION('ref_axis',(0.998680786707765,0.,-0.0513486734079894));
#31254=DIRECTION('',(0.,1.,0.));
#31255=DIRECTION('center_axis',(-0.0513486734079893,0.,0.998680786707765));
#31256=DIRECTION('ref_axis',(0.998680786707765,0.,0.0513486734079893));
#31257=DIRECTION('',(0.,1.,0.));
#31258=DIRECTION('center_axis',(0.99472662747848,0.,0.10256186711098));
#31259=DIRECTION('ref_axis',(0.10256186711098,0.,-0.99472662747848));
#31260=DIRECTION('',(0.,1.,0.));
#31261=DIRECTION('center_axis',(0.96021545546593,0.,0.279260235415565));
#31262=DIRECTION('ref_axis',(0.279260235415565,0.,-0.96021545546593));
#31263=DIRECTION('center_axis',(0.814205826049523,0.,0.580576328166257));
#31264=DIRECTION('ref_axis',(0.580576328166257,0.,-0.814205826049523));
#31265=DIRECTION('',(0.,1.,0.));
#31266=DIRECTION('center_axis',(0.768901013309911,0.,0.639367837579427));
#31267=DIRECTION('ref_axis',(0.639367837579427,0.,-0.768901013309911));
#31268=DIRECTION('',(0.,1.,0.));
#31269=DIRECTION('center_axis',(0.723794277210452,0.,0.690015829004958));
#31270=DIRECTION('ref_axis',(0.690015829004958,0.,-0.723794277210452));
#31271=DIRECTION('',(0.,1.,0.));
#31272=DIRECTION('center_axis',(0.678733020845836,0.,0.734385107701324));
#31273=DIRECTION('ref_axis',(0.734385107701324,0.,-0.678733020845836));
#31274=DIRECTION('',(0.,1.,0.));
#31275=DIRECTION('center_axis',(0.633643470019727,0.,0.773625201826672));
#31276=DIRECTION('ref_axis',(0.773625201826672,0.,-0.633643470019727));
#31277=DIRECTION('',(0.,1.,0.));
#31278=DIRECTION('center_axis',(-0.237293631490364,0.,0.971437971490777));
#31279=DIRECTION('ref_axis',(0.971437971490777,0.,0.237293631490364));
#31280=DIRECTION('',(0.,1.,0.));
#31281=DIRECTION('center_axis',(-0.251657582099957,0.,0.967816336590576));
#31282=DIRECTION('ref_axis',(0.967816336590576,0.,0.251657582099957));
#31283=DIRECTION('',(0.,1.,0.));
#31284=DIRECTION('center_axis',(-0.265966309141762,0.,0.963982324735007));
#31285=DIRECTION('ref_axis',(0.963982324735007,0.,0.265966309141762));
#31286=DIRECTION('',(0.,1.,0.));
#31287=DIRECTION('center_axis',(-0.28021667271847,0.,0.959936777257018));
#31288=DIRECTION('ref_axis',(0.959936777257018,0.,0.28021667271847));
#31289=DIRECTION('',(0.,1.,0.));
#31290=DIRECTION('center_axis',(-0.935563942892543,0.,0.353157342779898));
#31291=DIRECTION('ref_axis',(0.353157342779898,0.,0.935563942892543));
#31292=DIRECTION('',(0.,1.,0.));
#31293=DIRECTION('center_axis',(-0.954992592290509,0.,0.296629649007399));
#31294=DIRECTION('ref_axis',(0.296629649007399,0.,0.954992592290509));
#31295=DIRECTION('',(0.,1.,0.));
#31296=DIRECTION('center_axis',(-0.971832145680527,0.,0.235674098326447));
#31297=DIRECTION('ref_axis',(0.235674098326447,0.,0.971832145680527));
#31298=DIRECTION('',(0.,1.,0.));
#31299=DIRECTION('center_axis',(-0.985571729311692,0.,0.169258283051554));
#31300=DIRECTION('ref_axis',(0.169258283051554,0.,0.985571729311692));
#31301=DIRECTION('',(0.,1.,0.));
#31302=DIRECTION('center_axis',(-0.995411093351309,0.,0.0956909360031101));
#31303=DIRECTION('ref_axis',(0.0956909360031101,0.,0.995411093351309));
#31304=DIRECTION('',(0.,1.,0.));
#31305=DIRECTION('center_axis',(-0.999929660354767,0.,0.0118606215182901));
#31306=DIRECTION('ref_axis',(0.0118606215182901,0.,0.999929660354767));
#31307=DIRECTION('',(0.,1.,0.));
#31308=DIRECTION('center_axis',(-0.996005310591038,0.,-0.0892940158938378));
#31309=DIRECTION('ref_axis',(-0.0892940158938378,0.,0.996005310591038));
#31310=DIRECTION('center_axis',(-0.454871137731935,0.,0.890557268264346));
#31311=DIRECTION('ref_axis',(0.890557268264346,0.,0.454871137731935));
#31312=DIRECTION('',(0.,1.,0.));
#31313=DIRECTION('center_axis',(-0.54380964897583,0.,0.839208594856359));
#31314=DIRECTION('ref_axis',(0.839208594856359,0.,0.54380964897583));
#31315=DIRECTION('',(0.,1.,0.));
#31316=DIRECTION('center_axis',(0.810177595661693,0.,0.586184496116912));
#31317=DIRECTION('ref_axis',(0.586184496116912,0.,-0.810177595661693));
#31318=DIRECTION('',(0.,1.,0.));
#31319=DIRECTION('center_axis',(0.69194085983215,0.,0.721954185869675));
#31320=DIRECTION('ref_axis',(0.721954185869675,0.,-0.69194085983215));
#31321=DIRECTION('center_axis',(0.414834765185043,0.,0.909896762052635));
#31322=DIRECTION('ref_axis',(0.909896762052635,0.,-0.414834765185043));
#31323=DIRECTION('',(0.,1.,0.));
#31324=DIRECTION('center_axis',(0.346203891732275,0.,0.938159296361459));
#31325=DIRECTION('ref_axis',(0.938159296361459,0.,-0.346203891732275));
#31326=DIRECTION('',(0.,1.,0.));
#31327=DIRECTION('center_axis',(0.281816316675565,0.,0.9594683755369));
#31328=DIRECTION('ref_axis',(0.9594683755369,0.,-0.281816316675565));
#31329=DIRECTION('',(0.,1.,0.));
#31330=DIRECTION('center_axis',(0.220607484589184,0.,0.975362669853236));
#31331=DIRECTION('ref_axis',(0.975362669853236,0.,-0.220607484589184));
#31332=DIRECTION('',(0.,1.,0.));
#31333=DIRECTION('center_axis',(0.161938741065868,0.,0.986800812799626));
#31334=DIRECTION('ref_axis',(0.986800812799626,0.,-0.161938741065868));
#31335=DIRECTION('',(0.,1.,0.));
#31336=DIRECTION('center_axis',(-0.691221298772308,0.,0.722643145766652));
#31337=DIRECTION('ref_axis',(0.722643145766652,0.,0.691221298772308));
#31338=DIRECTION('',(0.,1.,0.));
#31339=DIRECTION('center_axis',(-0.701850027448819,0.,0.712324742635051));
#31340=DIRECTION('ref_axis',(0.712324742635051,0.,0.701850027448819));
#31341=DIRECTION('',(0.,1.,0.));
#31342=DIRECTION('center_axis',(-0.712324742635055,0.,0.701850027448815));
#31343=DIRECTION('ref_axis',(0.701850027448815,0.,0.712324742635055));
#31344=DIRECTION('',(0.,1.,0.));
#31345=DIRECTION('center_axis',(-0.722643145766649,0.,0.691221298772312));
#31346=DIRECTION('ref_axis',(0.691221298772312,0.,0.722643145766649));
#31347=DIRECTION('',(0.,1.,0.));
#31348=DIRECTION('center_axis',(-0.986800812799626,0.,-0.161938741065865));
#31349=DIRECTION('ref_axis',(-0.161938741065865,0.,0.986800812799626));
#31350=DIRECTION('',(0.,1.,0.));
#31351=DIRECTION('center_axis',(-0.975362669853235,0.,-0.220607484589187));
#31352=DIRECTION('ref_axis',(-0.220607484589187,0.,0.975362669853235));
#31353=DIRECTION('',(0.,1.,0.));
#31354=DIRECTION('center_axis',(-0.9594683755369,0.,-0.281816316675565));
#31355=DIRECTION('ref_axis',(-0.281816316675565,0.,0.9594683755369));
#31356=DIRECTION('',(0.,1.,0.));
#31357=DIRECTION('center_axis',(-0.93815929636146,0.,-0.346203891732272));
#31358=DIRECTION('ref_axis',(-0.346203891732272,0.,0.93815929636146));
#31359=DIRECTION('',(0.,1.,0.));
#31360=DIRECTION('center_axis',(-0.909896762052633,0.,-0.414834765185049));
#31361=DIRECTION('ref_axis',(-0.414834765185049,0.,0.909896762052633));
#31362=DIRECTION('',(0.,1.,0.));
#31363=DIRECTION('center_axis',(-0.871894798623921,0.,-0.489693230637868));
#31364=DIRECTION('ref_axis',(-0.489693230637868,0.,0.871894798623921));
#31365=DIRECTION('',(0.,1.,0.));
#31366=DIRECTION('center_axis',(-0.817918893329128,0.,-0.575333541465517));
#31367=DIRECTION('ref_axis',(-0.575333541465517,0.,0.817918893329128));
#31368=DIRECTION('center_axis',(-0.839208594856358,0.,0.543809648975831));
#31369=DIRECTION('ref_axis',(0.543809648975831,0.,0.839208594856358));
#31370=DIRECTION('',(0.,1.,0.));
#31371=DIRECTION('center_axis',(-0.890557268264347,0.,0.454871137731934));
#31372=DIRECTION('ref_axis',(0.454871137731934,0.,0.890557268264347));
#31373=DIRECTION('',(0.,1.,0.));
#31374=DIRECTION('center_axis',(0.408542131361568,0.,0.912739462772673));
#31375=DIRECTION('ref_axis',(0.912739462772673,0.,-0.408542131361568));
#31376=DIRECTION('',(0.,1.,0.));
#31377=DIRECTION('center_axis',(0.238261269596254,0.,0.971201095247725));
#31378=DIRECTION('ref_axis',(0.971201095247725,0.,-0.238261269596254));
#31379=DIRECTION('center_axis',(-0.0956909360031137,0.,0.995411093351309));
#31380=DIRECTION('ref_axis',(0.995411093351309,0.,0.0956909360031137));
#31381=DIRECTION('',(0.,1.,0.));
#31382=DIRECTION('center_axis',(-0.169258283051549,0.,0.985571729311693));
#31383=DIRECTION('ref_axis',(0.985571729311693,0.,0.169258283051549));
#31384=DIRECTION('',(0.,1.,0.));
#31385=DIRECTION('center_axis',(-0.235674098326448,0.,0.971832145680526));
#31386=DIRECTION('ref_axis',(0.971832145680526,0.,0.235674098326448));
#31387=DIRECTION('',(0.,1.,0.));
#31388=DIRECTION('center_axis',(-0.296629649007392,0.,0.954992592290512));
#31389=DIRECTION('ref_axis',(0.954992592290512,0.,0.296629649007392));
#31390=DIRECTION('',(0.,1.,0.));
#31391=DIRECTION('center_axis',(-0.353157342779906,0.,0.93556394289254));
#31392=DIRECTION('ref_axis',(0.93556394289254,0.,0.353157342779906));
#31393=DIRECTION('',(0.,1.,0.));
#31394=DIRECTION('center_axis',(-0.95993677725702,0.,0.280216672718464));
#31395=DIRECTION('ref_axis',(0.280216672718464,0.,0.95993677725702));
#31396=DIRECTION('',(0.,1.,0.));
#31397=DIRECTION('center_axis',(-0.963982324735009,0.,0.265966309141754));
#31398=DIRECTION('ref_axis',(0.265966309141754,0.,0.963982324735009));
#31399=DIRECTION('',(0.,1.,0.));
#31400=DIRECTION('center_axis',(-0.967816336590576,0.,0.251657582099958));
#31401=DIRECTION('ref_axis',(0.251657582099958,0.,0.967816336590576));
#31402=DIRECTION('',(0.,1.,0.));
#31403=DIRECTION('center_axis',(-0.971437971490776,0.,0.237293631490368));
#31404=DIRECTION('ref_axis',(0.237293631490368,0.,0.971437971490776));
#31405=DIRECTION('',(0.,1.,0.));
#31406=DIRECTION('center_axis',(-0.773625201826675,0.,-0.633643470019724));
#31407=DIRECTION('ref_axis',(-0.633643470019724,0.,0.773625201826675));
#31408=DIRECTION('',(0.,1.,0.));
#31409=DIRECTION('center_axis',(-0.734385107701318,0.,-0.678733020845843));
#31410=DIRECTION('ref_axis',(-0.678733020845843,0.,0.734385107701318));
#31411=DIRECTION('',(0.,1.,0.));
#31412=DIRECTION('center_axis',(-0.690015829004965,0.,-0.723794277210445));
#31413=DIRECTION('ref_axis',(-0.723794277210445,0.,0.690015829004965));
#31414=DIRECTION('',(0.,1.,0.));
#31415=DIRECTION('center_axis',(-0.639367837579419,0.,-0.768901013309918));
#31416=DIRECTION('ref_axis',(-0.768901013309918,0.,0.639367837579419));
#31417=DIRECTION('',(0.,1.,0.));
#31418=DIRECTION('center_axis',(-0.580576328166263,0.,-0.814205826049519));
#31419=DIRECTION('ref_axis',(-0.814205826049519,0.,0.580576328166263));
#31420=DIRECTION('',(0.,1.,0.));
#31421=DIRECTION('center_axis',(-0.510236429716893,0.,-0.86003417710563));
#31422=DIRECTION('ref_axis',(-0.86003417710563,0.,0.510236429716893));
#31423=DIRECTION('',(0.,1.,0.));
#31424=DIRECTION('center_axis',(-0.420671769125522,0.,-0.907212909222969));
#31425=DIRECTION('ref_axis',(-0.907212909222969,0.,0.420671769125522));
#31426=DIRECTION('center_axis',(-0.998680786707765,0.,0.0513486734079878));
#31427=DIRECTION('ref_axis',(0.0513486734079878,0.,0.998680786707765));
#31428=DIRECTION('',(0.,1.,0.));
#31429=DIRECTION('center_axis',(-0.998680786707765,0.,-0.0513486734079878));
#31430=DIRECTION('ref_axis',(-0.0513486734079878,0.,0.998680786707765));
#31431=DIRECTION('',(0.,1.,0.));
#31432=DIRECTION('center_axis',(-0.102561867110979,0.,0.99472662747848));
#31433=DIRECTION('ref_axis',(0.99472662747848,0.,0.102561867110979));
#31434=DIRECTION('',(0.,1.,0.));
#31435=DIRECTION('center_axis',(-0.279260235415588,0.,0.960215455465923));
#31436=DIRECTION('ref_axis',(0.960215455465923,0.,0.279260235415588));
#31437=DIRECTION('center_axis',(-0.580576328166259,0.,0.814205826049522));
#31438=DIRECTION('ref_axis',(0.814205826049522,0.,0.580576328166259));
#31439=DIRECTION('',(0.,1.,0.));
#31440=DIRECTION('center_axis',(-0.639367837579427,0.,0.768901013309911));
#31441=DIRECTION('ref_axis',(0.768901013309911,0.,0.639367837579427));
#31442=DIRECTION('',(0.,1.,0.));
#31443=DIRECTION('center_axis',(-0.690015829004956,0.,0.723794277210454));
#31444=DIRECTION('ref_axis',(0.723794277210454,0.,0.690015829004956));
#31445=DIRECTION('',(0.,1.,0.));
#31446=DIRECTION('center_axis',(-0.734385107701322,0.,0.678733020845838));
#31447=DIRECTION('ref_axis',(0.678733020845838,0.,0.734385107701322));
#31448=DIRECTION('',(0.,1.,0.));
#31449=DIRECTION('center_axis',(-0.773625201826678,0.,0.63364347001972));
#31450=DIRECTION('ref_axis',(0.63364347001972,0.,0.773625201826678));
#31451=DIRECTION('',(0.,1.,0.));
#31452=DIRECTION('center_axis',(-0.971437971490779,0.,-0.237293631490357));
#31453=DIRECTION('ref_axis',(-0.237293631490357,0.,0.971437971490779));
#31454=DIRECTION('',(0.,1.,0.));
#31455=DIRECTION('center_axis',(-0.967816336590576,0.,-0.251657582099958));
#31456=DIRECTION('ref_axis',(-0.251657582099958,0.,0.967816336590576));
#31457=DIRECTION('',(0.,1.,0.));
#31458=DIRECTION('center_axis',(-0.963982324735009,0.,-0.265966309141754));
#31459=DIRECTION('ref_axis',(-0.265966309141754,0.,0.963982324735009));
#31460=DIRECTION('',(0.,1.,0.));
#31461=DIRECTION('center_axis',(-0.959936777257016,0.,-0.280216672718478));
#31462=DIRECTION('ref_axis',(-0.280216672718478,0.,0.959936777257016));
#31463=DIRECTION('',(0.,1.,0.));
#31464=DIRECTION('center_axis',(-0.3531573427799,0.,-0.935563942892542));
#31465=DIRECTION('ref_axis',(-0.935563942892542,0.,0.3531573427799));
#31466=DIRECTION('',(0.,1.,0.));
#31467=DIRECTION('center_axis',(-0.296629649007398,0.,-0.95499259229051));
#31468=DIRECTION('ref_axis',(-0.95499259229051,0.,0.296629649007398));
#31469=DIRECTION('',(0.,1.,0.));
#31470=DIRECTION('center_axis',(-0.235674098326456,0.,-0.971832145680524));
#31471=DIRECTION('ref_axis',(-0.971832145680524,0.,0.235674098326456));
#31472=DIRECTION('',(0.,1.,0.));
#31473=DIRECTION('center_axis',(-0.169258283051542,0.,-0.985571729311695));
#31474=DIRECTION('ref_axis',(-0.985571729311695,0.,0.169258283051542));
#31475=DIRECTION('',(0.,1.,0.));
#31476=DIRECTION('center_axis',(-0.0956909360031057,0.,-0.99541109335131));
#31477=DIRECTION('ref_axis',(-0.99541109335131,0.,0.0956909360031057));
#31478=DIRECTION('',(0.,1.,0.));
#31479=DIRECTION('center_axis',(-0.011860621518292,0.,-0.999929660354767));
#31480=DIRECTION('ref_axis',(-0.999929660354767,0.,0.011860621518292));
#31481=DIRECTION('',(0.,1.,0.));
#31482=DIRECTION('center_axis',(0.0892940158938382,0.,-0.996005310591038));
#31483=DIRECTION('ref_axis',(-0.996005310591038,0.,-0.0892940158938382));
#31484=DIRECTION('center_axis',(-0.890557268264347,0.,-0.454871137731934));
#31485=DIRECTION('ref_axis',(-0.454871137731934,0.,0.890557268264347));
#31486=DIRECTION('',(0.,1.,0.));
#31487=DIRECTION('center_axis',(-0.839208594856358,0.,-0.543809648975832));
#31488=DIRECTION('ref_axis',(-0.543809648975832,0.,0.839208594856358));
#31489=DIRECTION('',(0.,1.,0.));
#31490=DIRECTION('center_axis',(-0.586184496116913,0.,0.810177595661692));
#31491=DIRECTION('ref_axis',(0.810177595661692,0.,0.586184496116913));
#31492=DIRECTION('',(0.,1.,0.));
#31493=DIRECTION('center_axis',(-0.72195418586968,0.,0.691940859832145));
#31494=DIRECTION('ref_axis',(0.691940859832145,0.,0.72195418586968));
#31495=DIRECTION('center_axis',(-0.909896762052634,0.,0.414834765185046));
#31496=DIRECTION('ref_axis',(0.414834765185046,0.,0.909896762052634));
#31497=DIRECTION('',(0.,1.,0.));
#31498=DIRECTION('center_axis',(-0.938159296361461,0.,0.346203891732269));
#31499=DIRECTION('ref_axis',(0.346203891732269,0.,0.938159296361461));
#31500=DIRECTION('',(0.,1.,0.));
#31501=DIRECTION('center_axis',(-0.9594683755369,0.,0.281816316675564));
#31502=DIRECTION('ref_axis',(0.281816316675564,0.,0.9594683755369));
#31503=DIRECTION('',(0.,1.,0.));
#31504=DIRECTION('center_axis',(-0.975362669853235,0.,0.22060748458919));
#31505=DIRECTION('ref_axis',(0.22060748458919,0.,0.975362669853235));
#31506=DIRECTION('',(0.,1.,0.));
#31507=DIRECTION('center_axis',(-0.986800812799626,0.,0.161938741065865));
#31508=DIRECTION('ref_axis',(0.161938741065865,0.,0.986800812799626));
#31509=DIRECTION('',(0.,1.,0.));
#31510=DIRECTION('center_axis',(-0.722643145766667,0.,-0.691221298772293));
#31511=DIRECTION('ref_axis',(-0.691221298772293,0.,0.722643145766667));
#31512=DIRECTION('',(0.,1.,0.));
#31513=DIRECTION('center_axis',(-0.712324742635048,0.,-0.701850027448823));
#31514=DIRECTION('ref_axis',(-0.701850027448823,0.,0.712324742635048));
#31515=DIRECTION('',(0.,1.,0.));
#31516=DIRECTION('center_axis',(-0.701850027448831,0.,-0.71232474263504));
#31517=DIRECTION('ref_axis',(-0.71232474263504,0.,0.701850027448831));
#31518=DIRECTION('',(0.,1.,0.));
#31519=DIRECTION('center_axis',(-0.691221298772292,0.,-0.722643145766668));
#31520=DIRECTION('ref_axis',(-0.722643145766668,0.,0.691221298772292));
#31521=DIRECTION('',(0.,1.,0.));
#31522=DIRECTION('center_axis',(0.161938741065863,0.,-0.986800812799627));
#31523=DIRECTION('ref_axis',(-0.986800812799626,0.,-0.161938741065863));
#31524=DIRECTION('',(0.,1.,0.));
#31525=DIRECTION('center_axis',(0.2206074845892,0.,-0.975362669853233));
#31526=DIRECTION('ref_axis',(-0.975362669853233,0.,-0.2206074845892));
#31527=DIRECTION('',(0.,1.,0.));
#31528=DIRECTION('center_axis',(0.281816316675571,0.,-0.959468375536898));
#31529=DIRECTION('ref_axis',(-0.959468375536898,0.,-0.281816316675571));
#31530=DIRECTION('',(0.,1.,0.));
#31531=DIRECTION('center_axis',(0.346203891732263,0.,-0.938159296361463));
#31532=DIRECTION('ref_axis',(-0.938159296361463,0.,-0.346203891732263));
#31533=DIRECTION('',(0.,1.,0.));
#31534=DIRECTION('center_axis',(0.414834765185061,0.,-0.909896762052627));
#31535=DIRECTION('ref_axis',(-0.909896762052627,0.,-0.414834765185061));
#31536=DIRECTION('',(0.,1.,0.));
#31537=DIRECTION('center_axis',(0.48969323063784,0.,-0.871894798623937));
#31538=DIRECTION('ref_axis',(-0.871894798623937,0.,-0.48969323063784));
#31539=DIRECTION('',(0.,1.,0.));
#31540=DIRECTION('center_axis',(0.575333541465521,0.,-0.817918893329125));
#31541=DIRECTION('ref_axis',(-0.817918893329125,0.,-0.575333541465521));
#31542=DIRECTION('center_axis',(-0.543809648975832,0.,-0.839208594856358));
#31543=DIRECTION('ref_axis',(-0.839208594856358,0.,0.543809648975832));
#31544=DIRECTION('',(0.,1.,0.));
#31545=DIRECTION('center_axis',(-0.454871137731935,0.,-0.890557268264346));
#31546=DIRECTION('ref_axis',(-0.890557268264346,0.,0.454871137731935));
#31547=DIRECTION('',(0.,1.,0.));
#31548=DIRECTION('center_axis',(-0.912739462772673,0.,0.408542131361568));
#31549=DIRECTION('ref_axis',(0.408542131361568,0.,0.912739462772673));
#31550=DIRECTION('',(0.,1.,0.));
#31551=DIRECTION('center_axis',(-0.971201095247723,0.,0.238261269596262));
#31552=DIRECTION('ref_axis',(0.238261269596262,0.,0.971201095247723));
#31553=DIRECTION('center_axis',(-0.99541109335131,0.,-0.0956909360031021));
#31554=DIRECTION('ref_axis',(-0.0956909360031021,0.,0.99541109335131));
#31555=DIRECTION('',(0.,1.,0.));
#31556=DIRECTION('center_axis',(-0.985571729311692,0.,-0.169258283051555));
#31557=DIRECTION('ref_axis',(-0.169258283051555,0.,0.985571729311692));
#31558=DIRECTION('',(0.,1.,0.));
#31559=DIRECTION('center_axis',(-0.97183214568053,0.,-0.235674098326432));
#31560=DIRECTION('ref_axis',(-0.235674098326432,0.,0.97183214568053));
#31561=DIRECTION('',(0.,1.,0.));
#31562=DIRECTION('center_axis',(-0.954992592290506,0.,-0.296629649007409));
#31563=DIRECTION('ref_axis',(-0.296629649007409,0.,0.954992592290506));
#31564=DIRECTION('',(0.,1.,0.));
#31565=DIRECTION('center_axis',(-0.935563942892542,0.,-0.3531573427799));
#31566=DIRECTION('ref_axis',(-0.3531573427799,0.,0.935563942892542));
#31567=DIRECTION('',(0.,1.,0.));
#31568=DIRECTION('center_axis',(-0.280216672718486,0.,-0.959936777257014));
#31569=DIRECTION('ref_axis',(-0.959936777257014,0.,0.280216672718486));
#31570=DIRECTION('',(0.,1.,0.));
#31571=DIRECTION('center_axis',(-0.265966309141761,0.,-0.963982324735007));
#31572=DIRECTION('ref_axis',(-0.963982324735007,0.,0.265966309141761));
#31573=DIRECTION('',(0.,1.,0.));
#31574=DIRECTION('center_axis',(-0.251657582099936,0.,-0.967816336590582));
#31575=DIRECTION('ref_axis',(-0.967816336590582,0.,0.251657582099936));
#31576=DIRECTION('',(0.,1.,0.));
#31577=DIRECTION('center_axis',(-0.237293631490379,0.,-0.971437971490773));
#31578=DIRECTION('ref_axis',(-0.971437971490773,0.,0.237293631490379));
#31579=DIRECTION('',(0.,1.,0.));
#31580=DIRECTION('center_axis',(0.633643470019722,0.,-0.773625201826676));
#31581=DIRECTION('ref_axis',(-0.773625201826676,0.,-0.633643470019722));
#31582=DIRECTION('',(0.,1.,0.));
#31583=DIRECTION('center_axis',(0.678733020845836,0.,-0.734385107701325));
#31584=DIRECTION('ref_axis',(-0.734385107701325,0.,-0.678733020845836));
#31585=DIRECTION('',(0.,1.,0.));
#31586=DIRECTION('center_axis',(0.723794277210459,0.,-0.69001582900495));
#31587=DIRECTION('ref_axis',(-0.69001582900495,0.,-0.723794277210459));
#31588=DIRECTION('',(0.,1.,0.));
#31589=DIRECTION('center_axis',(0.768901013309907,0.,-0.639367837579431));
#31590=DIRECTION('ref_axis',(-0.639367837579431,0.,-0.768901013309907));
#31591=DIRECTION('',(0.,1.,0.));
#31592=DIRECTION('center_axis',(0.814205826049531,0.,-0.580576328166246));
#31593=DIRECTION('ref_axis',(-0.580576328166246,0.,-0.814205826049531));
#31594=DIRECTION('',(0.,1.,0.));
#31595=DIRECTION('center_axis',(0.860034177105626,0.,-0.510236429716899));
#31596=DIRECTION('ref_axis',(-0.510236429716899,0.,-0.860034177105626));
#31597=DIRECTION('',(0.,1.,0.));
#31598=DIRECTION('center_axis',(0.907212909222961,0.,-0.42067176912554));
#31599=DIRECTION('ref_axis',(-0.42067176912554,0.,-0.907212909222961));
#31600=DIRECTION('center_axis',(-0.0513486734079864,0.,-0.998680786707765));
#31601=DIRECTION('ref_axis',(-0.998680786707765,0.,0.0513486734079864));
#31602=DIRECTION('',(0.,1.,0.));
#31603=DIRECTION('center_axis',(0.0513486734079863,0.,-0.998680786707765));
#31604=DIRECTION('ref_axis',(-0.998680786707765,0.,-0.0513486734079863));
#31605=DIRECTION('',(0.,1.,0.));
#31606=DIRECTION('center_axis',(-0.99472662747848,0.,-0.102561867110979));
#31607=DIRECTION('ref_axis',(-0.102561867110979,0.,0.99472662747848));
#31608=DIRECTION('',(0.,1.,0.));
#31609=DIRECTION('center_axis',(-0.960215455465929,0.,-0.279260235415567));
#31610=DIRECTION('ref_axis',(-0.279260235415567,0.,0.960215455465929));
#31611=DIRECTION('center_axis',(-0.814205826049532,0.,-0.580576328166246));
#31612=DIRECTION('ref_axis',(-0.580576328166246,0.,0.814205826049532));
#31613=DIRECTION('',(0.,1.,0.));
#31614=DIRECTION('center_axis',(-0.768901013309908,0.,-0.639367837579431));
#31615=DIRECTION('ref_axis',(-0.639367837579431,0.,0.768901013309908));
#31616=DIRECTION('',(0.,1.,0.));
#31617=DIRECTION('center_axis',(-0.723794277210459,0.,-0.69001582900495));
#31618=DIRECTION('ref_axis',(-0.69001582900495,0.,0.723794277210459));
#31619=DIRECTION('',(0.,1.,0.));
#31620=DIRECTION('center_axis',(-0.678733020845836,0.,-0.734385107701325));
#31621=DIRECTION('ref_axis',(-0.734385107701325,0.,0.678733020845836));
#31622=DIRECTION('',(0.,1.,0.));
#31623=DIRECTION('center_axis',(-0.63364347001973,0.,-0.77362520182667));
#31624=DIRECTION('ref_axis',(-0.77362520182667,0.,0.63364347001973));
#31625=DIRECTION('',(0.,1.,0.));
#31626=DIRECTION('center_axis',(0.237293631490407,0.,-0.971437971490766));
#31627=DIRECTION('ref_axis',(-0.971437971490766,0.,-0.237293631490407));
#31628=DIRECTION('',(0.,1.,0.));
#31629=DIRECTION('center_axis',(0.251657582099936,0.,-0.967816336590582));
#31630=DIRECTION('ref_axis',(-0.967816336590582,0.,-0.251657582099936));
#31631=DIRECTION('',(0.,1.,0.));
#31632=DIRECTION('center_axis',(0.265966309141763,0.,-0.963982324735007));
#31633=DIRECTION('ref_axis',(-0.963982324735007,0.,-0.265966309141763));
#31634=DIRECTION('',(0.,1.,0.));
#31635=DIRECTION('center_axis',(0.280216672718455,0.,-0.959936777257023));
#31636=DIRECTION('ref_axis',(-0.959936777257023,0.,-0.280216672718455));
#31637=DIRECTION('',(0.,1.,0.));
#31638=DIRECTION('center_axis',(0.935563942892543,0.,-0.353157342779899));
#31639=DIRECTION('ref_axis',(-0.353157342779899,0.,-0.935563942892543));
#31640=DIRECTION('',(0.,1.,0.));
#31641=DIRECTION('center_axis',(0.954992592290507,0.,-0.296629649007407));
#31642=DIRECTION('ref_axis',(-0.296629649007407,0.,-0.954992592290507));
#31643=DIRECTION('',(0.,1.,0.));
#31644=DIRECTION('center_axis',(0.97183214568053,0.,-0.235674098326432));
#31645=DIRECTION('ref_axis',(-0.235674098326432,0.,-0.97183214568053));
#31646=DIRECTION('',(0.,1.,0.));
#31647=DIRECTION('center_axis',(0.985571729311692,0.,-0.169258283051555));
#31648=DIRECTION('ref_axis',(-0.169258283051555,0.,-0.985571729311692));
#31649=DIRECTION('',(0.,1.,0.));
#31650=DIRECTION('center_axis',(0.99541109335131,0.,-0.0956909360031021));
#31651=DIRECTION('ref_axis',(-0.0956909360031021,0.,-0.99541109335131));
#31652=DIRECTION('',(0.,1.,0.));
#31653=DIRECTION('center_axis',(0.999929660354767,0.,-0.0118606215182939));
#31654=DIRECTION('ref_axis',(-0.0118606215182939,0.,-0.999929660354767));
#31655=DIRECTION('',(0.,1.,0.));
#31656=DIRECTION('center_axis',(0.99600531059104,0.,0.0892940158938226));
#31657=DIRECTION('ref_axis',(0.0892940158938226,0.,-0.99600531059104));
#31658=DIRECTION('center_axis',(0.45487113773193,0.,-0.890557268264349));
#31659=DIRECTION('ref_axis',(-0.890557268264349,0.,-0.45487113773193));
#31660=DIRECTION('',(0.,1.,0.));
#31661=DIRECTION('center_axis',(0.543809648975832,0.,-0.839208594856358));
#31662=DIRECTION('ref_axis',(-0.839208594856358,0.,-0.543809648975832));
#31663=DIRECTION('',(0.,1.,0.));
#31664=DIRECTION('center_axis',(-0.810177595661693,0.,-0.586184496116913));
#31665=DIRECTION('ref_axis',(-0.586184496116913,0.,0.810177595661693));
#31666=DIRECTION('',(0.,1.,0.));
#31667=DIRECTION('center_axis',(-0.691940859832157,0.,-0.721954185869668));
#31668=DIRECTION('ref_axis',(-0.721954185869668,0.,0.691940859832157));
#31669=DIRECTION('center_axis',(-0.41483476518505,0.,-0.909896762052632));
#31670=DIRECTION('ref_axis',(-0.909896762052632,0.,0.41483476518505));
#31671=DIRECTION('',(0.,1.,0.));
#31672=DIRECTION('center_axis',(-0.346203891732262,0.,-0.938159296361464));
#31673=DIRECTION('ref_axis',(-0.938159296361463,0.,0.346203891732262));
#31674=DIRECTION('',(0.,1.,0.));
#31675=DIRECTION('center_axis',(-0.2818163166756,0.,-0.95946837553689));
#31676=DIRECTION('ref_axis',(-0.95946837553689,0.,0.2818163166756));
#31677=DIRECTION('',(0.,1.,0.));
#31678=DIRECTION('center_axis',(-0.220607484589173,0.,-0.975362669853239));
#31679=DIRECTION('ref_axis',(-0.975362669853239,0.,0.220607484589173));
#31680=DIRECTION('',(0.,1.,0.));
#31681=DIRECTION('center_axis',(-0.161938741065875,0.,-0.986800812799625));
#31682=DIRECTION('ref_axis',(-0.986800812799624,0.,0.161938741065875));
#31683=DIRECTION('',(0.,1.,0.));
#31684=DIRECTION('center_axis',(0.691221298772324,0.,-0.722643145766637));
#31685=DIRECTION('ref_axis',(-0.722643145766637,0.,-0.691221298772324));
#31686=DIRECTION('',(0.,1.,0.));
#31687=DIRECTION('center_axis',(0.701850027448807,0.,-0.712324742635063));
#31688=DIRECTION('ref_axis',(-0.712324742635063,0.,-0.701850027448807));
#31689=DIRECTION('',(0.,1.,0.));
#31690=DIRECTION('center_axis',(0.712324742635063,0.,-0.701850027448807));
#31691=DIRECTION('ref_axis',(-0.701850027448807,0.,-0.712324742635063));
#31692=DIRECTION('',(0.,1.,0.));
#31693=DIRECTION('center_axis',(0.722643145766645,0.,-0.691221298772316));
#31694=DIRECTION('ref_axis',(-0.691221298772316,0.,-0.722643145766645));
#31695=DIRECTION('',(0.,1.,0.));
#31696=DIRECTION('center_axis',(0.986800812799627,0.,0.161938741065862));
#31697=DIRECTION('ref_axis',(0.161938741065862,0.,-0.986800812799627));
#31698=DIRECTION('',(0.,1.,0.));
#31699=DIRECTION('center_axis',(0.975362669853236,0.,0.220607484589184));
#31700=DIRECTION('ref_axis',(0.220607484589184,0.,-0.975362669853236));
#31701=DIRECTION('',(0.,1.,0.));
#31702=DIRECTION('center_axis',(0.959468375536897,0.,0.281816316675577));
#31703=DIRECTION('ref_axis',(0.281816316675577,0.,-0.959468375536896));
#31704=DIRECTION('',(0.,1.,0.));
#31705=DIRECTION('center_axis',(0.938159296361463,0.,0.346203891732263));
#31706=DIRECTION('ref_axis',(0.346203891732263,0.,-0.938159296361463));
#31707=DIRECTION('',(0.,1.,0.));
#31708=DIRECTION('center_axis',(0.909896762052627,0.,0.414834765185061));
#31709=DIRECTION('ref_axis',(0.414834765185061,0.,-0.909896762052627));
#31710=DIRECTION('',(0.,1.,0.));
#31711=DIRECTION('center_axis',(0.871894798623931,0.,0.48969323063785));
#31712=DIRECTION('ref_axis',(0.48969323063785,0.,-0.871894798623931));
#31713=DIRECTION('',(0.,1.,0.));
#31714=DIRECTION('center_axis',(0.817918893329121,0.,0.575333541465527));
#31715=DIRECTION('ref_axis',(0.575333541465527,0.,-0.817918893329121));
#31716=DIRECTION('center_axis',(0.839208594856359,0.,-0.543809648975831));
#31717=DIRECTION('ref_axis',(-0.543809648975831,0.,-0.839208594856359));
#31718=DIRECTION('',(0.,1.,0.));
#31719=DIRECTION('center_axis',(0.890557268264347,0.,-0.454871137731933));
#31720=DIRECTION('ref_axis',(-0.454871137731933,0.,-0.890557268264347));
#31721=DIRECTION('',(0.,1.,0.));
#31722=DIRECTION('center_axis',(-0.408542131361568,0.,-0.912739462772673));
#31723=DIRECTION('ref_axis',(-0.912739462772673,0.,0.408542131361568));
#31724=DIRECTION('',(0.,1.,0.));
#31725=DIRECTION('center_axis',(-0.238261269596263,0.,-0.971201095247723));
#31726=DIRECTION('ref_axis',(-0.971201095247723,0.,0.238261269596263));
#31727=DIRECTION('center_axis',(0.0956909360030992,0.,-0.99541109335131));
#31728=DIRECTION('ref_axis',(-0.99541109335131,0.,-0.0956909360030991));
#31729=DIRECTION('',(0.,1.,0.));
#31730=DIRECTION('center_axis',(0.169258283051569,0.,-0.98557172931169));
#31731=DIRECTION('ref_axis',(-0.98557172931169,0.,-0.169258283051569));
#31732=DIRECTION('',(0.,1.,0.));
#31733=DIRECTION('center_axis',(0.235674098326418,0.,-0.971832145680534));
#31734=DIRECTION('ref_axis',(-0.971832145680534,0.,-0.235674098326418));
#31735=DIRECTION('',(0.,1.,0.));
#31736=DIRECTION('center_axis',(0.29662964900741,0.,-0.954992592290506));
#31737=DIRECTION('ref_axis',(-0.954992592290506,0.,-0.29662964900741));
#31738=DIRECTION('',(0.,1.,0.));
#31739=DIRECTION('center_axis',(0.3531573427799,0.,-0.935563942892542));
#31740=DIRECTION('ref_axis',(-0.935563942892542,0.,-0.3531573427799));
#31741=DIRECTION('',(0.,1.,0.));
#31742=DIRECTION('center_axis',(0.959936777257017,0.,-0.280216672718472));
#31743=DIRECTION('ref_axis',(-0.280216672718472,0.,-0.959936777257017));
#31744=DIRECTION('',(0.,1.,0.));
#31745=DIRECTION('center_axis',(0.963982324735009,0.,-0.265966309141757));
#31746=DIRECTION('ref_axis',(-0.265966309141757,0.,-0.963982324735009));
#31747=DIRECTION('',(0.,1.,0.));
#31748=DIRECTION('center_axis',(0.967816336590577,0.,-0.251657582099955));
#31749=DIRECTION('ref_axis',(-0.251657582099955,0.,-0.967816336590577));
#31750=DIRECTION('',(0.,1.,0.));
#31751=DIRECTION('center_axis',(0.971437971490778,0.,-0.237293631490361));
#31752=DIRECTION('ref_axis',(-0.237293631490361,0.,-0.971437971490778));
#31753=DIRECTION('',(0.,1.,0.));
#31754=DIRECTION('center_axis',(0.773625201826675,0.,0.633643470019724));
#31755=DIRECTION('ref_axis',(0.633643470019724,0.,-0.773625201826675));
#31756=DIRECTION('',(0.,1.,0.));
#31757=DIRECTION('center_axis',(0.734385107701329,0.,0.678733020845831));
#31758=DIRECTION('ref_axis',(0.678733020845831,0.,-0.734385107701329));
#31759=DIRECTION('',(0.,1.,0.));
#31760=DIRECTION('center_axis',(0.690015829004945,0.,0.723794277210464));
#31761=DIRECTION('ref_axis',(0.723794277210464,0.,-0.690015829004945));
#31762=DIRECTION('',(0.,1.,0.));
#31763=DIRECTION('center_axis',(0.639367837579431,0.,0.768901013309907));
#31764=DIRECTION('ref_axis',(0.768901013309907,0.,-0.639367837579431));
#31765=DIRECTION('',(0.,1.,0.));
#31766=DIRECTION('center_axis',(0.580576328166249,0.,0.814205826049529));
#31767=DIRECTION('ref_axis',(0.814205826049529,0.,-0.580576328166249));
#31768=DIRECTION('',(0.,1.,0.));
#31769=DIRECTION('center_axis',(0.510236429716898,0.,0.860034177105627));
#31770=DIRECTION('ref_axis',(0.860034177105627,0.,-0.510236429716898));
#31771=DIRECTION('',(0.,1.,0.));
#31772=DIRECTION('center_axis',(0.420671769125548,0.,0.907212909222957));
#31773=DIRECTION('ref_axis',(0.907212909222957,0.,-0.420671769125548));
#31774=DIRECTION('center_axis',(0.998680786707765,0.,-0.0513486734079878));
#31775=DIRECTION('ref_axis',(-0.0513486734079878,0.,-0.998680786707765));
#31776=DIRECTION('',(0.,1.,0.));
#31777=DIRECTION('center_axis',(0.998680786707765,0.,0.0513486734079865));
#31778=DIRECTION('ref_axis',(0.0513486734079865,0.,-0.998680786707765));
#31779=DIRECTION('',(0.,1.,0.));
#31780=DIRECTION('center_axis',(0.102561867110979,0.,-0.99472662747848));
#31781=DIRECTION('ref_axis',(-0.99472662747848,0.,-0.102561867110979));
#31782=DIRECTION('',(0.,1.,0.));
#31783=DIRECTION('center_axis',(0.279260235415567,0.,-0.960215455465929));
#31784=DIRECTION('ref_axis',(-0.960215455465929,0.,-0.279260235415567));
#31785=DIRECTION('center_axis',(0.580576328166254,0.,-0.814205826049526));
#31786=DIRECTION('ref_axis',(-0.814205826049526,0.,-0.580576328166254));
#31787=DIRECTION('',(0.,1.,0.));
#31788=DIRECTION('center_axis',(0.639367837579427,0.,-0.768901013309911));
#31789=DIRECTION('ref_axis',(-0.768901013309911,0.,-0.639367837579427));
#31790=DIRECTION('',(0.,1.,0.));
#31791=DIRECTION('center_axis',(0.690015829004942,0.,-0.723794277210468));
#31792=DIRECTION('ref_axis',(-0.723794277210468,0.,-0.690015829004942));
#31793=DIRECTION('',(0.,1.,0.));
#31794=DIRECTION('center_axis',(0.734385107701332,0.,-0.678733020845828));
#31795=DIRECTION('ref_axis',(-0.678733020845828,0.,-0.734385107701332));
#31796=DIRECTION('',(0.,1.,0.));
#31797=DIRECTION('center_axis',(0.773625201826672,0.,-0.633643470019728));
#31798=DIRECTION('ref_axis',(-0.633643470019728,0.,-0.773625201826672));
#31799=DIRECTION('',(0.,1.,0.));
#31800=DIRECTION('center_axis',(0.971437971490777,0.,0.237293631490364));
#31801=DIRECTION('ref_axis',(0.237293631490364,0.,-0.971437971490777));
#31802=DIRECTION('',(0.,1.,0.));
#31803=DIRECTION('center_axis',(0.967816336590574,0.,0.251657582099965));
#31804=DIRECTION('ref_axis',(0.251657582099965,0.,-0.967816336590574));
#31805=DIRECTION('',(0.,1.,0.));
#31806=DIRECTION('center_axis',(0.963982324735012,0.,0.265966309141746));
#31807=DIRECTION('ref_axis',(0.265966309141746,0.,-0.963982324735012));
#31808=DIRECTION('',(0.,1.,0.));
#31809=DIRECTION('center_axis',(0.959936777257017,0.,0.280216672718472));
#31810=DIRECTION('ref_axis',(0.280216672718472,0.,-0.959936777257017));
#31811=DIRECTION('',(0.,1.,0.));
#31812=DIRECTION('center_axis',(0.353157342779907,0.,0.93556394289254));
#31813=DIRECTION('ref_axis',(0.93556394289254,0.,-0.353157342779907));
#31814=DIRECTION('',(0.,1.,0.));
#31815=DIRECTION('center_axis',(0.29662964900741,0.,0.954992592290506));
#31816=DIRECTION('ref_axis',(0.954992592290506,0.,-0.29662964900741));
#31817=DIRECTION('',(0.,1.,0.));
#31818=DIRECTION('center_axis',(0.235674098326429,0.,0.971832145680531));
#31819=DIRECTION('ref_axis',(0.971832145680531,0.,-0.235674098326429));
#31820=DIRECTION('',(0.,1.,0.));
#31821=DIRECTION('center_axis',(0.169258283051549,0.,0.985571729311693));
#31822=DIRECTION('ref_axis',(0.985571729311693,0.,-0.169258283051549));
#31823=DIRECTION('',(0.,1.,0.));
#31824=DIRECTION('center_axis',(0.0956909360031064,0.,0.99541109335131));
#31825=DIRECTION('ref_axis',(0.995411093351309,0.,-0.0956909360031064));
#31826=DIRECTION('',(0.,1.,0.));
#31827=DIRECTION('center_axis',(0.0118606215182996,0.,0.999929660354767));
#31828=DIRECTION('ref_axis',(0.999929660354767,0.,-0.0118606215182996));
#31829=DIRECTION('',(0.,1.,0.));
#31830=DIRECTION('center_axis',(-0.0892940158938297,0.,0.996005310591039));
#31831=DIRECTION('ref_axis',(0.996005310591039,0.,0.0892940158938297));
#31832=DIRECTION('center_axis',(0.890557268264347,0.,0.454871137731933));
#31833=DIRECTION('ref_axis',(0.454871137731933,0.,-0.890557268264347));
#31834=DIRECTION('',(0.,1.,0.));
#31835=DIRECTION('center_axis',(0.839208594856359,0.,0.54380964897583));
#31836=DIRECTION('ref_axis',(0.54380964897583,0.,-0.839208594856359));
#31837=DIRECTION('',(0.,1.,0.));
#31838=DIRECTION('center_axis',(0.586184496116911,0.,-0.810177595661694));
#31839=DIRECTION('ref_axis',(-0.810177595661694,0.,-0.586184496116911));
#31840=DIRECTION('',(0.,1.,0.));
#31841=DIRECTION('center_axis',(0.721954185869668,0.,-0.691940859832157));
#31842=DIRECTION('ref_axis',(-0.691940859832157,0.,-0.721954185869668));
#31843=DIRECTION('center_axis',(0.909896762052629,0.,-0.414834765185058));
#31844=DIRECTION('ref_axis',(-0.414834765185058,0.,-0.909896762052629));
#31845=DIRECTION('',(0.,1.,0.));
#31846=DIRECTION('center_axis',(0.938159296361463,0.,-0.346203891732264));
#31847=DIRECTION('ref_axis',(-0.346203891732264,0.,-0.938159296361463));
#31848=DIRECTION('',(0.,1.,0.));
#31849=DIRECTION('center_axis',(0.959468375536894,0.,-0.281816316675586));
#31850=DIRECTION('ref_axis',(-0.281816316675586,0.,-0.959468375536894));
#31851=DIRECTION('',(0.,1.,0.));
#31852=DIRECTION('center_axis',(0.975362669853238,0.,-0.220607484589178));
#31853=DIRECTION('ref_axis',(-0.220607484589178,0.,-0.975362669853237));
#31854=DIRECTION('',(0.,1.,0.));
#31855=DIRECTION('center_axis',(0.986800812799626,0.,-0.161938741065869));
#31856=DIRECTION('ref_axis',(-0.161938741065869,0.,-0.986800812799626));
#31857=DIRECTION('',(0.,1.,0.));
#31858=DIRECTION('center_axis',(0.722643145766656,0.,0.691221298772304));
#31859=DIRECTION('ref_axis',(0.691221298772304,0.,-0.722643145766656));
#31860=DIRECTION('',(0.,1.,0.));
#31861=DIRECTION('center_axis',(0.712324742635051,0.,0.701850027448819));
#31862=DIRECTION('ref_axis',(0.701850027448819,0.,-0.712324742635051));
#31863=DIRECTION('',(0.,1.,0.));
#31864=DIRECTION('center_axis',(0.701850027448819,0.,0.712324742635051));
#31865=DIRECTION('ref_axis',(0.712324742635051,0.,-0.701850027448819));
#31866=DIRECTION('',(0.,1.,0.));
#31867=DIRECTION('center_axis',(0.691221298772308,0.,0.722643145766653));
#31868=DIRECTION('ref_axis',(0.722643145766653,0.,-0.691221298772308));
#31869=DIRECTION('',(0.,1.,0.));
#31870=DIRECTION('center_axis',(-0.161938741065865,0.,0.986800812799626));
#31871=DIRECTION('ref_axis',(0.986800812799626,0.,0.161938741065865));
#31872=DIRECTION('',(0.,1.,0.));
#31873=DIRECTION('center_axis',(-0.220607484589183,0.,0.975362669853236));
#31874=DIRECTION('ref_axis',(0.975362669853236,0.,0.220607484589183));
#31875=DIRECTION('',(0.,1.,0.));
#31876=DIRECTION('center_axis',(-0.28181631667558,0.,0.959468375536896));
#31877=DIRECTION('ref_axis',(0.959468375536896,0.,0.28181631667558));
#31878=DIRECTION('',(0.,1.,0.));
#31879=DIRECTION('center_axis',(-0.346203891732262,0.,0.938159296361464));
#31880=DIRECTION('ref_axis',(0.938159296361463,0.,0.346203891732262));
#31881=DIRECTION('',(0.,1.,0.));
#31882=DIRECTION('center_axis',(-0.414834765185062,0.,0.909896762052627));
#31883=DIRECTION('ref_axis',(0.909896762052626,0.,0.414834765185062));
#31884=DIRECTION('',(0.,1.,0.));
#31885=DIRECTION('center_axis',(-0.489693230637852,0.,0.87189479862393));
#31886=DIRECTION('ref_axis',(0.87189479862393,0.,0.489693230637852));
#31887=DIRECTION('',(0.,1.,0.));
#31888=DIRECTION('center_axis',(-0.575333541465516,0.,0.817918893329129));
#31889=DIRECTION('ref_axis',(0.817918893329129,0.,0.575333541465516));
#31890=DIRECTION('center_axis',(0.543809648975832,0.,0.839208594856358));
#31891=DIRECTION('ref_axis',(0.839208594856358,0.,-0.543809648975832));
#31892=DIRECTION('center_axis',(0.,1.,0.));
#31893=DIRECTION('ref_axis',(0.,0.,1.));
#31894=DIRECTION('',(0.,-1.,0.));
#31895=DIRECTION('center_axis',(0.,1.,0.));
#31896=DIRECTION('ref_axis',(1.,0.,0.));
#31897=DIRECTION('center_axis',(0.,-1.,0.));
#31898=DIRECTION('ref_axis',(0.,0.,-1.));
#31899=DIRECTION('center_axis',(0.,1.,0.));
#31900=DIRECTION('ref_axis',(0.,0.,1.));
#31901=DIRECTION('center_axis',(0.,1.,0.));
#31902=DIRECTION('ref_axis',(1.,0.,0.));
#31903=DIRECTION('',(0.,-1.,0.));
#31904=DIRECTION('center_axis',(0.,1.,0.));
#31905=DIRECTION('ref_axis',(0.,0.,1.));
#38096=CARTESIAN_POINT('',(0.,0.,0.));
#38097=CARTESIAN_POINT('Origin',(5.91118355257506,37.28,-28.4145311199496));
#38098=CARTESIAN_POINT('',(12.8183396498506,37.2481324154382,-23.3776905273493));
#38099=CARTESIAN_POINT('',(13.0730690072096,37.03,-22.9241469865312));
#38100=CARTESIAN_POINT('',(11.3376395086249,38.5161005118286,-26.014065038336));
#38101=CARTESIAN_POINT('',(10.3106808445568,37.03,-24.9228064432661));
#38102=CARTESIAN_POINT('',(5.76463742854583,37.03,-28.2119867210341));
#38103=CARTESIAN_POINT('',(10.5829448433309,37.53,-25.3429650194728));
#38104=CARTESIAN_POINT('',(10.4860359897738,37.3520314584495,-25.1934150014179));
#38105=CARTESIAN_POINT('',(12.1154593532086,37.53,-24.23415103773));
#38106=CARTESIAN_POINT('',(6.05772967660429,37.53,-28.617075518865));
#38107=CARTESIAN_POINT('',(12.4929286389212,37.4321844925501,-23.8403088083181));
#38108=CARTESIAN_POINT('',(9.89277877754194,38.1059743550985,-26.5532416401305));
#38109=CARTESIAN_POINT('',(10.7287682421066,38.4299914950389,-26.3483150610773));
#38110=CARTESIAN_POINT('Origin',(2.22044604925031E-15,37.03,-33.));
#38111=CARTESIAN_POINT('',(11.3124568369342,37.03,-26.46875));
#38112=CARTESIAN_POINT('',(11.3124568369342,37.03,-26.46875));
#38113=CARTESIAN_POINT('',(13.1048089083576,37.03,-22.8676343517052));
#38114=CARTESIAN_POINT('',(12.8183396498506,37.03,-23.3776905273493));
#38115=CARTESIAN_POINT('',(13.3555043472661,37.03,-22.3177600709842));
#38116=CARTESIAN_POINT('',(13.1048089083576,37.03,-22.8676343517052));
#38117=CARTESIAN_POINT('',(13.571408774188,37.03,-21.7326922826676));
#38118=CARTESIAN_POINT('',(13.3555043472661,37.03,-22.3177600709842));
#38119=CARTESIAN_POINT('',(13.7525975185565,37.03,-21.1158193057032));
#38120=CARTESIAN_POINT('',(13.571408774188,37.03,-21.7326922826676));
#38121=CARTESIAN_POINT('',(13.8986893840657,37.03,-20.4699094343666));
#38122=CARTESIAN_POINT('',(13.7525975185565,37.03,-21.1158193057032));
#38123=CARTESIAN_POINT('',(14.009053161491,37.03,-19.7973892915637));
#38124=CARTESIAN_POINT('',(13.8986893840657,37.03,-20.4699094343666));
#38125=CARTESIAN_POINT('',(13.8119447915281,37.03,-19.5913206811491));
#38126=CARTESIAN_POINT('',(14.009053161491,37.03,-19.7973892915637));
#38127=CARTESIAN_POINT('',(13.611805537841,37.03,-19.388194462159));
#38128=CARTESIAN_POINT('',(13.8119447915281,37.03,-19.5913206811491));
#38129=CARTESIAN_POINT('',(13.4086793188509,37.03,-19.1880552084719));
#38130=CARTESIAN_POINT('',(13.611805537841,37.03,-19.388194462159));
#38131=CARTESIAN_POINT('',(13.2026107084364,37.03,-18.990946838509));
#38132=CARTESIAN_POINT('',(13.4086793188509,37.03,-19.1880552084719));
#38133=CARTESIAN_POINT('',(12.5300905656334,37.03,-19.1013106159343));
#38134=CARTESIAN_POINT('',(13.2026107084364,37.03,-18.990946838509));
#38135=CARTESIAN_POINT('',(11.8841806942968,37.03,-19.2474024814435));
#38136=CARTESIAN_POINT('',(12.5300905656334,37.03,-19.1013106159343));
#38137=CARTESIAN_POINT('',(11.2673077173324,37.03,-19.428591225812));
#38138=CARTESIAN_POINT('',(11.8841806942968,37.03,-19.2474024814435));
#38139=CARTESIAN_POINT('',(10.6822399290158,37.03,-19.6444956527339));
#38140=CARTESIAN_POINT('',(11.2673077173324,37.03,-19.428591225812));
#38141=CARTESIAN_POINT('',(10.1323656482948,37.03,-19.8951910916424));
#38142=CARTESIAN_POINT('',(10.6822399290158,37.03,-19.6444956527339));
#38143=CARTESIAN_POINT('',(10.0758530134688,37.03,-19.9269309927904));
#38144=CARTESIAN_POINT('',(10.1323656482948,37.03,-19.8951910916424));
#38145=CARTESIAN_POINT('',(8.07719355673392,37.03,-22.6893191554432));
#38146=CARTESIAN_POINT('',(4.23360628809444,37.03,-28.001619826393));
#38147=CARTESIAN_POINT('',(6.53125,37.03,-21.6875431630658));
#38148=CARTESIAN_POINT('',(7.65703498052716,37.03,-22.4170551566691));
#38149=CARTESIAN_POINT('',(4.8907147633328,37.03,-20.8496047663061));
#38150=CARTESIAN_POINT('',(6.53125,37.03,-21.6875431630658));
#38151=CARTESIAN_POINT('',(6.28368335893611,37.03,-17.7375208219333));
#38152=CARTESIAN_POINT('',(2.59831581724435,37.03,-25.9711401524854));
#38153=CARTESIAN_POINT('',(6.28291460223091,37.03,-17.6727094939652));
#38154=CARTESIAN_POINT('',(6.28985303478256,37.03,-18.2576657286835));
#38155=CARTESIAN_POINT('',(6.22508608057805,37.03,-17.0711566785188));
#38156=CARTESIAN_POINT('',(6.28291460223091,37.03,-17.6727094939652));
#38157=CARTESIAN_POINT('',(6.11953090492364,37.03,-16.4565208974396));
#38158=CARTESIAN_POINT('',(6.22508608057805,37.03,-17.0711566785188));
#38159=CARTESIAN_POINT('',(5.96800847194436,37.03,-15.8316988562961));
#38160=CARTESIAN_POINT('',(6.11953090492364,37.03,-16.4565208974396));
#38161=CARTESIAN_POINT('',(5.77157280309329,37.03,-15.1992785664089));
#38162=CARTESIAN_POINT('',(5.96800847194436,37.03,-15.8316988562961));
#38163=CARTESIAN_POINT('',(5.53089056659976,37.03,-14.5616771494721));
#38164=CARTESIAN_POINT('',(5.77157280309329,37.03,-15.1992785664089));
#38165=CARTESIAN_POINT('',(5.25715540570603,37.03,-14.481770682912));
#38166=CARTESIAN_POINT('',(5.53089056659976,37.03,-14.5616771494721));
#38167=CARTESIAN_POINT('',(4.98226661822352,37.03,-14.4059278439354));
#38168=CARTESIAN_POINT('',(5.25715540570603,37.03,-14.481770682912));
#38169=CARTESIAN_POINT('',(4.70628452555987,37.03,-14.3341652754431));
#38170=CARTESIAN_POINT('',(4.98226661822352,37.03,-14.4059278439354));
#38171=CARTESIAN_POINT('',(4.42926968903683,37.03,-14.2664987249639));
#38172=CARTESIAN_POINT('',(4.70628452555987,37.03,-14.3341652754431));
#38173=CARTESIAN_POINT('',(3.90203204952539,37.03,-14.6983366312733));
#38174=CARTESIAN_POINT('',(4.42926968903683,37.03,-14.2664987249639));
#38175=CARTESIAN_POINT('',(3.41570362514739,37.03,-15.1478108337588));
#38176=CARTESIAN_POINT('',(3.90203204952539,37.03,-14.6983366312733));
#38177=CARTESIAN_POINT('',(2.97207032837233,37.03,-15.6131613777439));
#38178=CARTESIAN_POINT('',(3.41570362514739,37.03,-15.1478108337588));
#38179=CARTESIAN_POINT('',(2.57333897421511,37.03,-16.0926739904062));
#38180=CARTESIAN_POINT('',(2.97207032837233,37.03,-15.6131613777439));
#38181=CARTESIAN_POINT('',(2.22248159767725,37.03,-16.5847197494743));
#38182=CARTESIAN_POINT('',(2.57333897421511,37.03,-16.0926739904062));
#38183=CARTESIAN_POINT('',(2.18941017085717,37.03,-16.6404636275951));
#38184=CARTESIAN_POINT('',(2.22248159767725,37.03,-16.5847197494743));
#38185=CARTESIAN_POINT('',(1.83971438913717,37.03,-20.0320916799333));
#38186=CARTESIAN_POINT('',(1.16722050830783,37.03,-26.5544726478367));
#38187=CARTESIAN_POINT('',(7.99847440693115E-16,37.03,-19.9375));
#38188=CARTESIAN_POINT('',(1.33971438913717,37.03,-20.0063834285624));
#38189=CARTESIAN_POINT('',(-1.83971438913717,37.03,-20.0320916799333));
#38190=CARTESIAN_POINT('',(7.99847440693115E-16,37.03,-19.9375));
#38191=CARTESIAN_POINT('',(-2.18941017085717,37.03,-16.6404636275951));
#38192=CARTESIAN_POINT('',(-1.26422241896876,37.03,-25.6136709037898));
#38193=CARTESIAN_POINT('',(-2.22248159767725,37.03,-16.5847197494743));
#38194=CARTESIAN_POINT('',(-1.92399462146589,37.03,-17.0878374925667));
#38195=CARTESIAN_POINT('',(-2.57333897421511,37.03,-16.0926739904062));
#38196=CARTESIAN_POINT('',(-2.22248159767725,37.03,-16.5847197494743));
#38197=CARTESIAN_POINT('',(-2.97207032837233,37.03,-15.6131613777439));
#38198=CARTESIAN_POINT('',(-2.57333897421511,37.03,-16.0926739904062));
#38199=CARTESIAN_POINT('',(-3.4157036251474,37.03,-15.1478108337588));
#38200=CARTESIAN_POINT('',(-2.97207032837233,37.03,-15.6131613777439));
#38201=CARTESIAN_POINT('',(-3.90203204952539,37.03,-14.6983366312733));
#38202=CARTESIAN_POINT('',(-3.4157036251474,37.03,-15.1478108337588));
#38203=CARTESIAN_POINT('',(-4.42926968903683,37.03,-14.2664987249639));
#38204=CARTESIAN_POINT('',(-3.90203204952539,37.03,-14.6983366312733));
#38205=CARTESIAN_POINT('',(-4.70628452555987,37.03,-14.3341652754431));
#38206=CARTESIAN_POINT('',(-4.42926968903683,37.03,-14.2664987249639));
#38207=CARTESIAN_POINT('',(-4.98226661822353,37.03,-14.4059278439354));
#38208=CARTESIAN_POINT('',(-4.70628452555987,37.03,-14.3341652754431));
#38209=CARTESIAN_POINT('',(-5.25715540570604,37.03,-14.481770682912));
#38210=CARTESIAN_POINT('',(-4.98226661822353,37.03,-14.4059278439354));
#38211=CARTESIAN_POINT('',(-5.53089056659977,37.03,-14.5616771494721));
#38212=CARTESIAN_POINT('',(-5.25715540570604,37.03,-14.481770682912));
#38213=CARTESIAN_POINT('',(-5.7715728030933,37.03,-15.1992785664089));
#38214=CARTESIAN_POINT('',(-5.53089056659977,37.03,-14.5616771494721));
#38215=CARTESIAN_POINT('',(-5.96800847194436,37.03,-15.8316988562961));
#38216=CARTESIAN_POINT('',(-5.7715728030933,37.03,-15.1992785664089));
#38217=CARTESIAN_POINT('',(-6.11953090492364,37.03,-16.4565208974396));
#38218=CARTESIAN_POINT('',(-5.96800847194436,37.03,-15.8316988562961));
#38219=CARTESIAN_POINT('',(-6.22508608057805,37.03,-17.0711566785188));
#38220=CARTESIAN_POINT('',(-6.11953090492364,37.03,-16.4565208974396));
#38221=CARTESIAN_POINT('',(-6.28291460223091,37.03,-17.6727094939652));
#38222=CARTESIAN_POINT('',(-6.22508608057805,37.03,-17.0711566785188));
#38223=CARTESIAN_POINT('',(-6.28368335893612,37.03,-17.7375208219333));
#38224=CARTESIAN_POINT('',(-6.28291460223091,37.03,-17.6727094939652));
#38225=CARTESIAN_POINT('',(-4.8907147633328,37.03,-20.8496047663061));
#38226=CARTESIAN_POINT('',(-2.21192106406889,37.03,-26.8343993180852));
#38227=CARTESIAN_POINT('',(-6.53125,37.03,-21.6875431630658));
#38228=CARTESIAN_POINT('',(-5.33658159091048,37.03,-21.077340767532));
#38229=CARTESIAN_POINT('',(-8.07719355673392,37.03,-22.6893191554432));
#38230=CARTESIAN_POINT('',(-6.53125,37.03,-21.6875431630658));
#38231=CARTESIAN_POINT('',(-10.0758530134688,37.03,-19.9269309927904));
#38232=CARTESIAN_POINT('',(-4.78801327896586,37.03,-27.2353625714542));
#38233=CARTESIAN_POINT('',(-10.1323656482948,37.03,-19.8951910916424));
#38234=CARTESIAN_POINT('',(-9.62230947265072,37.03,-20.1816603501494));
#38235=CARTESIAN_POINT('',(-10.6822399290158,37.03,-19.6444956527339));
#38236=CARTESIAN_POINT('',(-10.1323656482948,37.03,-19.8951910916424));
#38237=CARTESIAN_POINT('',(-11.2673077173324,37.03,-19.428591225812));
#38238=CARTESIAN_POINT('',(-10.6822399290158,37.03,-19.6444956527339));
#38239=CARTESIAN_POINT('',(-11.8841806942968,37.03,-19.2474024814435));
#38240=CARTESIAN_POINT('',(-11.2673077173324,37.03,-19.428591225812));
#38241=CARTESIAN_POINT('',(-12.5300905656334,37.03,-19.1013106159343));
#38242=CARTESIAN_POINT('',(-11.8841806942968,37.03,-19.2474024814435));
#38243=CARTESIAN_POINT('',(-13.2026107084363,37.03,-18.990946838509));
#38244=CARTESIAN_POINT('',(-12.5300905656334,37.03,-19.1013106159343));
#38245=CARTESIAN_POINT('',(-13.4086793188509,37.03,-19.1880552084719));
#38246=CARTESIAN_POINT('',(-13.2026107084363,37.03,-18.990946838509));
#38247=CARTESIAN_POINT('',(-13.611805537841,37.03,-19.388194462159));
#38248=CARTESIAN_POINT('',(-13.4086793188509,37.03,-19.1880552084719));
#38249=CARTESIAN_POINT('',(-13.8119447915281,37.03,-19.5913206811491));
#38250=CARTESIAN_POINT('',(-13.611805537841,37.03,-19.388194462159));
#38251=CARTESIAN_POINT('',(-14.009053161491,37.03,-19.7973892915637));
#38252=CARTESIAN_POINT('',(-13.8119447915281,37.03,-19.5913206811491));
#38253=CARTESIAN_POINT('',(-13.8986893840657,37.03,-20.4699094343666));
#38254=CARTESIAN_POINT('',(-14.009053161491,37.03,-19.7973892915637));
#38255=CARTESIAN_POINT('',(-13.7525975185565,37.03,-21.1158193057032));
#38256=CARTESIAN_POINT('',(-13.8986893840657,37.03,-20.4699094343666));
#38257=CARTESIAN_POINT('',(-13.571408774188,37.03,-21.7326922826676));
#38258=CARTESIAN_POINT('',(-13.7525975185565,37.03,-21.1158193057032));
#38259=CARTESIAN_POINT('',(-13.3555043472661,37.03,-22.3177600709842));
#38260=CARTESIAN_POINT('',(-13.571408774188,37.03,-21.7326922826676));
#38261=CARTESIAN_POINT('',(-13.1048089083576,37.03,-22.8676343517052));
#38262=CARTESIAN_POINT('',(-13.3555043472661,37.03,-22.3177600709842));
#38263=CARTESIAN_POINT('',(-13.0730690072096,37.03,-22.9241469865312));
#38264=CARTESIAN_POINT('',(-13.1048089083576,37.03,-22.8676343517052));
#38265=CARTESIAN_POINT('',(-10.3106808445568,37.03,-24.9228064432661));
#38266=CARTESIAN_POINT('',(-4.99838017360698,37.03,-28.7663937119056));
#38267=CARTESIAN_POINT('',(-11.3124568369342,37.03,-26.46875));
#38268=CARTESIAN_POINT('',(-10.5829448433309,37.03,-25.3429650194728));
#38269=CARTESIAN_POINT('',(-12.1503952336939,37.03,-28.1092852366672));
#38270=CARTESIAN_POINT('',(-11.3124568369342,37.03,-26.46875));
#38271=CARTESIAN_POINT('',(-15.2624791780667,37.03,-26.7163166410639));
#38272=CARTESIAN_POINT('',(-7.02885984751459,37.03,-30.4016841827556));
#38273=CARTESIAN_POINT('',(-15.3272905060348,37.03,-26.7170853977691));
#38274=CARTESIAN_POINT('',(-14.7423342713164,37.03,-26.7101469652174));
#38275=CARTESIAN_POINT('',(-15.9288433214812,37.03,-26.7749139194219));
#38276=CARTESIAN_POINT('',(-15.3272905060348,37.03,-26.7170853977691));
#38277=CARTESIAN_POINT('',(-16.5434791025604,37.03,-26.8804690950764));
#38278=CARTESIAN_POINT('',(-15.9288433214812,37.03,-26.7749139194219));
#38279=CARTESIAN_POINT('',(-17.1683011437039,37.03,-27.0319915280556));
#38280=CARTESIAN_POINT('',(-16.5434791025604,37.03,-26.8804690950764));
#38281=CARTESIAN_POINT('',(-17.8007214335911,37.03,-27.2284271969067));
#38282=CARTESIAN_POINT('',(-17.1683011437039,37.03,-27.0319915280556));
#38283=CARTESIAN_POINT('',(-18.4383228505279,37.03,-27.4691094334002));
#38284=CARTESIAN_POINT('',(-17.8007214335911,37.03,-27.2284271969067));
#38285=CARTESIAN_POINT('',(-18.518229317088,37.03,-27.742844594294));
#38286=CARTESIAN_POINT('',(-18.4383228505279,37.03,-27.4691094334002));
#38287=CARTESIAN_POINT('',(-18.5940721560646,37.03,-28.0177333817765));
#38288=CARTESIAN_POINT('',(-18.518229317088,37.03,-27.742844594294));
#38289=CARTESIAN_POINT('',(-18.6658347245569,37.03,-28.2937154744401));
#38290=CARTESIAN_POINT('',(-18.5940721560646,37.03,-28.0177333817765));
#38291=CARTESIAN_POINT('',(-18.7335012750361,37.03,-28.5707303109632));
#38292=CARTESIAN_POINT('',(-18.6658347245569,37.03,-28.2937154744401));
#38293=CARTESIAN_POINT('',(-18.3016633687267,37.03,-29.0979679504746));
#38294=CARTESIAN_POINT('',(-18.7335012750361,37.03,-28.5707303109632));
#38295=CARTESIAN_POINT('',(-17.8521891662412,37.03,-29.5842963748526));
#38296=CARTESIAN_POINT('',(-18.3016633687267,37.03,-29.0979679504746));
#38297=CARTESIAN_POINT('',(-17.3868386222561,37.03,-30.0279296716277));
#38298=CARTESIAN_POINT('',(-17.8521891662412,37.03,-29.5842963748526));
#38299=CARTESIAN_POINT('',(-16.9073260095938,37.03,-30.4266610257849));
#38300=CARTESIAN_POINT('',(-17.3868386222561,37.03,-30.0279296716277));
#38301=CARTESIAN_POINT('',(-16.4152802505257,37.03,-30.7775184023227));
#38302=CARTESIAN_POINT('',(-16.9073260095938,37.03,-30.4266610257849));
#38303=CARTESIAN_POINT('',(-16.3595363724049,37.03,-30.8105898291428));
#38304=CARTESIAN_POINT('',(-16.4152802505257,37.03,-30.7775184023227));
#38305=CARTESIAN_POINT('',(-12.9679083200667,37.03,-31.1602856108628));
#38306=CARTESIAN_POINT('',(-6.44552735216333,37.03,-31.8327794916922));
#38307=CARTESIAN_POINT('',(-13.0625,37.03,-33.));
#38308=CARTESIAN_POINT('',(-12.9936165714376,37.03,-31.6602856108628));
#38309=CARTESIAN_POINT('',(-12.9679083200667,37.03,-34.8397143891372));
#38310=CARTESIAN_POINT('',(-13.0625,37.03,-33.));
#38311=CARTESIAN_POINT('',(-16.3595363724049,37.03,-35.1894101708572));
#38312=CARTESIAN_POINT('',(-7.38632909621023,37.03,-34.2642224189688));
#38313=CARTESIAN_POINT('',(-16.4152802505257,37.03,-35.2224815976773));
#38314=CARTESIAN_POINT('',(-15.9121625074333,37.03,-34.9239946214659));
#38315=CARTESIAN_POINT('',(-16.9073260095938,37.03,-35.5733389742151));
#38316=CARTESIAN_POINT('',(-16.4152802505257,37.03,-35.2224815976773));
#38317=CARTESIAN_POINT('',(-17.3868386222561,37.03,-35.9720703283723));
#38318=CARTESIAN_POINT('',(-16.9073260095938,37.03,-35.5733389742151));
#38319=CARTESIAN_POINT('',(-17.8521891662412,37.03,-36.4157036251474));
#38320=CARTESIAN_POINT('',(-17.3868386222561,37.03,-35.9720703283723));
#38321=CARTESIAN_POINT('',(-18.3016633687267,37.03,-36.9020320495254));
#38322=CARTESIAN_POINT('',(-17.8521891662412,37.03,-36.4157036251474));
#38323=CARTESIAN_POINT('',(-18.7335012750361,37.03,-37.4292696890368));
#38324=CARTESIAN_POINT('',(-18.3016633687267,37.03,-36.9020320495254));
#38325=CARTESIAN_POINT('',(-18.6658347245569,37.03,-37.7062845255599));
#38326=CARTESIAN_POINT('',(-18.7335012750361,37.03,-37.4292696890368));
#38327=CARTESIAN_POINT('',(-18.5940721560646,37.03,-37.9822666182235));
#38328=CARTESIAN_POINT('',(-18.6658347245569,37.03,-37.7062845255599));
#38329=CARTESIAN_POINT('',(-18.518229317088,37.03,-38.257155405706));
#38330=CARTESIAN_POINT('',(-18.5940721560646,37.03,-37.9822666182235));
#38331=CARTESIAN_POINT('',(-18.4383228505279,37.03,-38.5308905665998));
#38332=CARTESIAN_POINT('',(-18.518229317088,37.03,-38.257155405706));
#38333=CARTESIAN_POINT('',(-17.8007214335911,37.03,-38.7715728030933));
#38334=CARTESIAN_POINT('',(-18.4383228505279,37.03,-38.5308905665998));
#38335=CARTESIAN_POINT('',(-17.1683011437039,37.03,-38.9680084719444));
#38336=CARTESIAN_POINT('',(-17.8007214335911,37.03,-38.7715728030933));
#38337=CARTESIAN_POINT('',(-16.5434791025604,37.03,-39.1195309049236));
#38338=CARTESIAN_POINT('',(-17.1683011437039,37.03,-38.9680084719444));
#38339=CARTESIAN_POINT('',(-15.9288433214812,37.03,-39.225086080578));
#38340=CARTESIAN_POINT('',(-16.5434791025604,37.03,-39.1195309049236));
#38341=CARTESIAN_POINT('',(-15.3272905060348,37.03,-39.2829146022309));
#38342=CARTESIAN_POINT('',(-15.9288433214812,37.03,-39.225086080578));
#38343=CARTESIAN_POINT('',(-15.2624791780667,37.03,-39.2836833589361));
#38344=CARTESIAN_POINT('',(-15.3272905060348,37.03,-39.2829146022309));
#38345=CARTESIAN_POINT('',(-12.1503952336939,37.03,-37.8907147633328));
#38346=CARTESIAN_POINT('',(-6.16560068191481,37.03,-35.2119210640689));
#38347=CARTESIAN_POINT('',(-11.3124568369342,37.03,-39.53125));
#38348=CARTESIAN_POINT('',(-11.922659232468,37.03,-38.3365815909105));
#38349=CARTESIAN_POINT('',(-10.3106808445568,37.03,-41.0771935567339));
#38350=CARTESIAN_POINT('',(-11.3124568369342,37.03,-39.53125));
#38351=CARTESIAN_POINT('',(-13.0730690072096,37.03,-43.0758530134688));
#38352=CARTESIAN_POINT('',(-5.76463742854584,37.03,-37.7880132789659));
#38353=CARTESIAN_POINT('',(-13.1048089083576,37.03,-43.1323656482948));
#38354=CARTESIAN_POINT('',(-12.8183396498506,37.03,-42.6223094726507));
#38355=CARTESIAN_POINT('',(-13.3555043472661,37.03,-43.6822399290158));
#38356=CARTESIAN_POINT('',(-13.1048089083576,37.03,-43.1323656482948));
#38357=CARTESIAN_POINT('',(-13.571408774188,37.03,-44.2673077173324));
#38358=CARTESIAN_POINT('',(-13.3555043472661,37.03,-43.6822399290158));
#38359=CARTESIAN_POINT('',(-13.7525975185565,37.03,-44.8841806942968));
#38360=CARTESIAN_POINT('',(-13.571408774188,37.03,-44.2673077173324));
#38361=CARTESIAN_POINT('',(-13.8986893840657,37.03,-45.5300905656334));
#38362=CARTESIAN_POINT('',(-13.7525975185565,37.03,-44.8841806942968));
#38363=CARTESIAN_POINT('',(-14.009053161491,37.03,-46.2026107084363));
#38364=CARTESIAN_POINT('',(-13.8986893840657,37.03,-45.5300905656334));
#38365=CARTESIAN_POINT('',(-13.8119447915281,37.03,-46.4086793188509));
#38366=CARTESIAN_POINT('',(-14.009053161491,37.03,-46.2026107084363));
#38367=CARTESIAN_POINT('',(-13.611805537841,37.03,-46.611805537841));
#38368=CARTESIAN_POINT('',(-13.8119447915281,37.03,-46.4086793188509));
#38369=CARTESIAN_POINT('',(-13.4086793188509,37.03,-46.8119447915281));
#38370=CARTESIAN_POINT('',(-13.611805537841,37.03,-46.611805537841));
#38371=CARTESIAN_POINT('',(-13.2026107084363,37.03,-47.009053161491));
#38372=CARTESIAN_POINT('',(-13.4086793188509,37.03,-46.8119447915281));
#38373=CARTESIAN_POINT('',(-12.5300905656334,37.03,-46.8986893840657));
#38374=CARTESIAN_POINT('',(-13.2026107084363,37.03,-47.009053161491));
#38375=CARTESIAN_POINT('',(-11.8841806942968,37.03,-46.7525975185565));
#38376=CARTESIAN_POINT('',(-12.5300905656334,37.03,-46.8986893840657));
#38377=CARTESIAN_POINT('',(-11.2673077173324,37.03,-46.571408774188));
#38378=CARTESIAN_POINT('',(-11.8841806942968,37.03,-46.7525975185565));
#38379=CARTESIAN_POINT('',(-10.6822399290158,37.03,-46.3555043472661));
#38380=CARTESIAN_POINT('',(-11.2673077173324,37.03,-46.571408774188));
#38381=CARTESIAN_POINT('',(-10.1323656482948,37.03,-46.1048089083576));
#38382=CARTESIAN_POINT('',(-10.6822399290158,37.03,-46.3555043472661));
#38383=CARTESIAN_POINT('',(-10.0758530134688,37.03,-46.0730690072096));
#38384=CARTESIAN_POINT('',(-10.1323656482948,37.03,-46.1048089083576));
#38385=CARTESIAN_POINT('',(-8.07719355673392,37.03,-43.3106808445568));
#38386=CARTESIAN_POINT('',(-4.23360628809444,37.03,-37.998380173607));
#38387=CARTESIAN_POINT('',(-6.53125000000001,37.03,-44.3124568369342));
#38388=CARTESIAN_POINT('',(-7.65703498052716,37.03,-43.5829448433309));
#38389=CARTESIAN_POINT('',(-4.8907147633328,37.03,-45.1503952336939));
#38390=CARTESIAN_POINT('',(-6.53125000000001,37.03,-44.3124568369342));
#38391=CARTESIAN_POINT('',(-6.2836833589361,37.03,-48.2624791780667));
#38392=CARTESIAN_POINT('',(-2.59831581724436,37.03,-40.0288598475146));
#38393=CARTESIAN_POINT('',(-6.2829146022309,37.03,-48.3272905060348));
#38394=CARTESIAN_POINT('',(-6.28985303478255,37.03,-47.7423342713165));
#38395=CARTESIAN_POINT('',(-6.22508608057804,37.03,-48.9288433214812));
#38396=CARTESIAN_POINT('',(-6.2829146022309,37.03,-48.3272905060348));
#38397=CARTESIAN_POINT('',(-6.11953090492364,37.03,-49.5434791025604));
#38398=CARTESIAN_POINT('',(-6.22508608057804,37.03,-48.9288433214812));
#38399=CARTESIAN_POINT('',(-5.96800847194436,37.03,-50.1683011437039));
#38400=CARTESIAN_POINT('',(-6.11953090492364,37.03,-49.5434791025604));
#38401=CARTESIAN_POINT('',(-5.7715728030933,37.03,-50.8007214335911));
#38402=CARTESIAN_POINT('',(-5.96800847194436,37.03,-50.1683011437039));
#38403=CARTESIAN_POINT('',(-5.53089056659976,37.03,-51.4383228505279));
#38404=CARTESIAN_POINT('',(-5.7715728030933,37.03,-50.8007214335911));
#38405=CARTESIAN_POINT('',(-5.25715540570604,37.03,-51.518229317088));
#38406=CARTESIAN_POINT('',(-5.53089056659976,37.03,-51.4383228505279));
#38407=CARTESIAN_POINT('',(-4.98226661822352,37.03,-51.5940721560646));
#38408=CARTESIAN_POINT('',(-5.25715540570604,37.03,-51.518229317088));
#38409=CARTESIAN_POINT('',(-4.70628452555985,37.03,-51.6658347245569));
#38410=CARTESIAN_POINT('',(-4.98226661822352,37.03,-51.5940721560646));
#38411=CARTESIAN_POINT('',(-4.42926968903682,37.03,-51.7335012750361));
#38412=CARTESIAN_POINT('',(-4.70628452555985,37.03,-51.6658347245569));
#38413=CARTESIAN_POINT('',(-3.90203204952539,37.03,-51.3016633687267));
#38414=CARTESIAN_POINT('',(-4.42926968903682,37.03,-51.7335012750361));
#38415=CARTESIAN_POINT('',(-3.41570362514739,37.03,-50.8521891662412));
#38416=CARTESIAN_POINT('',(-3.90203204952539,37.03,-51.3016633687267));
#38417=CARTESIAN_POINT('',(-2.97207032837234,37.03,-50.3868386222561));
#38418=CARTESIAN_POINT('',(-3.41570362514739,37.03,-50.8521891662412));
#38419=CARTESIAN_POINT('',(-2.57333897421511,37.03,-49.9073260095938));
#38420=CARTESIAN_POINT('',(-2.97207032837234,37.03,-50.3868386222561));
#38421=CARTESIAN_POINT('',(-2.22248159767726,37.03,-49.4152802505257));
#38422=CARTESIAN_POINT('',(-2.57333897421511,37.03,-49.9073260095938));
#38423=CARTESIAN_POINT('',(-2.18941017085716,37.03,-49.3595363724049));
#38424=CARTESIAN_POINT('',(-2.22248159767726,37.03,-49.4152802505257));
#38425=CARTESIAN_POINT('',(-1.83971438913717,37.03,-45.9679083200667));
#38426=CARTESIAN_POINT('',(-1.16722050830782,37.03,-39.4455273521633));
#38427=CARTESIAN_POINT('',(-2.39954232207934E-15,37.03,-46.0625));
#38428=CARTESIAN_POINT('',(-1.33971438913717,37.03,-45.9936165714376));
#38429=CARTESIAN_POINT('',(1.83971438913716,37.03,-45.9679083200667));
#38430=CARTESIAN_POINT('',(-2.39954232207934E-15,37.03,-46.0625));
#38431=CARTESIAN_POINT('',(2.18941017085715,37.03,-49.3595363724049));
#38432=CARTESIAN_POINT('',(1.26422241896875,37.03,-40.3863290962102));
#38433=CARTESIAN_POINT('',(2.22248159767725,37.03,-49.4152802505257));
#38434=CARTESIAN_POINT('',(1.92399462146588,37.03,-48.9121625074333));
#38435=CARTESIAN_POINT('',(2.57333897421511,37.03,-49.9073260095938));
#38436=CARTESIAN_POINT('',(2.22248159767725,37.03,-49.4152802505257));
#38437=CARTESIAN_POINT('',(2.97207032837233,37.03,-50.3868386222561));
#38438=CARTESIAN_POINT('',(2.57333897421511,37.03,-49.9073260095938));
#38439=CARTESIAN_POINT('',(3.41570362514738,37.03,-50.8521891662412));
#38440=CARTESIAN_POINT('',(2.97207032837233,37.03,-50.3868386222561));
#38441=CARTESIAN_POINT('',(3.90203204952538,37.03,-51.3016633687267));
#38442=CARTESIAN_POINT('',(3.41570362514738,37.03,-50.8521891662412));
#38443=CARTESIAN_POINT('',(4.42926968903682,37.03,-51.7335012750361));
#38444=CARTESIAN_POINT('',(3.90203204952538,37.03,-51.3016633687267));
#38445=CARTESIAN_POINT('',(4.70628452555985,37.03,-51.6658347245569));
#38446=CARTESIAN_POINT('',(4.42926968903682,37.03,-51.7335012750361));
#38447=CARTESIAN_POINT('',(4.98226661822352,37.03,-51.5940721560646));
#38448=CARTESIAN_POINT('',(4.70628452555985,37.03,-51.6658347245569));
#38449=CARTESIAN_POINT('',(5.25715540570603,37.03,-51.518229317088));
#38450=CARTESIAN_POINT('',(4.98226661822352,37.03,-51.5940721560646));
#38451=CARTESIAN_POINT('',(5.53089056659975,37.03,-51.4383228505279));
#38452=CARTESIAN_POINT('',(5.25715540570603,37.03,-51.518229317088));
#38453=CARTESIAN_POINT('',(5.77157280309329,37.03,-50.8007214335911));
#38454=CARTESIAN_POINT('',(5.53089056659975,37.03,-51.4383228505279));
#38455=CARTESIAN_POINT('',(5.96800847194436,37.03,-50.1683011437039));
#38456=CARTESIAN_POINT('',(5.77157280309329,37.03,-50.8007214335911));
#38457=CARTESIAN_POINT('',(6.11953090492363,37.03,-49.5434791025604));
#38458=CARTESIAN_POINT('',(5.96800847194436,37.03,-50.1683011437039));
#38459=CARTESIAN_POINT('',(6.22508608057804,37.03,-48.9288433214812));
#38460=CARTESIAN_POINT('',(6.11953090492363,37.03,-49.5434791025604));
#38461=CARTESIAN_POINT('',(6.2829146022309,37.03,-48.3272905060348));
#38462=CARTESIAN_POINT('',(6.22508608057804,37.03,-48.9288433214812));
#38463=CARTESIAN_POINT('',(6.2836833589361,37.03,-48.2624791780667));
#38464=CARTESIAN_POINT('',(6.2829146022309,37.03,-48.3272905060348));
#38465=CARTESIAN_POINT('',(4.89071476333279,37.03,-45.1503952336939));
#38466=CARTESIAN_POINT('',(2.2119210640689,37.03,-39.1656006819148));
#38467=CARTESIAN_POINT('',(6.53125,37.03,-44.3124568369342));
#38468=CARTESIAN_POINT('',(5.33658159091047,37.03,-44.922659232468));
#38469=CARTESIAN_POINT('',(8.07719355673392,37.03,-43.3106808445568));
#38470=CARTESIAN_POINT('',(6.53125,37.03,-44.3124568369342));
#38471=CARTESIAN_POINT('',(10.0758530134688,37.03,-46.0730690072096));
#38472=CARTESIAN_POINT('',(4.78801327896586,37.03,-38.7646374285458));
#38473=CARTESIAN_POINT('',(10.1323656482948,37.03,-46.1048089083576));
#38474=CARTESIAN_POINT('',(9.62230947265071,37.03,-45.8183396498506));
#38475=CARTESIAN_POINT('',(10.6822399290158,37.03,-46.3555043472661));
#38476=CARTESIAN_POINT('',(10.1323656482948,37.03,-46.1048089083576));
#38477=CARTESIAN_POINT('',(11.2673077173324,37.03,-46.571408774188));
#38478=CARTESIAN_POINT('',(10.6822399290158,37.03,-46.3555043472661));
#38479=CARTESIAN_POINT('',(11.8841806942968,37.03,-46.7525975185565));
#38480=CARTESIAN_POINT('',(11.2673077173324,37.03,-46.571408774188));
#38481=CARTESIAN_POINT('',(12.5300905656334,37.03,-46.8986893840657));
#38482=CARTESIAN_POINT('',(11.8841806942968,37.03,-46.7525975185565));
#38483=CARTESIAN_POINT('',(13.2026107084363,37.03,-47.009053161491));
#38484=CARTESIAN_POINT('',(12.5300905656334,37.03,-46.8986893840657));
#38485=CARTESIAN_POINT('',(13.4086793188509,37.03,-46.8119447915281));
#38486=CARTESIAN_POINT('',(13.2026107084363,37.03,-47.009053161491));
#38487=CARTESIAN_POINT('',(13.611805537841,37.03,-46.6118055378411));
#38488=CARTESIAN_POINT('',(13.4086793188509,37.03,-46.8119447915281));
#38489=CARTESIAN_POINT('',(13.8119447915281,37.03,-46.4086793188509));
#38490=CARTESIAN_POINT('',(13.611805537841,37.03,-46.6118055378411));
#38491=CARTESIAN_POINT('',(14.009053161491,37.03,-46.2026107084364));
#38492=CARTESIAN_POINT('',(13.8119447915281,37.03,-46.4086793188509));
#38493=CARTESIAN_POINT('',(13.8986893840657,37.03,-45.5300905656334));
#38494=CARTESIAN_POINT('',(14.009053161491,37.03,-46.2026107084364));
#38495=CARTESIAN_POINT('',(13.7525975185565,37.03,-44.8841806942968));
#38496=CARTESIAN_POINT('',(13.8986893840657,37.03,-45.5300905656334));
#38497=CARTESIAN_POINT('',(13.571408774188,37.03,-44.2673077173324));
#38498=CARTESIAN_POINT('',(13.7525975185565,37.03,-44.8841806942968));
#38499=CARTESIAN_POINT('',(13.3555043472661,37.03,-43.6822399290158));
#38500=CARTESIAN_POINT('',(13.571408774188,37.03,-44.2673077173324));
#38501=CARTESIAN_POINT('',(13.1048089083576,37.03,-43.1323656482948));
#38502=CARTESIAN_POINT('',(13.3555043472661,37.03,-43.6822399290158));
#38503=CARTESIAN_POINT('',(13.0730690072096,37.03,-43.0758530134688));
#38504=CARTESIAN_POINT('',(13.1048089083576,37.03,-43.1323656482948));
#38505=CARTESIAN_POINT('',(10.3106808445568,37.03,-41.0771935567339));
#38506=CARTESIAN_POINT('',(4.99838017360697,37.03,-37.2336062880944));
#38507=CARTESIAN_POINT('',(11.3124568369342,37.03,-39.53125));
#38508=CARTESIAN_POINT('',(10.5829448433309,37.03,-40.6570349805272));
#38509=CARTESIAN_POINT('',(12.1503952336939,37.03,-37.8907147633328));
#38510=CARTESIAN_POINT('',(11.3124568369342,37.03,-39.53125));
#38511=CARTESIAN_POINT('',(15.2624791780667,37.03,-39.2836833589361));
#38512=CARTESIAN_POINT('',(7.02885984751459,37.03,-35.5983158172444));
#38513=CARTESIAN_POINT('',(15.3272905060348,37.03,-39.2829146022309));
#38514=CARTESIAN_POINT('',(14.7423342713165,37.03,-39.2898530347825));
#38515=CARTESIAN_POINT('',(15.9288433214812,37.03,-39.225086080578));
#38516=CARTESIAN_POINT('',(15.3272905060348,37.03,-39.2829146022309));
#38517=CARTESIAN_POINT('',(16.5434791025604,37.03,-39.1195309049236));
#38518=CARTESIAN_POINT('',(15.9288433214812,37.03,-39.225086080578));
#38519=CARTESIAN_POINT('',(17.1683011437039,37.03,-38.9680084719444));
#38520=CARTESIAN_POINT('',(16.5434791025604,37.03,-39.1195309049236));
#38521=CARTESIAN_POINT('',(17.8007214335911,37.03,-38.7715728030933));
#38522=CARTESIAN_POINT('',(17.1683011437039,37.03,-38.9680084719444));
#38523=CARTESIAN_POINT('',(18.4383228505279,37.03,-38.5308905665998));
#38524=CARTESIAN_POINT('',(17.8007214335911,37.03,-38.7715728030933));
#38525=CARTESIAN_POINT('',(18.518229317088,37.03,-38.257155405706));
#38526=CARTESIAN_POINT('',(18.4383228505279,37.03,-38.5308905665998));
#38527=CARTESIAN_POINT('',(18.5940721560646,37.03,-37.9822666182235));
#38528=CARTESIAN_POINT('',(18.518229317088,37.03,-38.257155405706));
#38529=CARTESIAN_POINT('',(18.6658347245569,37.03,-37.7062845255599));
#38530=CARTESIAN_POINT('',(18.5940721560646,37.03,-37.9822666182235));
#38531=CARTESIAN_POINT('',(18.7335012750361,37.03,-37.4292696890368));
#38532=CARTESIAN_POINT('',(18.6658347245569,37.03,-37.7062845255599));
#38533=CARTESIAN_POINT('',(18.3016633687267,37.03,-36.9020320495254));
#38534=CARTESIAN_POINT('',(18.7335012750361,37.03,-37.4292696890368));
#38535=CARTESIAN_POINT('',(17.8521891662412,37.03,-36.4157036251474));
#38536=CARTESIAN_POINT('',(18.3016633687267,37.03,-36.9020320495254));
#38537=CARTESIAN_POINT('',(17.3868386222561,37.03,-35.9720703283723));
#38538=CARTESIAN_POINT('',(17.8521891662412,37.03,-36.4157036251474));
#38539=CARTESIAN_POINT('',(16.9073260095938,37.03,-35.5733389742151));
#38540=CARTESIAN_POINT('',(17.3868386222561,37.03,-35.9720703283723));
#38541=CARTESIAN_POINT('',(16.4152802505257,37.03,-35.2224815976773));
#38542=CARTESIAN_POINT('',(16.9073260095938,37.03,-35.5733389742151));
#38543=CARTESIAN_POINT('',(16.3595363724049,37.03,-35.1894101708572));
#38544=CARTESIAN_POINT('',(16.4152802505257,37.03,-35.2224815976773));
#38545=CARTESIAN_POINT('',(12.9679083200667,37.03,-34.8397143891372));
#38546=CARTESIAN_POINT('',(6.44552735216333,37.03,-34.1672205083078));
#38547=CARTESIAN_POINT('',(13.0625,37.03,-33.));
#38548=CARTESIAN_POINT('',(12.9936165714376,37.03,-34.3397143891372));
#38549=CARTESIAN_POINT('',(12.9679083200667,37.03,-31.1602856108628));
#38550=CARTESIAN_POINT('',(13.0625,37.03,-33.));
#38551=CARTESIAN_POINT('',(16.3595363724049,37.03,-30.8105898291428));
#38552=CARTESIAN_POINT('',(7.38632909621023,37.03,-31.7357775810312));
#38553=CARTESIAN_POINT('',(16.4152802505257,37.03,-30.7775184023227));
#38554=CARTESIAN_POINT('',(15.9121625074333,37.03,-31.0760053785341));
#38555=CARTESIAN_POINT('',(16.9073260095938,37.03,-30.4266610257849));
#38556=CARTESIAN_POINT('',(16.4152802505257,37.03,-30.7775184023227));
#38557=CARTESIAN_POINT('',(17.3868386222561,37.03,-30.0279296716277));
#38558=CARTESIAN_POINT('',(16.9073260095938,37.03,-30.4266610257849));
#38559=CARTESIAN_POINT('',(17.8521891662412,37.03,-29.5842963748526));
#38560=CARTESIAN_POINT('',(17.3868386222561,37.03,-30.0279296716277));
#38561=CARTESIAN_POINT('',(18.3016633687267,37.03,-29.0979679504746));
#38562=CARTESIAN_POINT('',(17.8521891662412,37.03,-29.5842963748526));
#38563=CARTESIAN_POINT('',(18.7335012750361,37.03,-28.5707303109632));
#38564=CARTESIAN_POINT('',(18.3016633687267,37.03,-29.0979679504746));
#38565=CARTESIAN_POINT('',(18.6658347245569,37.03,-28.2937154744402));
#38566=CARTESIAN_POINT('',(18.7335012750361,37.03,-28.5707303109632));
#38567=CARTESIAN_POINT('',(18.5940721560646,37.03,-28.0177333817765));
#38568=CARTESIAN_POINT('',(18.6658347245569,37.03,-28.2937154744402));
#38569=CARTESIAN_POINT('',(18.518229317088,37.03,-27.742844594294));
#38570=CARTESIAN_POINT('',(18.5940721560646,37.03,-28.0177333817765));
#38571=CARTESIAN_POINT('',(18.4383228505279,37.03,-27.4691094334002));
#38572=CARTESIAN_POINT('',(18.518229317088,37.03,-27.742844594294));
#38573=CARTESIAN_POINT('',(17.8007214335911,37.03,-27.2284271969067));
#38574=CARTESIAN_POINT('',(18.4383228505279,37.03,-27.4691094334002));
#38575=CARTESIAN_POINT('',(17.1683011437039,37.03,-27.0319915280556));
#38576=CARTESIAN_POINT('',(17.8007214335911,37.03,-27.2284271969067));
#38577=CARTESIAN_POINT('',(16.5434791025604,37.03,-26.8804690950764));
#38578=CARTESIAN_POINT('',(17.1683011437039,37.03,-27.0319915280556));
#38579=CARTESIAN_POINT('',(15.9288433214812,37.03,-26.774913919422));
#38580=CARTESIAN_POINT('',(16.5434791025604,37.03,-26.8804690950764));
#38581=CARTESIAN_POINT('',(15.3272905060348,37.03,-26.7170853977691));
#38582=CARTESIAN_POINT('',(15.9288433214812,37.03,-26.774913919422));
#38583=CARTESIAN_POINT('',(15.2624791780667,37.03,-26.7163166410639));
#38584=CARTESIAN_POINT('',(15.3272905060348,37.03,-26.7170853977691));
#38585=CARTESIAN_POINT('',(12.1503952336939,37.03,-28.1092852366672));
#38586=CARTESIAN_POINT('',(6.1656006819148,37.03,-30.7880789359311));
#38587=CARTESIAN_POINT('',(11.922659232468,37.03,-27.6634184090895));
#38588=CARTESIAN_POINT('',(1.04094977927525E-15,37.03,-41.5));
#38589=CARTESIAN_POINT('Origin',(0.,37.03,-33.));
#38590=CARTESIAN_POINT('Origin',(13.1048089083576,37.03,-22.8676343517052));
#38591=CARTESIAN_POINT('',(12.8183396498506,64.7518675845618,-23.3776905273493));
#38592=CARTESIAN_POINT('',(12.8183396498506,37.03,-23.3776905273493));
#38593=CARTESIAN_POINT('',(13.0730690072096,64.97,-22.9241469865312));
#38594=CARTESIAN_POINT('',(8.8979438687676,61.3947146828798,-30.3579232040826));
#38595=CARTESIAN_POINT('',(13.1048089083576,64.97,-22.8676343517052));
#38596=CARTESIAN_POINT('',(12.8183396498506,64.97,-23.3776905273493));
#38597=CARTESIAN_POINT('',(13.1048089083576,37.03,-22.8676343517052));
#38598=CARTESIAN_POINT('Origin',(12.8183396498506,37.03,-23.3776905273493));
#38599=CARTESIAN_POINT('',(12.4929286389212,64.5678155074499,-23.8403088083181));
#38600=CARTESIAN_POINT('',(12.4929286389212,37.03,-23.8403088083181));
#38601=CARTESIAN_POINT('',(8.36376245460559,62.2323640708404,-29.7105089486481));
#38602=CARTESIAN_POINT('Origin',(7.41196956298798,37.28,-31.9844592379009));
#38603=CARTESIAN_POINT('',(15.9121625074333,37.2481324154382,-31.0760053785341));
#38604=CARTESIAN_POINT('',(13.3116513142512,38.5161005118285,-32.6188226083255));
#38605=CARTESIAN_POINT('',(12.9936165714376,37.53,-31.6602856108628));
#38606=CARTESIAN_POINT('',(12.984466051433,37.3520314584495,-31.4823170693123));
#38607=CARTESIAN_POINT('',(14.8752200595314,37.53,-31.466281789541));
#38608=CARTESIAN_POINT('',(7.43761002976572,37.53,-32.2331408947705));
#38609=CARTESIAN_POINT('',(15.3990391648128,37.4321844925501,-31.3139390566435));
#38610=CARTESIAN_POINT('',(11.7907769153056,38.1059743550985,-32.3633328770643));
#38611=CARTESIAN_POINT('',(12.6172283184415,38.429991495039,-32.603855985976));
#38612=CARTESIAN_POINT('Origin',(16.4152802505257,37.03,-30.7775184023227));
#38613=CARTESIAN_POINT('',(15.9121625074333,64.7518675845618,-31.0760053785341));
#38614=CARTESIAN_POINT('',(15.9121625074333,37.03,-31.0760053785341));
#38615=CARTESIAN_POINT('',(16.3595363724049,64.97,-30.8105898291428));
#38616=CARTESIAN_POINT('',(9.0268838297594,61.39471468288,-35.1608663103698));
#38617=CARTESIAN_POINT('',(16.4152802505257,64.97,-30.7775184023227));
#38618=CARTESIAN_POINT('',(15.9121625074333,64.97,-31.0760053785341));
#38619=CARTESIAN_POINT('',(16.4152802505257,37.03,-30.7775184023227));
#38620=CARTESIAN_POINT('Origin',(15.9121625074333,37.03,-31.0760053785341));
#38621=CARTESIAN_POINT('',(15.3990391648128,64.5678155074499,-31.3139390566435));
#38622=CARTESIAN_POINT('',(15.3990391648128,37.03,-31.3139390566435));
#38623=CARTESIAN_POINT('',(8.88797628258284,62.2323640708403,-34.3330984113106));
#38624=CARTESIAN_POINT('Origin',(6.9267243146742,37.28,-35.8265006829375));
#38625=CARTESIAN_POINT('',(14.7423342713165,37.2481324154382,-39.2898530347825));
#38626=CARTESIAN_POINT('',(11.7188169002993,38.5161005118285,-39.3257163525872));
#38627=CARTESIAN_POINT('',(11.922659232468,37.53,-38.3365815909105));
#38628=CARTESIAN_POINT('',(12.0037189204615,37.3520314584495,-38.177881052851));
#38629=CARTESIAN_POINT('',(13.6491775636676,37.53,-39.1093710972614));
#38630=CARTESIAN_POINT('',(6.82458878183381,37.53,-36.0546855486307));
#38631=CARTESIAN_POINT('',(14.1789895822776,37.4321844925501,-39.2393479731309));
#38632=CARTESIAN_POINT('',(10.5294459004776,38.1059743550985,-38.3440185554362));
#38633=CARTESIAN_POINT('',(11.1249122561308,38.429991495039,-38.9655433795188));
#38634=CARTESIAN_POINT('Origin',(15.3272905060348,37.03,-39.2829146022309));
#38635=CARTESIAN_POINT('',(14.7423342713165,64.7518675845618,-39.2898530347825));
#38636=CARTESIAN_POINT('',(14.7423342713165,37.03,-39.2898530347825));
#38637=CARTESIAN_POINT('',(15.2624791780667,64.97,-39.2836833589361));
#38638=CARTESIAN_POINT('',(6.73707755839776,61.3947146828801,-39.3848070338418));
#38639=CARTESIAN_POINT('',(15.3272905060348,64.97,-39.2829146022309));
#38640=CARTESIAN_POINT('',(14.7423342713165,64.97,-39.2898530347825));
#38641=CARTESIAN_POINT('',(15.3272905060348,37.03,-39.2829146022309));
#38642=CARTESIAN_POINT('Origin',(14.7423342713165,37.03,-39.2898530347825));
#38643=CARTESIAN_POINT('',(14.1789895822776,64.5678155074499,-39.2393479731309));
#38644=CARTESIAN_POINT('',(14.1789895822776,37.03,-39.2393479731309));
#38645=CARTESIAN_POINT('',(7.03066404329491,62.2323640708402,-38.5984852312312));
#38646=CARTESIAN_POINT('Origin',(4.58546888005044,37.28,-38.9111835525751));
#38647=CARTESIAN_POINT('',(9.62230947265071,37.2481324154382,-45.8183396498506));
#38648=CARTESIAN_POINT('',(6.98593496166402,38.5161005118286,-44.3376395086249));
#38649=CARTESIAN_POINT('',(7.65703498052716,37.53,-43.5829448433309));
#38650=CARTESIAN_POINT('',(7.80658499858209,37.3520314584495,-43.4860359897738));
#38651=CARTESIAN_POINT('',(8.76584896227005,37.53,-45.1154593532086));
#38652=CARTESIAN_POINT('',(4.38292448113502,37.53,-39.0577296766043));
#38653=CARTESIAN_POINT('',(9.15969119168186,37.4321844925501,-45.4929286389212));
#38654=CARTESIAN_POINT('',(6.44675835986946,38.1059743550985,-42.8927787775419));
#38655=CARTESIAN_POINT('',(6.65168493892267,38.4299914950389,-43.7287682421066));
#38656=CARTESIAN_POINT('Origin',(10.1323656482948,37.03,-46.1048089083576));
#38657=CARTESIAN_POINT('',(9.62230947265071,64.7518675845618,-45.8183396498506));
#38658=CARTESIAN_POINT('',(9.62230947265071,37.03,-45.8183396498506));
#38659=CARTESIAN_POINT('',(10.0758530134688,64.97,-46.0730690072096));
#38660=CARTESIAN_POINT('',(2.64207679591738,61.3947146828798,-41.8979438687676));
#38661=CARTESIAN_POINT('',(10.1323656482948,64.97,-46.1048089083576));
#38662=CARTESIAN_POINT('',(9.62230947265071,64.97,-45.8183396498506));
#38663=CARTESIAN_POINT('',(10.1323656482948,37.03,-46.1048089083576));
#38664=CARTESIAN_POINT('Origin',(9.62230947265071,37.03,-45.8183396498506));
#38665=CARTESIAN_POINT('',(9.15969119168186,64.5678155074499,-45.4929286389212));
#38666=CARTESIAN_POINT('',(9.15969119168186,37.03,-45.4929286389212));
#38667=CARTESIAN_POINT('',(3.2894910513519,62.2323640708404,-41.3637624546056));
#38668=CARTESIAN_POINT('Origin',(1.01554076209913,37.28,-40.411969562988));
#38669=CARTESIAN_POINT('',(1.92399462146588,37.2481324154382,-48.9121625074333));
#38670=CARTESIAN_POINT('',(0.381177391674463,38.5161005118285,-46.3116513142512));
#38671=CARTESIAN_POINT('',(1.33971438913717,37.53,-45.9936165714376));
#38672=CARTESIAN_POINT('',(1.51768293068769,37.3520314584495,-45.9844660514331));
#38673=CARTESIAN_POINT('',(1.53371821045902,37.53,-47.8752200595314));
#38674=CARTESIAN_POINT('',(0.766859105229514,37.53,-40.4376100297657));
#38675=CARTESIAN_POINT('',(1.68606094335647,37.4321844925501,-48.3990391648128));
#38676=CARTESIAN_POINT('',(0.636667122935676,38.1059743550985,-44.7907769153056));
#38677=CARTESIAN_POINT('',(0.396144014024024,38.429991495039,-45.6172283184415));
#38678=CARTESIAN_POINT('Origin',(2.22248159767725,37.03,-49.4152802505257));
#38679=CARTESIAN_POINT('',(1.92399462146588,64.7518675845618,-48.9121625074333));
#38680=CARTESIAN_POINT('',(1.92399462146588,37.03,-48.9121625074333));
#38681=CARTESIAN_POINT('',(2.18941017085715,64.97,-49.3595363724049));
#38682=CARTESIAN_POINT('',(-2.16086631036979,61.39471468288,-42.0268838297594));
#38683=CARTESIAN_POINT('',(2.22248159767725,64.97,-49.4152802505257));
#38684=CARTESIAN_POINT('',(1.92399462146588,64.97,-48.9121625074333));
#38685=CARTESIAN_POINT('',(2.22248159767725,37.03,-49.4152802505257));
#38686=CARTESIAN_POINT('Origin',(1.92399462146588,37.03,-48.9121625074333));
#38687=CARTESIAN_POINT('',(1.68606094335647,64.5678155074499,-48.3990391648128));
#38688=CARTESIAN_POINT('',(1.68606094335647,37.03,-48.3990391648128));
#38689=CARTESIAN_POINT('',(-1.3330984113107,62.2323640708402,-41.8879762825828));
#38690=CARTESIAN_POINT('Origin',(-2.82650068293752,37.28,-39.9267243146742));
#38691=CARTESIAN_POINT('',(-6.28985303478255,37.2481324154382,-47.7423342713165));
#38692=CARTESIAN_POINT('',(-6.32571635258722,38.5161005118285,-44.7188169002993));
#38693=CARTESIAN_POINT('',(-5.33658159091048,37.53,-44.922659232468));
#38694=CARTESIAN_POINT('',(-5.17788105285096,37.3520314584495,-45.0037189204615));
#38695=CARTESIAN_POINT('',(-6.10937109726139,37.53,-46.6491775636676));
#38696=CARTESIAN_POINT('',(-3.05468554863069,37.53,-39.8245887818338));
#38697=CARTESIAN_POINT('',(-6.23934797313094,37.4321844925501,-47.1789895822776));
#38698=CARTESIAN_POINT('',(-5.34401855543615,38.1059743550985,-43.5294459004776));
#38699=CARTESIAN_POINT('',(-5.96554337951879,38.429991495039,-44.1249122561308));
#38700=CARTESIAN_POINT('Origin',(-6.2829146022309,37.03,-48.3272905060348));
#38701=CARTESIAN_POINT('',(-6.28985303478255,64.7518675845618,-47.7423342713165));
#38702=CARTESIAN_POINT('',(-6.28985303478255,37.03,-47.7423342713165));
#38703=CARTESIAN_POINT('',(-6.2836833589361,64.97,-48.2624791780667));
#38704=CARTESIAN_POINT('',(-6.38480703384186,61.39471468288,-39.7370775583977));
#38705=CARTESIAN_POINT('',(-6.2829146022309,64.97,-48.3272905060348));
#38706=CARTESIAN_POINT('',(-6.28985303478255,64.97,-47.7423342713165));
#38707=CARTESIAN_POINT('',(-6.2829146022309,37.03,-48.3272905060348));
#38708=CARTESIAN_POINT('Origin',(-6.28985303478255,37.03,-47.7423342713165));
#38709=CARTESIAN_POINT('',(-6.23934797313094,64.5678155074499,-47.1789895822776));
#38710=CARTESIAN_POINT('',(-6.23934797313094,37.03,-47.1789895822776));
#38711=CARTESIAN_POINT('',(-5.59848523123113,62.2323640708402,-40.030664043295));
#38712=CARTESIAN_POINT('Origin',(-5.91118355257507,37.28,-37.5854688800504));
#38713=CARTESIAN_POINT('',(-12.8183396498506,37.2481324154382,-42.6223094726507));
#38714=CARTESIAN_POINT('',(-11.3376395086248,38.5161005118285,-39.985934961664));
#38715=CARTESIAN_POINT('',(-10.5829448433309,37.53,-40.6570349805272));
#38716=CARTESIAN_POINT('',(-10.4860359897738,37.3520314584495,-40.8065849985821));
#38717=CARTESIAN_POINT('',(-12.1154593532086,37.53,-41.76584896227));
#38718=CARTESIAN_POINT('',(-6.0577296766043,37.53,-37.382924481135));
#38719=CARTESIAN_POINT('',(-12.4929286389212,37.4321844925501,-42.1596911916819));
#38720=CARTESIAN_POINT('',(-9.89277877754201,38.1059743550986,-39.4467583598694));
#38721=CARTESIAN_POINT('',(-10.7287682421066,38.4299914950389,-39.6516849389227));
#38722=CARTESIAN_POINT('Origin',(-13.1048089083576,37.03,-43.1323656482948));
#38723=CARTESIAN_POINT('',(-12.8183396498506,64.7518675845618,-42.6223094726507));
#38724=CARTESIAN_POINT('',(-12.8183396498506,37.03,-42.6223094726507));
#38725=CARTESIAN_POINT('',(-13.0730690072096,64.97,-43.0758530134688));
#38726=CARTESIAN_POINT('',(-8.89794386876747,61.3947146828801,-35.6420767959176));
#38727=CARTESIAN_POINT('',(-13.1048089083576,64.97,-43.1323656482948));
#38728=CARTESIAN_POINT('',(-12.8183396498506,64.97,-42.6223094726507));
#38729=CARTESIAN_POINT('',(-13.1048089083576,37.03,-43.1323656482948));
#38730=CARTESIAN_POINT('Origin',(-12.8183396498506,37.03,-42.6223094726507));
#38731=CARTESIAN_POINT('',(-12.4929286389212,64.5678155074499,-42.1596911916819));
#38732=CARTESIAN_POINT('',(-12.4929286389212,37.03,-42.1596911916819));
#38733=CARTESIAN_POINT('',(-8.36376245460558,62.2323640708405,-36.289491051352));
#38734=CARTESIAN_POINT('Origin',(-7.41196956298797,37.28,-34.0155407620991));
#38735=CARTESIAN_POINT('',(-15.9121625074333,37.2481324154382,-34.9239946214659));
#38736=CARTESIAN_POINT('',(-13.3116513142512,38.5161005118285,-33.3811773916745));
#38737=CARTESIAN_POINT('',(-12.9936165714376,37.53,-34.3397143891372));
#38738=CARTESIAN_POINT('',(-12.984466051433,37.3520314584495,-34.5176829306877));
#38739=CARTESIAN_POINT('',(-14.8752200595314,37.53,-34.533718210459));
#38740=CARTESIAN_POINT('',(-7.43761002976572,37.53,-33.7668591052295));
#38741=CARTESIAN_POINT('',(-15.3990391648128,37.4321844925501,-34.6860609433565));
#38742=CARTESIAN_POINT('',(-11.7907769153057,38.1059743550986,-33.6366671229356));
#38743=CARTESIAN_POINT('',(-12.6172283184414,38.4299914950389,-33.3961440140241));
#38744=CARTESIAN_POINT('Origin',(-16.4152802505257,37.03,-35.2224815976773));
#38745=CARTESIAN_POINT('',(-15.9121625074333,64.7518675845618,-34.9239946214659));
#38746=CARTESIAN_POINT('',(-15.9121625074333,37.03,-34.9239946214659));
#38747=CARTESIAN_POINT('',(-16.3595363724049,64.97,-35.1894101708572));
#38748=CARTESIAN_POINT('',(-9.0268838297594,61.3947146828801,-30.8391336896303));
#38749=CARTESIAN_POINT('',(-16.4152802505257,64.97,-35.2224815976773));
#38750=CARTESIAN_POINT('',(-15.9121625074333,64.97,-34.9239946214659));
#38751=CARTESIAN_POINT('',(-16.4152802505257,37.03,-35.2224815976773));
#38752=CARTESIAN_POINT('Origin',(-15.9121625074333,37.03,-34.9239946214659));
#38753=CARTESIAN_POINT('',(-15.3990391648128,64.5678155074499,-34.6860609433565));
#38754=CARTESIAN_POINT('',(-15.3990391648128,37.03,-34.6860609433565));
#38755=CARTESIAN_POINT('',(-8.88797628258289,62.2323640708405,-31.6669015886896));
#38756=CARTESIAN_POINT('Origin',(-6.9267243146742,37.28,-30.1734993170625));
#38757=CARTESIAN_POINT('',(-14.7423342713164,37.2481324154382,-26.7101469652174));
#38758=CARTESIAN_POINT('',(-11.7188169002993,38.5161005118285,-26.6742836474128));
#38759=CARTESIAN_POINT('',(-11.922659232468,37.53,-27.6634184090895));
#38760=CARTESIAN_POINT('',(-12.0037189204615,37.3520314584495,-27.822118947149));
#38761=CARTESIAN_POINT('',(-13.6491775636676,37.53,-26.8906289027386));
#38762=CARTESIAN_POINT('',(-6.8245887818338,37.53,-29.9453144513693));
#38763=CARTESIAN_POINT('',(-14.1789895822776,37.4321844925501,-26.7606520268691));
#38764=CARTESIAN_POINT('',(-10.5294459004776,38.1059743550986,-27.6559814445638));
#38765=CARTESIAN_POINT('',(-11.1249122561307,38.4299914950389,-27.0344566204813));
#38766=CARTESIAN_POINT('Origin',(-15.3272905060348,37.03,-26.7170853977691));
#38767=CARTESIAN_POINT('',(-14.7423342713164,64.7518675845618,-26.7101469652174));
#38768=CARTESIAN_POINT('',(-14.7423342713164,37.03,-26.7101469652174));
#38769=CARTESIAN_POINT('',(-15.2624791780667,64.97,-26.7163166410639));
#38770=CARTESIAN_POINT('',(-6.73707755839773,61.39471468288,-26.6151929661581));
#38771=CARTESIAN_POINT('',(-15.3272905060348,64.97,-26.7170853977691));
#38772=CARTESIAN_POINT('',(-14.7423342713164,64.97,-26.7101469652174));
#38773=CARTESIAN_POINT('',(-15.3272905060348,37.03,-26.7170853977691));
#38774=CARTESIAN_POINT('Origin',(-14.7423342713164,37.03,-26.7101469652174));
#38775=CARTESIAN_POINT('',(-14.1789895822776,64.5678155074499,-26.7606520268691));
#38776=CARTESIAN_POINT('',(-14.1789895822776,37.03,-26.7606520268691));
#38777=CARTESIAN_POINT('',(-7.03066404329514,62.2323640708404,-27.401514768769));
#38778=CARTESIAN_POINT('Origin',(-4.58546888005044,37.28,-27.0888164474249));
#38779=CARTESIAN_POINT('',(-9.62230947265072,37.2481324154382,-20.1816603501494));
#38780=CARTESIAN_POINT('',(-6.98593496166398,38.5161005118285,-21.6623604913752));
#38781=CARTESIAN_POINT('',(-7.65703498052716,37.53,-22.4170551566691));
#38782=CARTESIAN_POINT('',(-7.80658499858209,37.3520314584495,-22.5139640102262));
#38783=CARTESIAN_POINT('',(-8.76584896227005,37.53,-20.8845406467914));
#38784=CARTESIAN_POINT('',(-4.38292448113502,37.53,-26.9422703233957));
#38785=CARTESIAN_POINT('',(-9.15969119168187,37.4321844925501,-20.5070713610788));
#38786=CARTESIAN_POINT('',(-6.44675835986946,38.1059743550986,-23.107221222458));
#38787=CARTESIAN_POINT('',(-6.65168493892268,38.4299914950389,-22.2712317578934));
#38788=CARTESIAN_POINT('Origin',(-10.1323656482948,37.03,-19.8951910916424));
#38789=CARTESIAN_POINT('',(-9.62230947265072,64.7518675845618,-20.1816603501494));
#38790=CARTESIAN_POINT('',(-9.62230947265072,37.03,-20.1816603501494));
#38791=CARTESIAN_POINT('',(-10.0758530134688,64.97,-19.9269309927904));
#38792=CARTESIAN_POINT('',(-2.64207679591758,61.39471468288,-24.1020561312325));
#38793=CARTESIAN_POINT('',(-10.1323656482948,64.97,-19.8951910916424));
#38794=CARTESIAN_POINT('',(-9.62230947265072,64.97,-20.1816603501494));
#38795=CARTESIAN_POINT('',(-10.1323656482948,37.03,-19.8951910916424));
#38796=CARTESIAN_POINT('Origin',(-9.62230947265072,37.03,-20.1816603501494));
#38797=CARTESIAN_POINT('',(-9.15969119168187,64.5678155074499,-20.5070713610788));
#38798=CARTESIAN_POINT('',(-9.15969119168187,37.03,-20.5070713610788));
#38799=CARTESIAN_POINT('',(-3.28949105135187,62.2323640708404,-24.6362375453944));
#38800=CARTESIAN_POINT('Origin',(-1.01554076209914,37.28,-25.588030437012));
#38801=CARTESIAN_POINT('',(-1.92399462146589,37.2481324154382,-17.0878374925667));
#38802=CARTESIAN_POINT('',(-0.381177391674473,38.5161005118285,-19.6883486857488));
#38803=CARTESIAN_POINT('',(-1.33971438913717,37.53,-20.0063834285624));
#38804=CARTESIAN_POINT('',(-1.5176829306877,37.3520314584495,-20.015533948567));
#38805=CARTESIAN_POINT('',(-1.53371821045904,37.53,-18.1247799404686));
#38806=CARTESIAN_POINT('',(-0.766859105229518,37.53,-25.5623899702343));
#38807=CARTESIAN_POINT('',(-1.68606094335648,37.4321844925501,-17.6009608351872));
#38808=CARTESIAN_POINT('',(-0.6366671229357,38.1059743550985,-21.2092230846944));
#38809=CARTESIAN_POINT('',(-0.396144014024061,38.4299914950389,-20.3827716815586));
#38810=CARTESIAN_POINT('Origin',(-2.22248159767725,37.03,-16.5847197494743));
#38811=CARTESIAN_POINT('',(-1.92399462146589,64.7518675845618,-17.0878374925667));
#38812=CARTESIAN_POINT('',(-1.92399462146589,37.03,-17.0878374925667));
#38813=CARTESIAN_POINT('',(-2.18941017085717,64.97,-16.6404636275951));
#38814=CARTESIAN_POINT('',(2.16086631036976,61.39471468288,-23.9731161702406));
#38815=CARTESIAN_POINT('',(-2.22248159767725,64.97,-16.5847197494743));
#38816=CARTESIAN_POINT('',(-1.92399462146589,64.97,-17.0878374925667));
#38817=CARTESIAN_POINT('',(-2.22248159767725,37.03,-16.5847197494743));
#38818=CARTESIAN_POINT('Origin',(-1.92399462146589,37.03,-17.0878374925667));
#38819=CARTESIAN_POINT('',(-1.68606094335648,64.5678155074499,-17.6009608351872));
#38820=CARTESIAN_POINT('',(-1.68606094335648,37.03,-17.6009608351872));
#38821=CARTESIAN_POINT('',(1.33309841131053,62.2323640708404,-24.1120237174171));
#38822=CARTESIAN_POINT('Origin',(2.82650068293752,37.28,-26.0732756853258));
#38823=CARTESIAN_POINT('',(6.28985303478256,37.2481324154382,-18.2576657286835));
#38824=CARTESIAN_POINT('',(6.32571635258722,38.5161005118285,-21.2811830997007));
#38825=CARTESIAN_POINT('',(5.33658159091048,37.53,-21.077340767532));
#38826=CARTESIAN_POINT('',(5.17788105285096,37.3520314584495,-20.9962810795385));
#38827=CARTESIAN_POINT('',(6.10937109726139,37.53,-19.3508224363324));
#38828=CARTESIAN_POINT('',(3.05468554863069,37.53,-26.1754112181662));
#38829=CARTESIAN_POINT('',(6.23934797313093,37.4321844925501,-18.8210104177224));
#38830=CARTESIAN_POINT('',(5.34401855543614,38.1059743550985,-22.4705540995224));
#38831=CARTESIAN_POINT('',(5.96554337951873,38.4299914950389,-21.8750877438693));
#38832=CARTESIAN_POINT('Origin',(6.28291460223091,37.03,-17.6727094939652));
#38833=CARTESIAN_POINT('',(6.28985303478256,64.7518675845618,-18.2576657286835));
#38834=CARTESIAN_POINT('',(6.28985303478256,37.03,-18.2576657286835));
#38835=CARTESIAN_POINT('',(6.28368335893611,64.97,-17.7375208219333));
#38836=CARTESIAN_POINT('',(6.38480703384186,61.39471468288,-26.2629224416023));
#38837=CARTESIAN_POINT('',(6.28291460223091,64.97,-17.6727094939652));
#38838=CARTESIAN_POINT('',(6.28985303478256,64.97,-18.2576657286835));
#38839=CARTESIAN_POINT('',(6.28291460223091,37.03,-17.6727094939652));
#38840=CARTESIAN_POINT('Origin',(6.28985303478256,37.03,-18.2576657286835));
#38841=CARTESIAN_POINT('',(6.23934797313093,64.5678155074499,-18.8210104177224));
#38842=CARTESIAN_POINT('',(6.23934797313093,37.03,-18.8210104177224));
#38843=CARTESIAN_POINT('',(5.59848523123102,62.2323640708404,-25.9693359567049));
#38844=CARTESIAN_POINT('Origin',(4.03106188917902,37.28,-27.8550737023638));
#38845=CARTESIAN_POINT('',(9.15969119168187,37.4321844925501,-20.5070713610788));
#38846=CARTESIAN_POINT('',(8.76584896227005,37.53,-20.8845406467914));
#38847=CARTESIAN_POINT('',(5.93055826671154,38.2341789260846,-23.6019616690071));
#38848=CARTESIAN_POINT('',(7.65703498052716,37.53,-22.4170551566691));
#38849=CARTESIAN_POINT('',(3.82851749026359,37.53,-27.7085275783346));
#38850=CARTESIAN_POINT('',(7.51456472435969,37.6995434345929,-22.3247340097329));
#38851=CARTESIAN_POINT('',(9.62230947265072,37.2481324154382,-20.1816603501494));
#38852=CARTESIAN_POINT('',(6.45071205345202,38.7735167359811,-21.9629644581006));
#38853=CARTESIAN_POINT('',(6.11180584490169,38.6447816854218,-22.6509889118845));
#38854=CARTESIAN_POINT('Origin',(7.65703498052716,37.03,-22.4170551566691));
#38855=CARTESIAN_POINT('',(8.76584896227005,64.47,-20.8845406467914));
#38856=CARTESIAN_POINT('',(8.76584896227005,37.03,-20.8845406467914));
#38857=CARTESIAN_POINT('',(7.65703498052716,64.47,-22.4170551566691));
#38858=CARTESIAN_POINT('',(3.82851749026359,64.47,-27.7085275783346));
#38859=CARTESIAN_POINT('',(7.65703498052716,37.03,-22.4170551566691));
#38860=CARTESIAN_POINT('Origin',(8.76584896227005,37.03,-20.8845406467914));
#38861=CARTESIAN_POINT('',(9.15969119168187,64.5678155074499,-20.5070713610788));
#38862=CARTESIAN_POINT('',(9.15969119168187,37.03,-20.5070713610788));
#38863=CARTESIAN_POINT('',(4.17846180539155,63.3306666093445,-25.2812193777137));
#38864=CARTESIAN_POINT('Origin',(6.06346514907441,37.28,-30.5598940702379));
#38865=CARTESIAN_POINT('',(14.1789895822776,37.4321844925501,-26.7606520268691));
#38866=CARTESIAN_POINT('',(13.6491775636676,37.53,-26.8906289027386));
#38867=CARTESIAN_POINT('',(9.83503328309243,38.2341789260845,-27.8263391929761));
#38868=CARTESIAN_POINT('',(11.922659232468,37.53,-27.6634184090895));
#38869=CARTESIAN_POINT('',(5.96132961623402,37.53,-30.3317092045448));
#38870=CARTESIAN_POINT('',(11.8454369448115,37.6995434345929,-27.5122308224524));
#38871=CARTESIAN_POINT('',(14.7423342713165,37.2481324154382,-26.7101469652175));
#38872=CARTESIAN_POINT('',(11.1049982817376,38.773516735981,-26.6670028649695));
#38873=CARTESIAN_POINT('',(10.4674846687408,38.6447816854218,-27.093396416096));
#38874=CARTESIAN_POINT('Origin',(11.922659232468,37.03,-27.6634184090895));
#38875=CARTESIAN_POINT('',(13.6491775636676,64.47,-26.8906289027386));
#38876=CARTESIAN_POINT('',(13.6491775636676,37.03,-26.8906289027386));
#38877=CARTESIAN_POINT('',(11.922659232468,64.47,-27.6634184090895));
#38878=CARTESIAN_POINT('',(5.96132961623402,64.47,-30.3317092045448));
#38879=CARTESIAN_POINT('',(11.922659232468,37.03,-27.6634184090895));
#38880=CARTESIAN_POINT('Origin',(13.6491775636676,37.03,-26.8906289027386));
#38881=CARTESIAN_POINT('',(14.1789895822776,64.5678155074499,-26.7606520268691));
#38882=CARTESIAN_POINT('',(14.1789895822776,37.03,-26.7606520268691));
#38883=CARTESIAN_POINT('',(7.47804438335529,63.3306666093445,-28.4045707975568));
#38884=CARTESIAN_POINT('Origin',(6.47116781894107,37.28,-33.9185388514382));
#38885=CARTESIAN_POINT('',(15.3990391648128,37.4321844925501,-34.6860609433565));
#38886=CARTESIAN_POINT('',(14.8752200595314,37.53,-34.533718210459));
#38887=CARTESIAN_POINT('',(11.1042190737355,38.2341789260845,-33.4369949520996));
#38888=CARTESIAN_POINT('',(12.9936165714376,37.53,-34.3397143891372));
#38889=CARTESIAN_POINT('',(6.49680828571882,37.53,-33.6698571945686));
#38890=CARTESIAN_POINT('',(13.0023339019072,37.6995434345929,-34.1701709545443));
#38891=CARTESIAN_POINT('',(15.9121625074333,37.2481324154382,-34.9239946214659));
#38892=CARTESIAN_POINT('',(12.7837091884825,38.773516735981,-33.0679627398383));
#38893=CARTESIAN_POINT('',(12.0184094288058,38.6447816854218,-33.1184735806253));
#38894=CARTESIAN_POINT('Origin',(12.9936165714376,37.03,-34.3397143891372));
#38895=CARTESIAN_POINT('',(14.8752200595314,64.47,-34.533718210459));
#38896=CARTESIAN_POINT('',(14.8752200595314,37.03,-34.533718210459));
#38897=CARTESIAN_POINT('',(12.9936165714376,64.47,-34.3397143891372));
#38898=CARTESIAN_POINT('',(6.49680828571882,64.47,-33.6698571945686));
#38899=CARTESIAN_POINT('',(12.9936165714376,37.03,-34.3397143891372));
#38900=CARTESIAN_POINT('Origin',(14.8752200595314,37.03,-34.533718210459));
#38901=CARTESIAN_POINT('',(15.3990391648128,64.5678155074499,-34.6860609433565));
#38902=CARTESIAN_POINT('',(15.3990391648128,37.03,-34.6860609433565));
#38903=CARTESIAN_POINT('',(8.77389100783484,63.3306666093446,-32.759263761069));
#38904=CARTESIAN_POINT('Origin',(5.1449262976362,37.28,-37.031061889179));
#38905=CARTESIAN_POINT('',(12.4929286389212,37.4321844925501,-42.1596911916819));
#38906=CARTESIAN_POINT('',(12.1154593532086,37.53,-41.76584896227));
#38907=CARTESIAN_POINT('',(9.39803833099293,38.2341789260846,-38.9305582667115));
#38908=CARTESIAN_POINT('',(10.5829448433309,37.53,-40.6570349805272));
#38909=CARTESIAN_POINT('',(5.29147242166543,37.53,-36.8285174902636));
#38910=CARTESIAN_POINT('',(10.6752659902672,37.6995434345929,-40.5145647243597));
#38911=CARTESIAN_POINT('',(12.8183396498506,37.2481324154382,-42.6223094726507));
#38912=CARTESIAN_POINT('',(11.0370355418994,38.7735167359811,-39.450712053452));
#38913=CARTESIAN_POINT('',(10.3490110881154,38.6447816854217,-39.1118058449017));
#38914=CARTESIAN_POINT('Origin',(10.5829448433309,37.03,-40.6570349805272));
#38915=CARTESIAN_POINT('',(12.1154593532086,64.47,-41.76584896227));
#38916=CARTESIAN_POINT('',(12.1154593532086,37.03,-41.76584896227));
#38917=CARTESIAN_POINT('',(10.5829448433309,64.47,-40.6570349805272));
#38918=CARTESIAN_POINT('',(5.29147242166543,64.47,-36.8285174902636));
#38919=CARTESIAN_POINT('',(10.5829448433309,37.03,-40.6570349805272));
#38920=CARTESIAN_POINT('Origin',(12.1154593532086,37.03,-41.76584896227));
#38921=CARTESIAN_POINT('',(12.4929286389212,64.5678155074499,-42.1596911916819));
#38922=CARTESIAN_POINT('',(12.4929286389212,37.03,-42.1596911916819));
#38923=CARTESIAN_POINT('',(7.71878062228625,63.3306666093444,-37.1784618053914));
#38924=CARTESIAN_POINT('Origin',(2.44010592976207,37.28,-39.0634651490744));
#38925=CARTESIAN_POINT('',(6.23934797313093,37.4321844925501,-47.1789895822776));
#38926=CARTESIAN_POINT('',(6.10937109726138,37.53,-46.6491775636676));
#38927=CARTESIAN_POINT('',(5.17366080702395,38.2341789260845,-42.8350332830924));
#38928=CARTESIAN_POINT('',(5.33658159091047,37.53,-44.922659232468));
#38929=CARTESIAN_POINT('',(2.66829079545524,37.53,-38.961329616234));
#38930=CARTESIAN_POINT('',(5.48776917754755,37.6995434345929,-44.8454369448115));
#38931=CARTESIAN_POINT('',(6.28985303478254,37.2481324154382,-47.7423342713165));
#38932=CARTESIAN_POINT('',(6.33299713503051,38.773516735981,-44.1049982817375));
#38933=CARTESIAN_POINT('',(5.90660358390404,38.6447816854218,-43.4674846687409));
#38934=CARTESIAN_POINT('Origin',(5.33658159091047,37.03,-44.922659232468));
#38935=CARTESIAN_POINT('',(6.10937109726138,64.47,-46.6491775636676));
#38936=CARTESIAN_POINT('',(6.10937109726138,37.03,-46.6491775636676));
#38937=CARTESIAN_POINT('',(5.33658159091047,64.47,-44.922659232468));
#38938=CARTESIAN_POINT('',(2.66829079545524,64.47,-38.961329616234));
#38939=CARTESIAN_POINT('',(5.33658159091047,37.03,-44.922659232468));
#38940=CARTESIAN_POINT('Origin',(6.10937109726138,37.03,-46.6491775636676));
#38941=CARTESIAN_POINT('',(6.23934797313093,64.5678155074499,-47.1789895822776));
#38942=CARTESIAN_POINT('',(6.23934797313093,37.03,-47.1789895822776));
#38943=CARTESIAN_POINT('',(4.5954292024432,63.3306666093445,-40.4780443833553));
#38944=CARTESIAN_POINT('Origin',(-0.918538851438202,37.28,-39.4711678189411));
#38945=CARTESIAN_POINT('',(-1.68606094335648,37.4321844925501,-48.3990391648128));
#38946=CARTESIAN_POINT('',(-1.53371821045903,37.53,-47.8752200595314));
#38947=CARTESIAN_POINT('',(-0.436994952099579,38.2341789260845,-44.1042190737355));
#38948=CARTESIAN_POINT('',(-1.33971438913717,37.53,-45.9936165714376));
#38949=CARTESIAN_POINT('',(-0.669857194568582,37.53,-39.4968082857188));
#38950=CARTESIAN_POINT('',(-1.17017095454431,37.6995434345929,-46.0023339019072));
#38951=CARTESIAN_POINT('',(-1.92399462146589,37.2481324154382,-48.9121625074333));
#38952=CARTESIAN_POINT('',(-0.0679627398382643,38.773516735981,-45.7837091884825));
#38953=CARTESIAN_POINT('',(-0.118473580625308,38.6447816854218,-45.0184094288058));
#38954=CARTESIAN_POINT('Origin',(-1.33971438913717,37.03,-45.9936165714376));
#38955=CARTESIAN_POINT('',(-1.53371821045903,64.47,-47.8752200595314));
#38956=CARTESIAN_POINT('',(-1.53371821045903,37.03,-47.8752200595314));
#38957=CARTESIAN_POINT('',(-1.33971438913717,64.47,-45.9936165714376));
#38958=CARTESIAN_POINT('',(-0.669857194568582,64.47,-39.4968082857188));
#38959=CARTESIAN_POINT('',(-1.33971438913717,37.03,-45.9936165714376));
#38960=CARTESIAN_POINT('Origin',(-1.53371821045903,37.03,-47.8752200595314));
#38961=CARTESIAN_POINT('',(-1.68606094335648,64.5678155074499,-48.3990391648128));
#38962=CARTESIAN_POINT('',(-1.68606094335648,37.03,-48.3990391648128));
#38963=CARTESIAN_POINT('',(0.240736238931031,63.3306666093445,-41.7738910078348));
#38964=CARTESIAN_POINT('Origin',(-4.03106188917902,37.28,-38.1449262976362));
#38965=CARTESIAN_POINT('',(-9.15969119168187,37.4321844925501,-45.4929286389212));
#38966=CARTESIAN_POINT('',(-8.76584896227005,37.53,-45.1154593532086));
#38967=CARTESIAN_POINT('',(-5.93055826671154,38.2341789260845,-42.3980383309929));
#38968=CARTESIAN_POINT('',(-7.65703498052716,37.53,-43.5829448433309));
#38969=CARTESIAN_POINT('',(-3.82851749026359,37.53,-38.2914724216654));
#38970=CARTESIAN_POINT('',(-7.51456472435969,37.6995434345929,-43.6752659902671));
#38971=CARTESIAN_POINT('',(-9.62230947265071,37.2481324154382,-45.8183396498506));
#38972=CARTESIAN_POINT('',(-6.45071205345204,38.7735167359811,-44.0370355418994));
#38973=CARTESIAN_POINT('',(-6.11180584490168,38.6447816854217,-43.3490110881154));
#38974=CARTESIAN_POINT('Origin',(-7.65703498052716,37.03,-43.5829448433309));
#38975=CARTESIAN_POINT('',(-8.76584896227005,64.47,-45.1154593532086));
#38976=CARTESIAN_POINT('',(-8.76584896227005,37.03,-45.1154593532086));
#38977=CARTESIAN_POINT('',(-7.65703498052716,64.47,-43.5829448433309));
#38978=CARTESIAN_POINT('',(-3.82851749026359,64.47,-38.2914724216654));
#38979=CARTESIAN_POINT('',(-7.65703498052716,37.03,-43.5829448433309));
#38980=CARTESIAN_POINT('Origin',(-8.76584896227005,37.03,-45.1154593532086));
#38981=CARTESIAN_POINT('',(-9.15969119168187,64.5678155074499,-45.4929286389212));
#38982=CARTESIAN_POINT('',(-9.15969119168187,37.03,-45.4929286389212));
#38983=CARTESIAN_POINT('',(-4.17846180539157,63.3306666093445,-40.7187806222863));
#38984=CARTESIAN_POINT('Origin',(-6.06346514907441,37.28,-35.4401059297621));
#38985=CARTESIAN_POINT('',(-14.1789895822776,37.4321844925501,-39.2393479731309));
#38986=CARTESIAN_POINT('',(-13.6491775636676,37.53,-39.1093710972614));
#38987=CARTESIAN_POINT('',(-9.83503328309245,38.2341789260846,-38.173660807024));
#38988=CARTESIAN_POINT('',(-11.922659232468,37.53,-38.3365815909105));
#38989=CARTESIAN_POINT('',(-5.96132961623402,37.53,-35.6682907954552));
#38990=CARTESIAN_POINT('',(-11.8454369448115,37.6995434345929,-38.4877691775476));
#38991=CARTESIAN_POINT('',(-14.7423342713165,37.2481324154382,-39.2898530347826));
#38992=CARTESIAN_POINT('',(-11.1049982817375,38.773516735981,-39.3329971350305));
#38993=CARTESIAN_POINT('',(-10.4674846687408,38.6447816854218,-38.906603583904));
#38994=CARTESIAN_POINT('Origin',(-11.922659232468,37.03,-38.3365815909105));
#38995=CARTESIAN_POINT('',(-13.6491775636676,64.47,-39.1093710972614));
#38996=CARTESIAN_POINT('',(-13.6491775636676,37.03,-39.1093710972614));
#38997=CARTESIAN_POINT('',(-11.922659232468,64.47,-38.3365815909105));
#38998=CARTESIAN_POINT('',(-5.96132961623402,64.47,-35.6682907954552));
#38999=CARTESIAN_POINT('',(-11.922659232468,37.03,-38.3365815909105));
#39000=CARTESIAN_POINT('Origin',(-13.6491775636676,37.03,-39.1093710972614));
#39001=CARTESIAN_POINT('',(-14.1789895822776,64.5678155074499,-39.2393479731309));
#39002=CARTESIAN_POINT('',(-14.1789895822776,37.03,-39.2393479731309));
#39003=CARTESIAN_POINT('',(-7.47804438335517,63.3306666093444,-37.5954292024432));
#39004=CARTESIAN_POINT('Origin',(-6.47116781894107,37.28,-32.0814611485618));
#39005=CARTESIAN_POINT('',(-15.3990391648128,37.4321844925501,-31.3139390566435));
#39006=CARTESIAN_POINT('',(-14.8752200595314,37.53,-31.466281789541));
#39007=CARTESIAN_POINT('',(-11.1042190737355,38.2341789260846,-32.5630050479005));
#39008=CARTESIAN_POINT('',(-12.9936165714376,37.53,-31.6602856108628));
#39009=CARTESIAN_POINT('',(-6.49680828571882,37.53,-32.3301428054314));
#39010=CARTESIAN_POINT('',(-13.0023339019072,37.6995434345929,-31.8298290454557));
#39011=CARTESIAN_POINT('',(-15.9121625074333,37.2481324154382,-31.0760053785341));
#39012=CARTESIAN_POINT('',(-12.7837091884825,38.773516735981,-32.9320372601617));
#39013=CARTESIAN_POINT('',(-12.0184094288057,38.6447816854217,-32.8815264193746));
#39014=CARTESIAN_POINT('Origin',(-12.9936165714376,37.03,-31.6602856108628));
#39015=CARTESIAN_POINT('',(-14.8752200595314,64.47,-31.466281789541));
#39016=CARTESIAN_POINT('',(-14.8752200595314,37.03,-31.466281789541));
#39017=CARTESIAN_POINT('',(-12.9936165714376,64.47,-31.6602856108628));
#39018=CARTESIAN_POINT('',(-6.49680828571882,64.47,-32.3301428054314));
#39019=CARTESIAN_POINT('',(-12.9936165714376,37.03,-31.6602856108628));
#39020=CARTESIAN_POINT('Origin',(-14.8752200595314,37.03,-31.466281789541));
#39021=CARTESIAN_POINT('',(-15.3990391648128,64.5678155074499,-31.3139390566435));
#39022=CARTESIAN_POINT('',(-15.3990391648128,37.03,-31.3139390566435));
#39023=CARTESIAN_POINT('',(-8.77389100783466,63.3306666093444,-33.2407362389312));
#39024=CARTESIAN_POINT('Origin',(-5.14492629763621,37.28,-28.968938110821));
#39025=CARTESIAN_POINT('',(-12.4929286389212,37.4321844925501,-23.8403088083181));
#39026=CARTESIAN_POINT('',(-12.1154593532086,37.53,-24.23415103773));
#39027=CARTESIAN_POINT('',(-9.39803833099287,38.2341789260845,-27.0694417332885));
#39028=CARTESIAN_POINT('',(-10.5829448433309,37.53,-25.3429650194728));
#39029=CARTESIAN_POINT('',(-5.29147242166544,37.53,-29.1714825097364));
#39030=CARTESIAN_POINT('',(-10.6752659902672,37.6995434345929,-25.4854352756403));
#39031=CARTESIAN_POINT('',(-12.8183396498506,37.2481324154382,-23.3776905273493));
#39032=CARTESIAN_POINT('',(-11.0370355418993,38.773516735981,-26.549287946548));
#39033=CARTESIAN_POINT('',(-10.3490110881154,38.6447816854218,-26.8881941550983));
#39034=CARTESIAN_POINT('Origin',(-10.5829448433309,37.03,-25.3429650194728));
#39035=CARTESIAN_POINT('',(-12.1154593532086,64.47,-24.23415103773));
#39036=CARTESIAN_POINT('',(-12.1154593532086,37.03,-24.23415103773));
#39037=CARTESIAN_POINT('',(-10.5829448433309,64.47,-25.3429650194728));
#39038=CARTESIAN_POINT('',(-5.29147242166544,64.47,-29.1714825097364));
#39039=CARTESIAN_POINT('',(-10.5829448433309,37.03,-25.3429650194728));
#39040=CARTESIAN_POINT('Origin',(-12.1154593532086,37.03,-24.23415103773));
#39041=CARTESIAN_POINT('',(-12.4929286389212,64.5678155074499,-23.8403088083181));
#39042=CARTESIAN_POINT('',(-12.4929286389212,37.03,-23.8403088083181));
#39043=CARTESIAN_POINT('',(-7.7187806222863,63.3306666093445,-28.8215381946084));
#39044=CARTESIAN_POINT('Origin',(-2.44010592976206,37.28,-26.9365348509256));
#39045=CARTESIAN_POINT('',(-6.23934797313094,37.4321844925501,-18.8210104177224));
#39046=CARTESIAN_POINT('',(-6.10937109726139,37.53,-19.3508224363324));
#39047=CARTESIAN_POINT('',(-5.17366080702394,38.2341789260845,-23.1649667169076));
#39048=CARTESIAN_POINT('',(-5.33658159091048,37.53,-21.077340767532));
#39049=CARTESIAN_POINT('',(-2.66829079545523,37.53,-27.038670383766));
#39050=CARTESIAN_POINT('',(-5.48776917754756,37.6995434345929,-21.1545630551885));
#39051=CARTESIAN_POINT('',(-6.28985303478256,37.2481324154382,-18.2576657286835));
#39052=CARTESIAN_POINT('',(-6.33299713503051,38.773516735981,-21.8950017182625));
#39053=CARTESIAN_POINT('',(-5.90660358390399,38.6447816854218,-22.5325153312592));
#39054=CARTESIAN_POINT('Origin',(-5.33658159091048,37.03,-21.077340767532));
#39055=CARTESIAN_POINT('',(-6.10937109726139,64.47,-19.3508224363324));
#39056=CARTESIAN_POINT('',(-6.10937109726139,37.03,-19.3508224363324));
#39057=CARTESIAN_POINT('',(-5.33658159091048,64.47,-21.077340767532));
#39058=CARTESIAN_POINT('',(-2.66829079545523,64.47,-27.038670383766));
#39059=CARTESIAN_POINT('',(-5.33658159091048,37.03,-21.077340767532));
#39060=CARTESIAN_POINT('Origin',(-6.10937109726139,37.03,-19.3508224363324));
#39061=CARTESIAN_POINT('',(-6.23934797313094,64.5678155074499,-18.8210104177224));
#39062=CARTESIAN_POINT('',(-6.23934797313094,37.03,-18.8210104177224));
#39063=CARTESIAN_POINT('',(-4.59542920244319,63.3306666093445,-25.5219556166447));
#39064=CARTESIAN_POINT('Origin',(0.918538851438207,37.28,-26.5288321810589));
#39065=CARTESIAN_POINT('',(1.68606094335648,37.4321844925501,-17.6009608351872));
#39066=CARTESIAN_POINT('',(1.53371821045903,37.53,-18.1247799404686));
#39067=CARTESIAN_POINT('',(0.43699495209958,38.2341789260845,-21.8957809262645));
#39068=CARTESIAN_POINT('',(1.33971438913717,37.53,-20.0063834285624));
#39069=CARTESIAN_POINT('',(0.669857194568587,37.53,-26.5031917142812));
#39070=CARTESIAN_POINT('',(1.17017095454432,37.6995434345929,-19.9976660980928));
#39071=CARTESIAN_POINT('',(1.92399462146589,37.2481324154382,-17.0878374925667));
#39072=CARTESIAN_POINT('',(0.0679627398382635,38.773516735981,-20.2162908115175));
#39073=CARTESIAN_POINT('',(0.118473580625342,38.6447816854218,-20.9815905711943));
#39074=CARTESIAN_POINT('Origin',(1.33971438913717,37.03,-20.0063834285624));
#39075=CARTESIAN_POINT('',(1.53371821045903,64.47,-18.1247799404686));
#39076=CARTESIAN_POINT('',(1.53371821045903,37.03,-18.1247799404686));
#39077=CARTESIAN_POINT('',(1.33971438913717,64.47,-20.0063834285624));
#39078=CARTESIAN_POINT('',(0.669857194568587,64.47,-26.5031917142812));
#39079=CARTESIAN_POINT('',(1.33971438913717,37.03,-20.0063834285624));
#39080=CARTESIAN_POINT('Origin',(1.53371821045903,37.03,-18.1247799404686));
#39081=CARTESIAN_POINT('',(1.68606094335648,64.5678155074499,-17.6009608351872));
#39082=CARTESIAN_POINT('',(1.68606094335648,37.03,-17.6009608351872));
#39083=CARTESIAN_POINT('',(-0.240736238931032,63.3306666093445,-24.2261089921652));
#39084=CARTESIAN_POINT('Origin',(2.82650068293752,64.72,-26.0732756853258));
#39085=CARTESIAN_POINT('',(6.10937109726139,64.47,-19.3508224363324));
#39086=CARTESIAN_POINT('',(4.76578695085538,63.4588711803305,-24.8275429992595));
#39087=CARTESIAN_POINT('',(5.33658159091048,64.47,-21.077340767532));
#39088=CARTESIAN_POINT('',(3.05468554863069,64.47,-26.1754112181662));
#39089=CARTESIAN_POINT('',(4.8907147633328,64.97,-20.8496047663061));
#39090=CARTESIAN_POINT('',(11.3984181516531,57.6721893244721,-24.173553208203));
#39091=CARTESIAN_POINT('',(2.59831581724435,64.97,-25.9711401524854));
#39092=CARTESIAN_POINT('Origin',(2.22044604925031E-15,64.97,-33.));
#39093=CARTESIAN_POINT('',(6.53125,64.97,-21.6875431630658));
#39094=CARTESIAN_POINT('',(6.53125,64.97,-21.6875431630658));
#39095=CARTESIAN_POINT('',(8.07719355673392,64.97,-22.6893191554432));
#39096=CARTESIAN_POINT('',(7.65703498052716,64.97,-22.4170551566691));
#39097=CARTESIAN_POINT('',(10.0758530134688,64.97,-19.9269309927904));
#39098=CARTESIAN_POINT('',(4.23360628809444,64.97,-28.001619826393));
#39099=CARTESIAN_POINT('',(10.1323656482948,64.97,-19.8951910916424));
#39100=CARTESIAN_POINT('',(10.1323656482948,64.97,-19.8951910916424));
#39101=CARTESIAN_POINT('',(10.6822399290158,64.97,-19.6444956527339));
#39102=CARTESIAN_POINT('',(10.6822399290158,64.97,-19.6444956527339));
#39103=CARTESIAN_POINT('',(11.2673077173324,64.97,-19.428591225812));
#39104=CARTESIAN_POINT('',(11.2673077173324,64.97,-19.428591225812));
#39105=CARTESIAN_POINT('',(11.8841806942968,64.97,-19.2474024814435));
#39106=CARTESIAN_POINT('',(11.8841806942968,64.97,-19.2474024814435));
#39107=CARTESIAN_POINT('',(12.5300905656334,64.97,-19.1013106159343));
#39108=CARTESIAN_POINT('',(12.5300905656334,64.97,-19.1013106159343));
#39109=CARTESIAN_POINT('',(13.2026107084364,64.97,-18.990946838509));
#39110=CARTESIAN_POINT('',(13.2026107084364,64.97,-18.990946838509));
#39111=CARTESIAN_POINT('',(13.4086793188509,64.97,-19.1880552084719));
#39112=CARTESIAN_POINT('',(13.4086793188509,64.97,-19.1880552084719));
#39113=CARTESIAN_POINT('',(13.611805537841,64.97,-19.388194462159));
#39114=CARTESIAN_POINT('',(13.611805537841,64.97,-19.388194462159));
#39115=CARTESIAN_POINT('',(13.8119447915281,64.97,-19.5913206811491));
#39116=CARTESIAN_POINT('',(13.8119447915281,64.97,-19.5913206811491));
#39117=CARTESIAN_POINT('',(14.009053161491,64.97,-19.7973892915637));
#39118=CARTESIAN_POINT('',(14.009053161491,64.97,-19.7973892915637));
#39119=CARTESIAN_POINT('',(13.8986893840657,64.97,-20.4699094343666));
#39120=CARTESIAN_POINT('',(13.8986893840657,64.97,-20.4699094343666));
#39121=CARTESIAN_POINT('',(13.7525975185565,64.97,-21.1158193057032));
#39122=CARTESIAN_POINT('',(13.7525975185565,64.97,-21.1158193057032));
#39123=CARTESIAN_POINT('',(13.571408774188,64.97,-21.7326922826676));
#39124=CARTESIAN_POINT('',(13.571408774188,64.97,-21.7326922826676));
#39125=CARTESIAN_POINT('',(13.3555043472661,64.97,-22.3177600709842));
#39126=CARTESIAN_POINT('',(13.3555043472661,64.97,-22.3177600709842));
#39127=CARTESIAN_POINT('',(13.1048089083576,64.97,-22.8676343517052));
#39128=CARTESIAN_POINT('',(10.3106808445568,64.97,-24.9228064432661));
#39129=CARTESIAN_POINT('',(5.76463742854583,64.97,-28.2119867210341));
#39130=CARTESIAN_POINT('',(11.3124568369342,64.97,-26.46875));
#39131=CARTESIAN_POINT('',(11.3124568369342,64.97,-26.46875));
#39132=CARTESIAN_POINT('',(12.1503952336939,64.97,-28.1092852366672));
#39133=CARTESIAN_POINT('',(11.922659232468,64.97,-27.6634184090895));
#39134=CARTESIAN_POINT('',(15.2624791780667,64.97,-26.7163166410639));
#39135=CARTESIAN_POINT('',(6.1656006819148,64.97,-30.7880789359311));
#39136=CARTESIAN_POINT('',(15.3272905060348,64.97,-26.7170853977691));
#39137=CARTESIAN_POINT('',(15.3272905060348,64.97,-26.7170853977691));
#39138=CARTESIAN_POINT('',(15.9288433214812,64.97,-26.774913919422));
#39139=CARTESIAN_POINT('',(15.9288433214812,64.97,-26.774913919422));
#39140=CARTESIAN_POINT('',(16.5434791025604,64.97,-26.8804690950764));
#39141=CARTESIAN_POINT('',(16.5434791025604,64.97,-26.8804690950764));
#39142=CARTESIAN_POINT('',(17.1683011437039,64.97,-27.0319915280556));
#39143=CARTESIAN_POINT('',(17.1683011437039,64.97,-27.0319915280556));
#39144=CARTESIAN_POINT('',(17.8007214335911,64.97,-27.2284271969067));
#39145=CARTESIAN_POINT('',(17.8007214335911,64.97,-27.2284271969067));
#39146=CARTESIAN_POINT('',(18.4383228505279,64.97,-27.4691094334002));
#39147=CARTESIAN_POINT('',(18.4383228505279,64.97,-27.4691094334002));
#39148=CARTESIAN_POINT('',(18.518229317088,64.97,-27.742844594294));
#39149=CARTESIAN_POINT('',(18.518229317088,64.97,-27.742844594294));
#39150=CARTESIAN_POINT('',(18.5940721560646,64.97,-28.0177333817765));
#39151=CARTESIAN_POINT('',(18.5940721560646,64.97,-28.0177333817765));
#39152=CARTESIAN_POINT('',(18.6658347245569,64.97,-28.2937154744402));
#39153=CARTESIAN_POINT('',(18.6658347245569,64.97,-28.2937154744402));
#39154=CARTESIAN_POINT('',(18.7335012750361,64.97,-28.5707303109632));
#39155=CARTESIAN_POINT('',(18.7335012750361,64.97,-28.5707303109632));
#39156=CARTESIAN_POINT('',(18.3016633687267,64.97,-29.0979679504746));
#39157=CARTESIAN_POINT('',(18.3016633687267,64.97,-29.0979679504746));
#39158=CARTESIAN_POINT('',(17.8521891662412,64.97,-29.5842963748526));
#39159=CARTESIAN_POINT('',(17.8521891662412,64.97,-29.5842963748526));
#39160=CARTESIAN_POINT('',(17.3868386222561,64.97,-30.0279296716277));
#39161=CARTESIAN_POINT('',(17.3868386222561,64.97,-30.0279296716277));
#39162=CARTESIAN_POINT('',(16.9073260095938,64.97,-30.4266610257849));
#39163=CARTESIAN_POINT('',(16.9073260095938,64.97,-30.4266610257849));
#39164=CARTESIAN_POINT('',(16.4152802505257,64.97,-30.7775184023227));
#39165=CARTESIAN_POINT('',(12.9679083200667,64.97,-31.1602856108628));
#39166=CARTESIAN_POINT('',(7.38632909621023,64.97,-31.7357775810312));
#39167=CARTESIAN_POINT('',(13.0625,64.97,-33.));
#39168=CARTESIAN_POINT('',(13.0625,64.97,-33.));
#39169=CARTESIAN_POINT('',(12.9679083200667,64.97,-34.8397143891372));
#39170=CARTESIAN_POINT('',(12.9936165714376,64.97,-34.3397143891372));
#39171=CARTESIAN_POINT('',(16.3595363724049,64.97,-35.1894101708572));
#39172=CARTESIAN_POINT('',(6.44552735216333,64.97,-34.1672205083078));
#39173=CARTESIAN_POINT('',(16.4152802505257,64.97,-35.2224815976773));
#39174=CARTESIAN_POINT('',(16.4152802505257,64.97,-35.2224815976773));
#39175=CARTESIAN_POINT('',(16.9073260095938,64.97,-35.5733389742151));
#39176=CARTESIAN_POINT('',(16.9073260095938,64.97,-35.5733389742151));
#39177=CARTESIAN_POINT('',(17.3868386222561,64.97,-35.9720703283723));
#39178=CARTESIAN_POINT('',(17.3868386222561,64.97,-35.9720703283723));
#39179=CARTESIAN_POINT('',(17.8521891662412,64.97,-36.4157036251474));
#39180=CARTESIAN_POINT('',(17.8521891662412,64.97,-36.4157036251474));
#39181=CARTESIAN_POINT('',(18.3016633687267,64.97,-36.9020320495254));
#39182=CARTESIAN_POINT('',(18.3016633687267,64.97,-36.9020320495254));
#39183=CARTESIAN_POINT('',(18.7335012750361,64.97,-37.4292696890368));
#39184=CARTESIAN_POINT('',(18.7335012750361,64.97,-37.4292696890368));
#39185=CARTESIAN_POINT('',(18.6658347245569,64.97,-37.7062845255599));
#39186=CARTESIAN_POINT('',(18.6658347245569,64.97,-37.7062845255599));
#39187=CARTESIAN_POINT('',(18.5940721560646,64.97,-37.9822666182235));
#39188=CARTESIAN_POINT('',(18.5940721560646,64.97,-37.9822666182235));
#39189=CARTESIAN_POINT('',(18.518229317088,64.97,-38.257155405706));
#39190=CARTESIAN_POINT('',(18.518229317088,64.97,-38.257155405706));
#39191=CARTESIAN_POINT('',(18.4383228505279,64.97,-38.5308905665998));
#39192=CARTESIAN_POINT('',(18.4383228505279,64.97,-38.5308905665998));
#39193=CARTESIAN_POINT('',(17.8007214335911,64.97,-38.7715728030933));
#39194=CARTESIAN_POINT('',(17.8007214335911,64.97,-38.7715728030933));
#39195=CARTESIAN_POINT('',(17.1683011437039,64.97,-38.9680084719444));
#39196=CARTESIAN_POINT('',(17.1683011437039,64.97,-38.9680084719444));
#39197=CARTESIAN_POINT('',(16.5434791025604,64.97,-39.1195309049236));
#39198=CARTESIAN_POINT('',(16.5434791025604,64.97,-39.1195309049236));
#39199=CARTESIAN_POINT('',(15.9288433214812,64.97,-39.225086080578));
#39200=CARTESIAN_POINT('',(15.9288433214812,64.97,-39.225086080578));
#39201=CARTESIAN_POINT('',(15.3272905060348,64.97,-39.2829146022309));
#39202=CARTESIAN_POINT('',(12.1503952336939,64.97,-37.8907147633328));
#39203=CARTESIAN_POINT('',(7.02885984751459,64.97,-35.5983158172444));
#39204=CARTESIAN_POINT('',(11.3124568369342,64.97,-39.53125));
#39205=CARTESIAN_POINT('',(11.3124568369342,64.97,-39.53125));
#39206=CARTESIAN_POINT('',(10.3106808445568,64.97,-41.0771935567339));
#39207=CARTESIAN_POINT('',(10.5829448433309,64.97,-40.6570349805272));
#39208=CARTESIAN_POINT('',(13.0730690072096,64.97,-43.0758530134688));
#39209=CARTESIAN_POINT('',(4.99838017360697,64.97,-37.2336062880944));
#39210=CARTESIAN_POINT('',(13.1048089083576,64.97,-43.1323656482948));
#39211=CARTESIAN_POINT('',(13.1048089083576,64.97,-43.1323656482948));
#39212=CARTESIAN_POINT('',(13.3555043472661,64.97,-43.6822399290158));
#39213=CARTESIAN_POINT('',(13.3555043472661,64.97,-43.6822399290158));
#39214=CARTESIAN_POINT('',(13.571408774188,64.97,-44.2673077173324));
#39215=CARTESIAN_POINT('',(13.571408774188,64.97,-44.2673077173324));
#39216=CARTESIAN_POINT('',(13.7525975185565,64.97,-44.8841806942968));
#39217=CARTESIAN_POINT('',(13.7525975185565,64.97,-44.8841806942968));
#39218=CARTESIAN_POINT('',(13.8986893840657,64.97,-45.5300905656334));
#39219=CARTESIAN_POINT('',(13.8986893840657,64.97,-45.5300905656334));
#39220=CARTESIAN_POINT('',(14.009053161491,64.97,-46.2026107084364));
#39221=CARTESIAN_POINT('',(14.009053161491,64.97,-46.2026107084364));
#39222=CARTESIAN_POINT('',(13.8119447915281,64.97,-46.4086793188509));
#39223=CARTESIAN_POINT('',(13.8119447915281,64.97,-46.4086793188509));
#39224=CARTESIAN_POINT('',(13.611805537841,64.97,-46.6118055378411));
#39225=CARTESIAN_POINT('',(13.611805537841,64.97,-46.6118055378411));
#39226=CARTESIAN_POINT('',(13.4086793188509,64.97,-46.8119447915281));
#39227=CARTESIAN_POINT('',(13.4086793188509,64.97,-46.8119447915281));
#39228=CARTESIAN_POINT('',(13.2026107084363,64.97,-47.009053161491));
#39229=CARTESIAN_POINT('',(13.2026107084363,64.97,-47.009053161491));
#39230=CARTESIAN_POINT('',(12.5300905656334,64.97,-46.8986893840657));
#39231=CARTESIAN_POINT('',(12.5300905656334,64.97,-46.8986893840657));
#39232=CARTESIAN_POINT('',(11.8841806942968,64.97,-46.7525975185565));
#39233=CARTESIAN_POINT('',(11.8841806942968,64.97,-46.7525975185565));
#39234=CARTESIAN_POINT('',(11.2673077173324,64.97,-46.571408774188));
#39235=CARTESIAN_POINT('',(11.2673077173324,64.97,-46.571408774188));
#39236=CARTESIAN_POINT('',(10.6822399290158,64.97,-46.3555043472661));
#39237=CARTESIAN_POINT('',(10.6822399290158,64.97,-46.3555043472661));
#39238=CARTESIAN_POINT('',(10.1323656482948,64.97,-46.1048089083576));
#39239=CARTESIAN_POINT('',(8.07719355673392,64.97,-43.3106808445568));
#39240=CARTESIAN_POINT('',(4.78801327896586,64.97,-38.7646374285458));
#39241=CARTESIAN_POINT('',(6.53125,64.97,-44.3124568369342));
#39242=CARTESIAN_POINT('',(6.53125,64.97,-44.3124568369342));
#39243=CARTESIAN_POINT('',(4.89071476333279,64.97,-45.1503952336939));
#39244=CARTESIAN_POINT('',(5.33658159091047,64.97,-44.922659232468));
#39245=CARTESIAN_POINT('',(6.2836833589361,64.97,-48.2624791780667));
#39246=CARTESIAN_POINT('',(2.2119210640689,64.97,-39.1656006819148));
#39247=CARTESIAN_POINT('',(6.2829146022309,64.97,-48.3272905060348));
#39248=CARTESIAN_POINT('',(6.2829146022309,64.97,-48.3272905060348));
#39249=CARTESIAN_POINT('',(6.22508608057804,64.97,-48.9288433214812));
#39250=CARTESIAN_POINT('',(6.22508608057804,64.97,-48.9288433214812));
#39251=CARTESIAN_POINT('',(6.11953090492363,64.97,-49.5434791025604));
#39252=CARTESIAN_POINT('',(6.11953090492363,64.97,-49.5434791025604));
#39253=CARTESIAN_POINT('',(5.96800847194436,64.97,-50.1683011437039));
#39254=CARTESIAN_POINT('',(5.96800847194436,64.97,-50.1683011437039));
#39255=CARTESIAN_POINT('',(5.77157280309329,64.97,-50.8007214335911));
#39256=CARTESIAN_POINT('',(5.77157280309329,64.97,-50.8007214335911));
#39257=CARTESIAN_POINT('',(5.53089056659975,64.97,-51.4383228505279));
#39258=CARTESIAN_POINT('',(5.53089056659975,64.97,-51.4383228505279));
#39259=CARTESIAN_POINT('',(5.25715540570603,64.97,-51.518229317088));
#39260=CARTESIAN_POINT('',(5.25715540570603,64.97,-51.518229317088));
#39261=CARTESIAN_POINT('',(4.98226661822352,64.97,-51.5940721560646));
#39262=CARTESIAN_POINT('',(4.98226661822352,64.97,-51.5940721560646));
#39263=CARTESIAN_POINT('',(4.70628452555985,64.97,-51.6658347245569));
#39264=CARTESIAN_POINT('',(4.70628452555985,64.97,-51.6658347245569));
#39265=CARTESIAN_POINT('',(4.42926968903682,64.97,-51.7335012750361));
#39266=CARTESIAN_POINT('',(4.42926968903682,64.97,-51.7335012750361));
#39267=CARTESIAN_POINT('',(3.90203204952538,64.97,-51.3016633687267));
#39268=CARTESIAN_POINT('',(3.90203204952538,64.97,-51.3016633687267));
#39269=CARTESIAN_POINT('',(3.41570362514738,64.97,-50.8521891662412));
#39270=CARTESIAN_POINT('',(3.41570362514738,64.97,-50.8521891662412));
#39271=CARTESIAN_POINT('',(2.97207032837233,64.97,-50.3868386222561));
#39272=CARTESIAN_POINT('',(2.97207032837233,64.97,-50.3868386222561));
#39273=CARTESIAN_POINT('',(2.57333897421511,64.97,-49.9073260095938));
#39274=CARTESIAN_POINT('',(2.57333897421511,64.97,-49.9073260095938));
#39275=CARTESIAN_POINT('',(2.22248159767725,64.97,-49.4152802505257));
#39276=CARTESIAN_POINT('',(1.83971438913716,64.97,-45.9679083200667));
#39277=CARTESIAN_POINT('',(1.26422241896875,64.97,-40.3863290962102));
#39278=CARTESIAN_POINT('',(-2.22044604925031E-15,64.97,-46.0625));
#39279=CARTESIAN_POINT('',(-2.39954232207934E-15,64.97,-46.0625));
#39280=CARTESIAN_POINT('',(-1.83971438913717,64.97,-45.9679083200667));
#39281=CARTESIAN_POINT('',(-1.33971438913717,64.97,-45.9936165714376));
#39282=CARTESIAN_POINT('',(-2.18941017085716,64.97,-49.3595363724049));
#39283=CARTESIAN_POINT('',(-1.16722050830782,64.97,-39.4455273521633));
#39284=CARTESIAN_POINT('',(-2.22248159767726,64.97,-49.4152802505257));
#39285=CARTESIAN_POINT('',(-2.22248159767726,64.97,-49.4152802505257));
#39286=CARTESIAN_POINT('',(-2.57333897421511,64.97,-49.9073260095938));
#39287=CARTESIAN_POINT('',(-2.57333897421511,64.97,-49.9073260095938));
#39288=CARTESIAN_POINT('',(-2.97207032837233,64.97,-50.3868386222561));
#39289=CARTESIAN_POINT('',(-2.97207032837234,64.97,-50.3868386222561));
#39290=CARTESIAN_POINT('',(-3.41570362514738,64.97,-50.8521891662412));
#39291=CARTESIAN_POINT('',(-3.41570362514739,64.97,-50.8521891662412));
#39292=CARTESIAN_POINT('',(-3.90203204952539,64.97,-51.3016633687267));
#39293=CARTESIAN_POINT('',(-3.90203204952539,64.97,-51.3016633687267));
#39294=CARTESIAN_POINT('',(-4.42926968903682,64.97,-51.7335012750361));
#39295=CARTESIAN_POINT('',(-4.42926968903682,64.97,-51.7335012750361));
#39296=CARTESIAN_POINT('',(-4.70628452555985,64.97,-51.6658347245569));
#39297=CARTESIAN_POINT('',(-4.70628452555985,64.97,-51.6658347245569));
#39298=CARTESIAN_POINT('',(-4.98226661822352,64.97,-51.5940721560646));
#39299=CARTESIAN_POINT('',(-4.98226661822352,64.97,-51.5940721560646));
#39300=CARTESIAN_POINT('',(-5.25715540570604,64.97,-51.518229317088));
#39301=CARTESIAN_POINT('',(-5.25715540570604,64.97,-51.518229317088));
#39302=CARTESIAN_POINT('',(-5.53089056659976,64.97,-51.4383228505279));
#39303=CARTESIAN_POINT('',(-5.53089056659976,64.97,-51.4383228505279));
#39304=CARTESIAN_POINT('',(-5.7715728030933,64.97,-50.8007214335911));
#39305=CARTESIAN_POINT('',(-5.7715728030933,64.97,-50.8007214335911));
#39306=CARTESIAN_POINT('',(-5.96800847194436,64.97,-50.1683011437039));
#39307=CARTESIAN_POINT('',(-5.96800847194436,64.97,-50.1683011437039));
#39308=CARTESIAN_POINT('',(-6.11953090492364,64.97,-49.5434791025604));
#39309=CARTESIAN_POINT('',(-6.11953090492364,64.97,-49.5434791025604));
#39310=CARTESIAN_POINT('',(-6.22508608057804,64.97,-48.9288433214812));
#39311=CARTESIAN_POINT('',(-6.22508608057804,64.97,-48.9288433214812));
#39312=CARTESIAN_POINT('',(-6.2829146022309,64.97,-48.3272905060348));
#39313=CARTESIAN_POINT('',(-4.8907147633328,64.97,-45.1503952336939));
#39314=CARTESIAN_POINT('',(-2.59831581724436,64.97,-40.0288598475146));
#39315=CARTESIAN_POINT('',(-6.53125000000001,64.97,-44.3124568369342));
#39316=CARTESIAN_POINT('',(-6.53125000000001,64.97,-44.3124568369342));
#39317=CARTESIAN_POINT('',(-8.07719355673392,64.97,-43.3106808445568));
#39318=CARTESIAN_POINT('',(-7.65703498052716,64.97,-43.5829448433309));
#39319=CARTESIAN_POINT('',(-10.0758530134688,64.97,-46.0730690072096));
#39320=CARTESIAN_POINT('',(-4.23360628809444,64.97,-37.998380173607));
#39321=CARTESIAN_POINT('',(-10.1323656482948,64.97,-46.1048089083576));
#39322=CARTESIAN_POINT('',(-10.1323656482948,64.97,-46.1048089083576));
#39323=CARTESIAN_POINT('',(-10.6822399290158,64.97,-46.3555043472661));
#39324=CARTESIAN_POINT('',(-10.6822399290158,64.97,-46.3555043472661));
#39325=CARTESIAN_POINT('',(-11.2673077173324,64.97,-46.571408774188));
#39326=CARTESIAN_POINT('',(-11.2673077173324,64.97,-46.571408774188));
#39327=CARTESIAN_POINT('',(-11.8841806942968,64.97,-46.7525975185565));
#39328=CARTESIAN_POINT('',(-11.8841806942968,64.97,-46.7525975185565));
#39329=CARTESIAN_POINT('',(-12.5300905656334,64.97,-46.8986893840657));
#39330=CARTESIAN_POINT('',(-12.5300905656334,64.97,-46.8986893840657));
#39331=CARTESIAN_POINT('',(-13.2026107084363,64.97,-47.009053161491));
#39332=CARTESIAN_POINT('',(-13.2026107084363,64.97,-47.009053161491));
#39333=CARTESIAN_POINT('',(-13.4086793188509,64.97,-46.8119447915281));
#39334=CARTESIAN_POINT('',(-13.4086793188509,64.97,-46.8119447915281));
#39335=CARTESIAN_POINT('',(-13.611805537841,64.97,-46.611805537841));
#39336=CARTESIAN_POINT('',(-13.611805537841,64.97,-46.611805537841));
#39337=CARTESIAN_POINT('',(-13.8119447915281,64.97,-46.4086793188509));
#39338=CARTESIAN_POINT('',(-13.8119447915281,64.97,-46.4086793188509));
#39339=CARTESIAN_POINT('',(-14.009053161491,64.97,-46.2026107084363));
#39340=CARTESIAN_POINT('',(-14.009053161491,64.97,-46.2026107084363));
#39341=CARTESIAN_POINT('',(-13.8986893840657,64.97,-45.5300905656334));
#39342=CARTESIAN_POINT('',(-13.8986893840657,64.97,-45.5300905656334));
#39343=CARTESIAN_POINT('',(-13.7525975185565,64.97,-44.8841806942968));
#39344=CARTESIAN_POINT('',(-13.7525975185565,64.97,-44.8841806942968));
#39345=CARTESIAN_POINT('',(-13.571408774188,64.97,-44.2673077173324));
#39346=CARTESIAN_POINT('',(-13.571408774188,64.97,-44.2673077173324));
#39347=CARTESIAN_POINT('',(-13.3555043472661,64.97,-43.6822399290158));
#39348=CARTESIAN_POINT('',(-13.3555043472661,64.97,-43.6822399290158));
#39349=CARTESIAN_POINT('',(-13.1048089083576,64.97,-43.1323656482948));
#39350=CARTESIAN_POINT('',(-10.3106808445568,64.97,-41.0771935567339));
#39351=CARTESIAN_POINT('',(-5.76463742854584,64.97,-37.7880132789659));
#39352=CARTESIAN_POINT('',(-11.3124568369342,64.97,-39.53125));
#39353=CARTESIAN_POINT('',(-11.3124568369342,64.97,-39.53125));
#39354=CARTESIAN_POINT('',(-12.1503952336939,64.97,-37.8907147633328));
#39355=CARTESIAN_POINT('',(-11.922659232468,64.97,-38.3365815909105));
#39356=CARTESIAN_POINT('',(-15.2624791780667,64.97,-39.2836833589361));
#39357=CARTESIAN_POINT('',(-6.16560068191481,64.97,-35.2119210640689));
#39358=CARTESIAN_POINT('',(-15.3272905060348,64.97,-39.2829146022309));
#39359=CARTESIAN_POINT('',(-15.3272905060348,64.97,-39.2829146022309));
#39360=CARTESIAN_POINT('',(-15.9288433214812,64.97,-39.225086080578));
#39361=CARTESIAN_POINT('',(-15.9288433214812,64.97,-39.225086080578));
#39362=CARTESIAN_POINT('',(-16.5434791025604,64.97,-39.1195309049236));
#39363=CARTESIAN_POINT('',(-16.5434791025604,64.97,-39.1195309049236));
#39364=CARTESIAN_POINT('',(-17.1683011437039,64.97,-38.9680084719444));
#39365=CARTESIAN_POINT('',(-17.1683011437039,64.97,-38.9680084719444));
#39366=CARTESIAN_POINT('',(-17.8007214335911,64.97,-38.7715728030933));
#39367=CARTESIAN_POINT('',(-17.8007214335911,64.97,-38.7715728030933));
#39368=CARTESIAN_POINT('',(-18.4383228505279,64.97,-38.5308905665998));
#39369=CARTESIAN_POINT('',(-18.4383228505279,64.97,-38.5308905665998));
#39370=CARTESIAN_POINT('',(-18.518229317088,64.97,-38.257155405706));
#39371=CARTESIAN_POINT('',(-18.518229317088,64.97,-38.257155405706));
#39372=CARTESIAN_POINT('',(-18.5940721560646,64.97,-37.9822666182235));
#39373=CARTESIAN_POINT('',(-18.5940721560646,64.97,-37.9822666182235));
#39374=CARTESIAN_POINT('',(-18.6658347245569,64.97,-37.7062845255599));
#39375=CARTESIAN_POINT('',(-18.6658347245569,64.97,-37.7062845255599));
#39376=CARTESIAN_POINT('',(-18.7335012750361,64.97,-37.4292696890368));
#39377=CARTESIAN_POINT('',(-18.7335012750361,64.97,-37.4292696890368));
#39378=CARTESIAN_POINT('',(-18.3016633687267,64.97,-36.9020320495254));
#39379=CARTESIAN_POINT('',(-18.3016633687267,64.97,-36.9020320495254));
#39380=CARTESIAN_POINT('',(-17.8521891662412,64.97,-36.4157036251474));
#39381=CARTESIAN_POINT('',(-17.8521891662412,64.97,-36.4157036251474));
#39382=CARTESIAN_POINT('',(-17.3868386222561,64.97,-35.9720703283723));
#39383=CARTESIAN_POINT('',(-17.3868386222561,64.97,-35.9720703283723));
#39384=CARTESIAN_POINT('',(-16.9073260095938,64.97,-35.5733389742151));
#39385=CARTESIAN_POINT('',(-16.9073260095938,64.97,-35.5733389742151));
#39386=CARTESIAN_POINT('',(-16.4152802505257,64.97,-35.2224815976773));
#39387=CARTESIAN_POINT('',(-12.9679083200667,64.97,-34.8397143891372));
#39388=CARTESIAN_POINT('',(-7.38632909621023,64.97,-34.2642224189688));
#39389=CARTESIAN_POINT('',(-13.0625,64.97,-33.));
#39390=CARTESIAN_POINT('',(-13.0625,64.97,-33.));
#39391=CARTESIAN_POINT('',(-12.9679083200667,64.97,-31.1602856108628));
#39392=CARTESIAN_POINT('',(-12.9936165714376,64.97,-31.6602856108628));
#39393=CARTESIAN_POINT('',(-16.3595363724049,64.97,-30.8105898291428));
#39394=CARTESIAN_POINT('',(-6.44552735216333,64.97,-31.8327794916922));
#39395=CARTESIAN_POINT('',(-16.4152802505257,64.97,-30.7775184023227));
#39396=CARTESIAN_POINT('',(-16.4152802505257,64.97,-30.7775184023227));
#39397=CARTESIAN_POINT('',(-16.9073260095938,64.97,-30.4266610257849));
#39398=CARTESIAN_POINT('',(-16.9073260095938,64.97,-30.4266610257849));
#39399=CARTESIAN_POINT('',(-17.3868386222561,64.97,-30.0279296716277));
#39400=CARTESIAN_POINT('',(-17.3868386222561,64.97,-30.0279296716277));
#39401=CARTESIAN_POINT('',(-17.8521891662412,64.97,-29.5842963748526));
#39402=CARTESIAN_POINT('',(-17.8521891662412,64.97,-29.5842963748526));
#39403=CARTESIAN_POINT('',(-18.3016633687267,64.97,-29.0979679504746));
#39404=CARTESIAN_POINT('',(-18.3016633687267,64.97,-29.0979679504746));
#39405=CARTESIAN_POINT('',(-18.7335012750361,64.97,-28.5707303109632));
#39406=CARTESIAN_POINT('',(-18.7335012750361,64.97,-28.5707303109632));
#39407=CARTESIAN_POINT('',(-18.6658347245569,64.97,-28.2937154744401));
#39408=CARTESIAN_POINT('',(-18.6658347245569,64.97,-28.2937154744401));
#39409=CARTESIAN_POINT('',(-18.5940721560646,64.97,-28.0177333817765));
#39410=CARTESIAN_POINT('',(-18.5940721560646,64.97,-28.0177333817765));
#39411=CARTESIAN_POINT('',(-18.518229317088,64.97,-27.742844594294));
#39412=CARTESIAN_POINT('',(-18.518229317088,64.97,-27.742844594294));
#39413=CARTESIAN_POINT('',(-18.4383228505279,64.97,-27.4691094334002));
#39414=CARTESIAN_POINT('',(-18.4383228505279,64.97,-27.4691094334002));
#39415=CARTESIAN_POINT('',(-17.8007214335911,64.97,-27.2284271969067));
#39416=CARTESIAN_POINT('',(-17.8007214335911,64.97,-27.2284271969067));
#39417=CARTESIAN_POINT('',(-17.1683011437039,64.97,-27.0319915280556));
#39418=CARTESIAN_POINT('',(-17.1683011437039,64.97,-27.0319915280556));
#39419=CARTESIAN_POINT('',(-16.5434791025604,64.97,-26.8804690950764));
#39420=CARTESIAN_POINT('',(-16.5434791025604,64.97,-26.8804690950764));
#39421=CARTESIAN_POINT('',(-15.9288433214812,64.97,-26.7749139194219));
#39422=CARTESIAN_POINT('',(-15.9288433214812,64.97,-26.7749139194219));
#39423=CARTESIAN_POINT('',(-15.3272905060348,64.97,-26.7170853977691));
#39424=CARTESIAN_POINT('',(-12.1503952336939,64.97,-28.1092852366672));
#39425=CARTESIAN_POINT('',(-7.02885984751459,64.97,-30.4016841827556));
#39426=CARTESIAN_POINT('',(-11.3124568369342,64.97,-26.46875));
#39427=CARTESIAN_POINT('',(-11.3124568369342,64.97,-26.46875));
#39428=CARTESIAN_POINT('',(-10.3106808445568,64.97,-24.9228064432661));
#39429=CARTESIAN_POINT('',(-10.5829448433309,64.97,-25.3429650194728));
#39430=CARTESIAN_POINT('',(-13.0730690072096,64.97,-22.9241469865312));
#39431=CARTESIAN_POINT('',(-4.99838017360698,64.97,-28.7663937119056));
#39432=CARTESIAN_POINT('',(-13.1048089083576,64.97,-22.8676343517052));
#39433=CARTESIAN_POINT('',(-13.1048089083576,64.97,-22.8676343517052));
#39434=CARTESIAN_POINT('',(-13.3555043472661,64.97,-22.3177600709842));
#39435=CARTESIAN_POINT('',(-13.3555043472661,64.97,-22.3177600709842));
#39436=CARTESIAN_POINT('',(-13.571408774188,64.97,-21.7326922826676));
#39437=CARTESIAN_POINT('',(-13.571408774188,64.97,-21.7326922826676));
#39438=CARTESIAN_POINT('',(-13.7525975185565,64.97,-21.1158193057032));
#39439=CARTESIAN_POINT('',(-13.7525975185565,64.97,-21.1158193057032));
#39440=CARTESIAN_POINT('',(-13.8986893840657,64.97,-20.4699094343666));
#39441=CARTESIAN_POINT('',(-13.8986893840657,64.97,-20.4699094343666));
#39442=CARTESIAN_POINT('',(-14.009053161491,64.97,-19.7973892915637));
#39443=CARTESIAN_POINT('',(-14.009053161491,64.97,-19.7973892915637));
#39444=CARTESIAN_POINT('',(-13.8119447915281,64.97,-19.5913206811491));
#39445=CARTESIAN_POINT('',(-13.8119447915281,64.97,-19.5913206811491));
#39446=CARTESIAN_POINT('',(-13.611805537841,64.97,-19.388194462159));
#39447=CARTESIAN_POINT('',(-13.611805537841,64.97,-19.388194462159));
#39448=CARTESIAN_POINT('',(-13.4086793188509,64.97,-19.1880552084719));
#39449=CARTESIAN_POINT('',(-13.4086793188509,64.97,-19.1880552084719));
#39450=CARTESIAN_POINT('',(-13.2026107084363,64.97,-18.990946838509));
#39451=CARTESIAN_POINT('',(-13.2026107084363,64.97,-18.990946838509));
#39452=CARTESIAN_POINT('',(-12.5300905656334,64.97,-19.1013106159343));
#39453=CARTESIAN_POINT('',(-12.5300905656334,64.97,-19.1013106159343));
#39454=CARTESIAN_POINT('',(-11.8841806942968,64.97,-19.2474024814435));
#39455=CARTESIAN_POINT('',(-11.8841806942968,64.97,-19.2474024814435));
#39456=CARTESIAN_POINT('',(-11.2673077173324,64.97,-19.428591225812));
#39457=CARTESIAN_POINT('',(-11.2673077173324,64.97,-19.428591225812));
#39458=CARTESIAN_POINT('',(-10.6822399290158,64.97,-19.6444956527339));
#39459=CARTESIAN_POINT('',(-10.6822399290158,64.97,-19.6444956527339));
#39460=CARTESIAN_POINT('',(-10.1323656482948,64.97,-19.8951910916424));
#39461=CARTESIAN_POINT('',(-8.07719355673392,64.97,-22.6893191554432));
#39462=CARTESIAN_POINT('',(-4.78801327896586,64.97,-27.2353625714542));
#39463=CARTESIAN_POINT('',(-6.53125,64.97,-21.6875431630658));
#39464=CARTESIAN_POINT('',(-6.53125,64.97,-21.6875431630658));
#39465=CARTESIAN_POINT('',(-4.8907147633328,64.97,-20.8496047663061));
#39466=CARTESIAN_POINT('',(-5.33658159091048,64.97,-21.077340767532));
#39467=CARTESIAN_POINT('',(-6.28368335893612,64.97,-17.7375208219333));
#39468=CARTESIAN_POINT('',(-2.21192106406889,64.97,-26.8343993180852));
#39469=CARTESIAN_POINT('',(-6.28291460223091,64.97,-17.6727094939652));
#39470=CARTESIAN_POINT('',(-6.28291460223091,64.97,-17.6727094939652));
#39471=CARTESIAN_POINT('',(-6.22508608057805,64.97,-17.0711566785188));
#39472=CARTESIAN_POINT('',(-6.22508608057805,64.97,-17.0711566785188));
#39473=CARTESIAN_POINT('',(-6.11953090492364,64.97,-16.4565208974396));
#39474=CARTESIAN_POINT('',(-6.11953090492364,64.97,-16.4565208974396));
#39475=CARTESIAN_POINT('',(-5.96800847194436,64.97,-15.8316988562961));
#39476=CARTESIAN_POINT('',(-5.96800847194436,64.97,-15.8316988562961));
#39477=CARTESIAN_POINT('',(-5.7715728030933,64.97,-15.1992785664089));
#39478=CARTESIAN_POINT('',(-5.7715728030933,64.97,-15.1992785664089));
#39479=CARTESIAN_POINT('',(-5.53089056659976,64.97,-14.5616771494721));
#39480=CARTESIAN_POINT('',(-5.53089056659977,64.97,-14.5616771494721));
#39481=CARTESIAN_POINT('',(-5.25715540570604,64.97,-14.481770682912));
#39482=CARTESIAN_POINT('',(-5.25715540570604,64.97,-14.481770682912));
#39483=CARTESIAN_POINT('',(-4.98226661822352,64.97,-14.4059278439354));
#39484=CARTESIAN_POINT('',(-4.98226661822353,64.97,-14.4059278439354));
#39485=CARTESIAN_POINT('',(-4.70628452555987,64.97,-14.3341652754431));
#39486=CARTESIAN_POINT('',(-4.70628452555987,64.97,-14.3341652754431));
#39487=CARTESIAN_POINT('',(-4.42926968903683,64.97,-14.2664987249639));
#39488=CARTESIAN_POINT('',(-4.42926968903683,64.97,-14.2664987249639));
#39489=CARTESIAN_POINT('',(-3.90203204952539,64.97,-14.6983366312733));
#39490=CARTESIAN_POINT('',(-3.90203204952539,64.97,-14.6983366312733));
#39491=CARTESIAN_POINT('',(-3.4157036251474,64.97,-15.1478108337588));
#39492=CARTESIAN_POINT('',(-3.4157036251474,64.97,-15.1478108337588));
#39493=CARTESIAN_POINT('',(-2.97207032837233,64.97,-15.6131613777439));
#39494=CARTESIAN_POINT('',(-2.97207032837233,64.97,-15.6131613777439));
#39495=CARTESIAN_POINT('',(-2.57333897421511,64.97,-16.0926739904062));
#39496=CARTESIAN_POINT('',(-2.57333897421511,64.97,-16.0926739904062));
#39497=CARTESIAN_POINT('',(-2.22248159767725,64.97,-16.5847197494743));
#39498=CARTESIAN_POINT('',(-1.83971438913717,64.97,-20.0320916799333));
#39499=CARTESIAN_POINT('',(-1.26422241896876,64.97,-25.6136709037898));
#39500=CARTESIAN_POINT('',(1.11022302462516E-15,64.97,-19.9375));
#39501=CARTESIAN_POINT('',(7.99847440693115E-16,64.97,-19.9375));
#39502=CARTESIAN_POINT('',(1.83971438913717,64.97,-20.0320916799333));
#39503=CARTESIAN_POINT('',(1.33971438913717,64.97,-20.0063834285624));
#39504=CARTESIAN_POINT('',(2.18941017085717,64.97,-16.6404636275951));
#39505=CARTESIAN_POINT('',(1.16722050830783,64.97,-26.5544726478367));
#39506=CARTESIAN_POINT('',(2.22248159767725,64.97,-16.5847197494743));
#39507=CARTESIAN_POINT('',(2.22248159767725,64.97,-16.5847197494743));
#39508=CARTESIAN_POINT('',(2.57333897421511,64.97,-16.0926739904062));
#39509=CARTESIAN_POINT('',(2.57333897421511,64.97,-16.0926739904062));
#39510=CARTESIAN_POINT('',(2.97207032837233,64.97,-15.6131613777439));
#39511=CARTESIAN_POINT('',(2.97207032837233,64.97,-15.6131613777439));
#39512=CARTESIAN_POINT('',(3.41570362514739,64.97,-15.1478108337588));
#39513=CARTESIAN_POINT('',(3.41570362514739,64.97,-15.1478108337588));
#39514=CARTESIAN_POINT('',(3.90203204952539,64.97,-14.6983366312733));
#39515=CARTESIAN_POINT('',(3.90203204952539,64.97,-14.6983366312733));
#39516=CARTESIAN_POINT('',(4.42926968903683,64.97,-14.2664987249639));
#39517=CARTESIAN_POINT('',(4.42926968903683,64.97,-14.2664987249639));
#39518=CARTESIAN_POINT('',(4.70628452555987,64.97,-14.3341652754431));
#39519=CARTESIAN_POINT('',(4.70628452555987,64.97,-14.3341652754431));
#39520=CARTESIAN_POINT('',(4.98226661822352,64.97,-14.4059278439354));
#39521=CARTESIAN_POINT('',(4.98226661822352,64.97,-14.4059278439354));
#39522=CARTESIAN_POINT('',(5.25715540570603,64.97,-14.481770682912));
#39523=CARTESIAN_POINT('',(5.25715540570603,64.97,-14.481770682912));
#39524=CARTESIAN_POINT('',(5.53089056659976,64.97,-14.5616771494721));
#39525=CARTESIAN_POINT('',(5.53089056659976,64.97,-14.5616771494721));
#39526=CARTESIAN_POINT('',(5.77157280309329,64.97,-15.1992785664089));
#39527=CARTESIAN_POINT('',(5.77157280309329,64.97,-15.1992785664089));
#39528=CARTESIAN_POINT('',(5.96800847194436,64.97,-15.8316988562961));
#39529=CARTESIAN_POINT('',(5.96800847194436,64.97,-15.8316988562961));
#39530=CARTESIAN_POINT('',(6.11953090492364,64.97,-16.4565208974396));
#39531=CARTESIAN_POINT('',(6.11953090492364,64.97,-16.4565208974396));
#39532=CARTESIAN_POINT('',(6.22508608057805,64.97,-17.0711566785188));
#39533=CARTESIAN_POINT('',(6.22508608057805,64.97,-17.0711566785188));
#39534=CARTESIAN_POINT('',(6.28291460223091,64.97,-17.6727094939652));
#39535=CARTESIAN_POINT('',(-1.04094977927525E-15,64.97,-41.5));
#39536=CARTESIAN_POINT('Origin',(0.,64.97,-33.));
#39537=CARTESIAN_POINT('Origin',(0.918538851438207,64.72,-26.5288321810589));
#39538=CARTESIAN_POINT('',(1.92399462146589,64.7518675845618,-17.0878374925667));
#39539=CARTESIAN_POINT('',(-2.47408096220597,61.1372984587275,-24.5010582960093));
#39540=CARTESIAN_POINT('',(-5.80560826253415,57.3246773483287,-19.6389959268513));
#39541=CARTESIAN_POINT('',(-1.61076884470925,62.0175738804575,-24.7108426070529));
#39542=CARTESIAN_POINT('Origin',(-1.01554076209914,64.72,-25.588030437012));
#39543=CARTESIAN_POINT('',(-1.53371821045904,64.47,-18.1247799404686));
#39544=CARTESIAN_POINT('',(0.0410640680949126,63.4588711803305,-23.5395511505951));
#39545=CARTESIAN_POINT('',(-1.33971438913717,64.47,-20.0063834285624));
#39546=CARTESIAN_POINT('',(-0.766859105229518,64.47,-25.5623899702343));
#39547=CARTESIAN_POINT('',(5.45809628639077,57.6721893244721,-19.6568637773255));
#39548=CARTESIAN_POINT('Origin',(-2.44010592976206,64.72,-26.9365348509256));
#39549=CARTESIAN_POINT('',(-6.28985303478256,64.7518675845618,-18.2576657286835));
#39550=CARTESIAN_POINT('',(-6.39208781628514,61.1372984587275,-26.876741060164));
#39551=CARTESIAN_POINT('',(-11.7083062763497,57.3246773483287,-24.331835183853));
#39552=CARTESIAN_POINT('',(-5.53954543561629,62.0175738804576,-26.6267635440948));
#39553=CARTESIAN_POINT('Origin',(-4.58546888005044,64.72,-27.0888164474249));
#39554=CARTESIAN_POINT('',(-8.76584896227005,64.47,-20.8845406467914));
#39555=CARTESIAN_POINT('',(-4.69466189854939,63.4588711803304,-24.7864789311647));
#39556=CARTESIAN_POINT('',(-7.65703498052716,64.47,-22.4170551566691));
#39557=CARTESIAN_POINT('',(-4.38292448113502,64.47,-26.9422703233957));
#39558=CARTESIAN_POINT('',(-1.94471807102131,57.6721893244721,-18.7154569218122));
#39559=CARTESIAN_POINT('Origin',(-5.14492629763621,64.72,-28.968938110821));
#39560=CARTESIAN_POINT('',(-12.8183396498506,64.7518675845618,-23.3776905273493));
#39561=CARTESIAN_POINT('',(-8.59733990204194,61.1372984587275,-30.8931461122945));
#39562=CARTESIAN_POINT('',(-14.4737730786812,57.3246773483287,-31.3473022032011));
#39563=CARTESIAN_POINT('',(-7.98400530061442,62.0175738804576,-30.2503880426691));
#39564=CARTESIAN_POINT('Origin',(-6.9267243146742,64.72,-30.1734993170625));
#39565=CARTESIAN_POINT('',(-13.6491775636676,64.47,-26.8906289027386));
#39566=CARTESIAN_POINT('',(-8.17245700074035,63.4588711803304,-28.2342130491446));
#39567=CARTESIAN_POINT('',(-11.922659232468,64.47,-27.6634184090895));
#39568=CARTESIAN_POINT('',(-6.8245887818338,64.47,-29.9453144513693));
#39569=CARTESIAN_POINT('',(-8.82644679179704,57.6721893244721,-21.6015818483468));
#39570=CARTESIAN_POINT('Origin',(-6.47116781894107,64.72,-32.0814611485618));
#39571=CARTESIAN_POINT('',(-15.9121625074333,64.7518675845618,-31.0760053785341));
#39572=CARTESIAN_POINT('',(-8.49894170399068,61.1372984587276,-35.4740809622059));
#39573=CARTESIAN_POINT('',(-13.3610040731487,57.3246773483287,-38.8056082625342));
#39574=CARTESIAN_POINT('',(-8.28915739294713,62.0175738804576,-34.6107688447092));
#39575=CARTESIAN_POINT('Origin',(-7.41196956298797,64.72,-34.0155407620991));
#39576=CARTESIAN_POINT('',(-14.8752200595314,64.47,-34.533718210459));
#39577=CARTESIAN_POINT('',(-9.46044884940471,63.4588711803303,-32.9589359319049));
#39578=CARTESIAN_POINT('',(-12.9936165714376,64.47,-34.3397143891372));
#39579=CARTESIAN_POINT('',(-7.43761002976572,64.47,-33.7668591052295));
#39580=CARTESIAN_POINT('',(-13.3431362226745,57.6721893244721,-27.5419037136092));
#39581=CARTESIAN_POINT('Origin',(-6.06346514907441,64.72,-35.4401059297621));
#39582=CARTESIAN_POINT('',(-14.7423342713165,64.7518675845618,-39.2898530347826));
#39583=CARTESIAN_POINT('',(-6.12325893983596,61.1372984587275,-39.3920878162851));
#39584=CARTESIAN_POINT('',(-8.66816481614703,57.3246773483287,-44.7083062763498));
#39585=CARTESIAN_POINT('',(-6.37323645590517,62.0175738804575,-38.5395454356163));
#39586=CARTESIAN_POINT('Origin',(-5.91118355257507,64.72,-37.5854688800504));
#39587=CARTESIAN_POINT('',(-12.1154593532086,64.47,-41.76584896227));
#39588=CARTESIAN_POINT('',(-8.21352106883533,63.4588711803304,-37.6946618985493));
#39589=CARTESIAN_POINT('',(-10.5829448433309,64.47,-40.6570349805272));
#39590=CARTESIAN_POINT('',(-6.0577296766043,64.47,-37.382924481135));
#39591=CARTESIAN_POINT('',(-14.2845430781878,57.6721893244721,-34.9447180710213));
#39592=CARTESIAN_POINT('Origin',(-4.03106188917902,64.72,-38.1449262976362));
#39593=CARTESIAN_POINT('',(-9.62230947265071,64.7518675845618,-45.8183396498506));
#39594=CARTESIAN_POINT('',(-2.10685388770528,61.1372984587272,-41.5973399020421));
#39595=CARTESIAN_POINT('',(-1.65269779679893,57.3246773483287,-47.4737730786812));
#39596=CARTESIAN_POINT('',(-2.74961195733092,62.0175738804576,-40.9840053006144));
#39597=CARTESIAN_POINT('Origin',(-2.82650068293752,64.72,-39.9267243146742));
#39598=CARTESIAN_POINT('',(-6.10937109726139,64.47,-46.6491775636676));
#39599=CARTESIAN_POINT('',(-4.76578695085539,63.4588711803305,-41.1724570007404));
#39600=CARTESIAN_POINT('',(-5.33658159091048,64.47,-44.922659232468));
#39601=CARTESIAN_POINT('',(-3.05468554863069,64.47,-39.8245887818338));
#39602=CARTESIAN_POINT('',(-11.3984181516531,57.6721893244721,-41.826446791797));
#39603=CARTESIAN_POINT('Origin',(-0.918538851438202,64.72,-39.4711678189411));
#39604=CARTESIAN_POINT('',(-1.92399462146589,64.7518675845618,-48.9121625074333));
#39605=CARTESIAN_POINT('',(2.47408096220598,61.1372984587275,-41.4989417039907));
#39606=CARTESIAN_POINT('',(5.80560826253417,57.3246773483287,-46.3610040731487));
#39607=CARTESIAN_POINT('',(1.61076884470942,62.0175738804574,-41.2891573929471));
#39608=CARTESIAN_POINT('Origin',(1.01554076209913,64.72,-40.411969562988));
#39609=CARTESIAN_POINT('',(1.53371821045902,64.47,-47.8752200595314));
#39610=CARTESIAN_POINT('',(-0.0410640680949548,63.4588711803305,-42.4604488494049));
#39611=CARTESIAN_POINT('',(1.33971438913717,64.47,-45.9936165714376));
#39612=CARTESIAN_POINT('',(0.766859105229514,64.47,-40.4376100297657));
#39613=CARTESIAN_POINT('',(-5.45809628639078,57.6721893244721,-46.3431362226745));
#39614=CARTESIAN_POINT('Origin',(2.44010592976207,64.72,-39.0634651490744));
#39615=CARTESIAN_POINT('',(6.28985303478254,64.7518675845618,-47.7423342713165));
#39616=CARTESIAN_POINT('',(6.39208781628516,61.1372984587275,-39.123258939836));
#39617=CARTESIAN_POINT('',(11.7083062763498,57.3246773483287,-41.6681648161471));
#39618=CARTESIAN_POINT('',(5.53954543561639,62.0175738804574,-39.3732364559051));
#39619=CARTESIAN_POINT('Origin',(4.58546888005044,64.72,-38.9111835525751));
#39620=CARTESIAN_POINT('',(8.76584896227005,64.47,-45.1154593532086));
#39621=CARTESIAN_POINT('',(4.6946618985495,63.4588711803305,-41.2135210688354));
#39622=CARTESIAN_POINT('',(7.65703498052716,64.47,-43.5829448433309));
#39623=CARTESIAN_POINT('',(4.38292448113502,64.47,-39.0577296766043));
#39624=CARTESIAN_POINT('',(1.94471807102132,57.6721893244721,-47.2845430781878));
#39625=CARTESIAN_POINT('Origin',(5.1449262976362,64.72,-37.031061889179));
#39626=CARTESIAN_POINT('',(12.8183396498506,64.7518675845618,-42.6223094726507));
#39627=CARTESIAN_POINT('',(8.59733990204205,61.1372984587273,-35.1068538877054));
#39628=CARTESIAN_POINT('',(14.4737730786812,57.3246773483287,-34.6526977967989));
#39629=CARTESIAN_POINT('',(7.98400530061436,62.0175738804577,-35.749611957331));
#39630=CARTESIAN_POINT('Origin',(6.9267243146742,64.72,-35.8265006829375));
#39631=CARTESIAN_POINT('',(13.6491775636676,64.47,-39.1093710972614));
#39632=CARTESIAN_POINT('',(8.17245700074045,63.4588711803305,-37.7657869508554));
#39633=CARTESIAN_POINT('',(11.922659232468,64.47,-38.3365815909105));
#39634=CARTESIAN_POINT('',(6.82458878183381,64.47,-36.0546855486307));
#39635=CARTESIAN_POINT('',(8.82644679179704,57.6721893244721,-44.3984181516532));
#39636=CARTESIAN_POINT('Origin',(6.47116781894107,64.72,-33.9185388514382));
#39637=CARTESIAN_POINT('',(15.9121625074333,64.7518675845618,-34.9239946214659));
#39638=CARTESIAN_POINT('',(8.49894170399068,61.1372984587275,-30.525919037794));
#39639=CARTESIAN_POINT('',(13.3610040731487,57.3246773483287,-27.1943917374658));
#39640=CARTESIAN_POINT('',(8.28915739294707,62.0175738804573,-31.3892311552905));
#39641=CARTESIAN_POINT('Origin',(7.41196956298798,64.72,-31.9844592379009));
#39642=CARTESIAN_POINT('',(14.8752200595314,64.47,-31.466281789541));
#39643=CARTESIAN_POINT('',(9.4604488494049,63.4588711803305,-33.0410640680949));
#39644=CARTESIAN_POINT('',(12.9936165714376,64.47,-31.6602856108628));
#39645=CARTESIAN_POINT('',(7.43761002976572,64.47,-32.2331408947705));
#39646=CARTESIAN_POINT('',(13.3431362226745,57.6721893244721,-38.4580962863908));
#39647=CARTESIAN_POINT('Origin',(6.06346514907441,64.72,-30.5598940702379));
#39648=CARTESIAN_POINT('',(14.7423342713165,64.7518675845618,-26.7101469652175));
#39649=CARTESIAN_POINT('',(6.12325893983594,61.1372984587275,-26.6079121837148));
#39650=CARTESIAN_POINT('',(8.66816481614703,57.3246773483287,-21.2916937236502));
#39651=CARTESIAN_POINT('',(6.37323645590513,62.0175738804575,-27.4604545643837));
#39652=CARTESIAN_POINT('Origin',(5.91118355257506,64.72,-28.4145311199496));
#39653=CARTESIAN_POINT('',(12.1154593532086,64.47,-24.23415103773));
#39654=CARTESIAN_POINT('',(8.21352106883536,63.4588711803305,-28.3053381014505));
#39655=CARTESIAN_POINT('',(10.5829448433309,64.47,-25.3429650194728));
#39656=CARTESIAN_POINT('',(6.05772967660429,64.47,-28.617075518865));
#39657=CARTESIAN_POINT('',(14.2845430781878,57.6721893244721,-31.0552819289787));
#39658=CARTESIAN_POINT('Origin',(4.03106188917902,64.72,-27.8550737023638));
#39659=CARTESIAN_POINT('',(9.62230947265072,64.7518675845618,-20.1816603501494));
#39660=CARTESIAN_POINT('',(2.10685388770537,61.1372984587273,-24.402660097958));
#39661=CARTESIAN_POINT('',(1.65269779679893,57.3246773483287,-18.5262269213188));
#39662=CARTESIAN_POINT('',(2.74961195733085,62.0175738804575,-25.0159946993856));
#39663=CARTESIAN_POINT('Origin',(5.33658159091048,37.03,-21.077340767532));
#39664=CARTESIAN_POINT('',(6.53125,37.03,-21.6875431630658));
#39665=CARTESIAN_POINT('',(5.33658159091048,37.03,-21.077340767532));
#39666=CARTESIAN_POINT('Origin',(6.10937109726139,37.03,-19.3508224363324));
#39667=CARTESIAN_POINT('',(6.10937109726139,37.03,-19.3508224363324));
#39668=CARTESIAN_POINT('Origin',(6.23934797313093,37.03,-18.8210104177224));
#39669=CARTESIAN_POINT('Origin',(6.22508608057805,37.03,-17.0711566785188));
#39670=CARTESIAN_POINT('',(6.22508608057805,37.03,-17.0711566785188));
#39671=CARTESIAN_POINT('Origin',(6.11953090492364,37.03,-16.4565208974396));
#39672=CARTESIAN_POINT('',(6.11953090492364,37.03,-16.4565208974396));
#39673=CARTESIAN_POINT('Origin',(5.96800847194436,37.03,-15.8316988562961));
#39674=CARTESIAN_POINT('',(5.96800847194436,37.03,-15.8316988562961));
#39675=CARTESIAN_POINT('Origin',(5.77157280309329,37.03,-15.1992785664089));
#39676=CARTESIAN_POINT('',(5.77157280309329,37.03,-15.1992785664089));
#39677=CARTESIAN_POINT('Origin',(5.53089056659976,37.03,-14.5616771494721));
#39678=CARTESIAN_POINT('',(5.53089056659976,37.03,-14.5616771494721));
#39679=CARTESIAN_POINT('Origin',(5.25715540570603,37.03,-14.481770682912));
#39680=CARTESIAN_POINT('',(5.25715540570603,37.03,-14.481770682912));
#39681=CARTESIAN_POINT('Origin',(4.98226661822352,37.03,-14.4059278439354));
#39682=CARTESIAN_POINT('',(4.98226661822352,37.03,-14.4059278439354));
#39683=CARTESIAN_POINT('Origin',(4.70628452555987,37.03,-14.3341652754431));
#39684=CARTESIAN_POINT('',(4.70628452555987,37.03,-14.3341652754431));
#39685=CARTESIAN_POINT('Origin',(4.42926968903683,37.03,-14.2664987249639));
#39686=CARTESIAN_POINT('',(4.42926968903683,37.03,-14.2664987249639));
#39687=CARTESIAN_POINT('Origin',(3.90203204952539,37.03,-14.6983366312733));
#39688=CARTESIAN_POINT('',(3.90203204952539,37.03,-14.6983366312733));
#39689=CARTESIAN_POINT('Origin',(3.41570362514739,37.03,-15.1478108337588));
#39690=CARTESIAN_POINT('',(3.41570362514739,37.03,-15.1478108337588));
#39691=CARTESIAN_POINT('Origin',(2.97207032837233,37.03,-15.6131613777439));
#39692=CARTESIAN_POINT('',(2.97207032837233,37.03,-15.6131613777439));
#39693=CARTESIAN_POINT('Origin',(2.57333897421511,37.03,-16.0926739904062));
#39694=CARTESIAN_POINT('',(2.57333897421511,37.03,-16.0926739904062));
#39695=CARTESIAN_POINT('Origin',(2.22248159767725,37.03,-16.5847197494743));
#39696=CARTESIAN_POINT('',(2.22248159767725,37.03,-16.5847197494743));
#39697=CARTESIAN_POINT('Origin',(1.92399462146589,37.03,-17.0878374925667));
#39698=CARTESIAN_POINT('',(1.92399462146589,37.03,-17.0878374925667));
#39699=CARTESIAN_POINT('Origin',(1.68606094335648,37.03,-17.6009608351872));
#39700=CARTESIAN_POINT('Origin',(8.32667268468867E-16,37.03,-19.9375));
#39701=CARTESIAN_POINT('',(7.99847440693115E-16,37.03,-19.9375));
#39702=CARTESIAN_POINT('Origin',(-1.33971438913717,37.03,-20.0063834285624));
#39703=CARTESIAN_POINT('',(-1.33971438913717,37.03,-20.0063834285624));
#39704=CARTESIAN_POINT('Origin',(-1.53371821045904,37.03,-18.1247799404686));
#39705=CARTESIAN_POINT('',(-1.53371821045904,37.03,-18.1247799404686));
#39706=CARTESIAN_POINT('Origin',(-1.68606094335648,37.03,-17.6009608351872));
#39707=CARTESIAN_POINT('Origin',(-2.57333897421511,37.03,-16.0926739904062));
#39708=CARTESIAN_POINT('',(-2.57333897421511,37.03,-16.0926739904062));
#39709=CARTESIAN_POINT('Origin',(-2.97207032837233,37.03,-15.6131613777439));
#39710=CARTESIAN_POINT('',(-2.97207032837233,37.03,-15.6131613777439));
#39711=CARTESIAN_POINT('Origin',(-3.4157036251474,37.03,-15.1478108337588));
#39712=CARTESIAN_POINT('',(-3.4157036251474,37.03,-15.1478108337588));
#39713=CARTESIAN_POINT('Origin',(-3.90203204952539,37.03,-14.6983366312733));
#39714=CARTESIAN_POINT('',(-3.90203204952539,37.03,-14.6983366312733));
#39715=CARTESIAN_POINT('Origin',(-4.42926968903683,37.03,-14.2664987249639));
#39716=CARTESIAN_POINT('',(-4.42926968903683,37.03,-14.2664987249639));
#39717=CARTESIAN_POINT('Origin',(-4.70628452555987,37.03,-14.3341652754431));
#39718=CARTESIAN_POINT('',(-4.70628452555987,37.03,-14.3341652754431));
#39719=CARTESIAN_POINT('Origin',(-4.98226661822353,37.03,-14.4059278439354));
#39720=CARTESIAN_POINT('',(-4.98226661822353,37.03,-14.4059278439354));
#39721=CARTESIAN_POINT('Origin',(-5.25715540570604,37.03,-14.481770682912));
#39722=CARTESIAN_POINT('',(-5.25715540570604,37.03,-14.481770682912));
#39723=CARTESIAN_POINT('Origin',(-5.53089056659977,37.03,-14.5616771494721));
#39724=CARTESIAN_POINT('',(-5.53089056659977,37.03,-14.5616771494721));
#39725=CARTESIAN_POINT('Origin',(-5.7715728030933,37.03,-15.1992785664089));
#39726=CARTESIAN_POINT('',(-5.7715728030933,37.03,-15.1992785664089));
#39727=CARTESIAN_POINT('Origin',(-5.96800847194436,37.03,-15.8316988562961));
#39728=CARTESIAN_POINT('',(-5.96800847194436,37.03,-15.8316988562961));
#39729=CARTESIAN_POINT('Origin',(-6.11953090492364,37.03,-16.4565208974396));
#39730=CARTESIAN_POINT('',(-6.11953090492364,37.03,-16.4565208974396));
#39731=CARTESIAN_POINT('Origin',(-6.22508608057805,37.03,-17.0711566785188));
#39732=CARTESIAN_POINT('',(-6.22508608057805,37.03,-17.0711566785188));
#39733=CARTESIAN_POINT('Origin',(-6.28291460223091,37.03,-17.6727094939652));
#39734=CARTESIAN_POINT('',(-6.28291460223091,37.03,-17.6727094939652));
#39735=CARTESIAN_POINT('Origin',(-6.28985303478256,37.03,-18.2576657286835));
#39736=CARTESIAN_POINT('',(-6.28985303478256,37.03,-18.2576657286835));
#39737=CARTESIAN_POINT('Origin',(-6.23934797313094,37.03,-18.8210104177224));
#39738=CARTESIAN_POINT('Origin',(-6.53125,37.03,-21.6875431630658));
#39739=CARTESIAN_POINT('',(-6.53125,37.03,-21.6875431630658));
#39740=CARTESIAN_POINT('Origin',(-7.65703498052716,37.03,-22.4170551566691));
#39741=CARTESIAN_POINT('',(-7.65703498052716,37.03,-22.4170551566691));
#39742=CARTESIAN_POINT('Origin',(-8.76584896227005,37.03,-20.8845406467914));
#39743=CARTESIAN_POINT('',(-8.76584896227005,37.03,-20.8845406467914));
#39744=CARTESIAN_POINT('Origin',(-9.15969119168187,37.03,-20.5070713610788));
#39745=CARTESIAN_POINT('Origin',(-10.6822399290158,37.03,-19.6444956527339));
#39746=CARTESIAN_POINT('',(-10.6822399290158,37.03,-19.6444956527339));
#39747=CARTESIAN_POINT('Origin',(-11.2673077173324,37.03,-19.428591225812));
#39748=CARTESIAN_POINT('',(-11.2673077173324,37.03,-19.428591225812));
#39749=CARTESIAN_POINT('Origin',(-11.8841806942968,37.03,-19.2474024814435));
#39750=CARTESIAN_POINT('',(-11.8841806942968,37.03,-19.2474024814435));
#39751=CARTESIAN_POINT('Origin',(-12.5300905656334,37.03,-19.1013106159343));
#39752=CARTESIAN_POINT('',(-12.5300905656334,37.03,-19.1013106159343));
#39753=CARTESIAN_POINT('Origin',(-13.2026107084363,37.03,-18.990946838509));
#39754=CARTESIAN_POINT('',(-13.2026107084363,37.03,-18.990946838509));
#39755=CARTESIAN_POINT('Origin',(-13.4086793188509,37.03,-19.1880552084719));
#39756=CARTESIAN_POINT('',(-13.4086793188509,37.03,-19.1880552084719));
#39757=CARTESIAN_POINT('Origin',(-13.611805537841,37.03,-19.388194462159));
#39758=CARTESIAN_POINT('',(-13.611805537841,37.03,-19.388194462159));
#39759=CARTESIAN_POINT('Origin',(-13.8119447915281,37.03,-19.5913206811491));
#39760=CARTESIAN_POINT('',(-13.8119447915281,37.03,-19.5913206811491));
#39761=CARTESIAN_POINT('Origin',(-14.009053161491,37.03,-19.7973892915637));
#39762=CARTESIAN_POINT('',(-14.009053161491,37.03,-19.7973892915637));
#39763=CARTESIAN_POINT('Origin',(-13.8986893840657,37.03,-20.4699094343666));
#39764=CARTESIAN_POINT('',(-13.8986893840657,37.03,-20.4699094343666));
#39765=CARTESIAN_POINT('Origin',(-13.7525975185565,37.03,-21.1158193057032));
#39766=CARTESIAN_POINT('',(-13.7525975185565,37.03,-21.1158193057032));
#39767=CARTESIAN_POINT('Origin',(-13.571408774188,37.03,-21.7326922826676));
#39768=CARTESIAN_POINT('',(-13.571408774188,37.03,-21.7326922826676));
#39769=CARTESIAN_POINT('Origin',(-13.3555043472661,37.03,-22.3177600709842));
#39770=CARTESIAN_POINT('',(-13.3555043472661,37.03,-22.3177600709842));
#39771=CARTESIAN_POINT('Origin',(-13.1048089083576,37.03,-22.8676343517052));
#39772=CARTESIAN_POINT('',(-13.1048089083576,37.03,-22.8676343517052));
#39773=CARTESIAN_POINT('Origin',(-12.8183396498506,37.03,-23.3776905273493));
#39774=CARTESIAN_POINT('',(-12.8183396498506,37.03,-23.3776905273493));
#39775=CARTESIAN_POINT('Origin',(-12.4929286389212,37.03,-23.8403088083181));
#39776=CARTESIAN_POINT('Origin',(-11.3124568369342,37.03,-26.46875));
#39777=CARTESIAN_POINT('',(-11.3124568369342,37.03,-26.46875));
#39778=CARTESIAN_POINT('Origin',(-11.922659232468,37.03,-27.6634184090895));
#39779=CARTESIAN_POINT('',(-11.922659232468,37.03,-27.6634184090895));
#39780=CARTESIAN_POINT('Origin',(-13.6491775636676,37.03,-26.8906289027386));
#39781=CARTESIAN_POINT('',(-13.6491775636676,37.03,-26.8906289027386));
#39782=CARTESIAN_POINT('Origin',(-14.1789895822776,37.03,-26.7606520268691));
#39783=CARTESIAN_POINT('Origin',(-15.9288433214812,37.03,-26.7749139194219));
#39784=CARTESIAN_POINT('',(-15.9288433214812,37.03,-26.7749139194219));
#39785=CARTESIAN_POINT('Origin',(-16.5434791025604,37.03,-26.8804690950764));
#39786=CARTESIAN_POINT('',(-16.5434791025604,37.03,-26.8804690950764));
#39787=CARTESIAN_POINT('Origin',(-17.1683011437039,37.03,-27.0319915280556));
#39788=CARTESIAN_POINT('',(-17.1683011437039,37.03,-27.0319915280556));
#39789=CARTESIAN_POINT('Origin',(-17.8007214335911,37.03,-27.2284271969067));
#39790=CARTESIAN_POINT('',(-17.8007214335911,37.03,-27.2284271969067));
#39791=CARTESIAN_POINT('Origin',(-18.4383228505279,37.03,-27.4691094334002));
#39792=CARTESIAN_POINT('',(-18.4383228505279,37.03,-27.4691094334002));
#39793=CARTESIAN_POINT('Origin',(-18.518229317088,37.03,-27.742844594294));
#39794=CARTESIAN_POINT('',(-18.518229317088,37.03,-27.742844594294));
#39795=CARTESIAN_POINT('Origin',(-18.5940721560646,37.03,-28.0177333817765));
#39796=CARTESIAN_POINT('',(-18.5940721560646,37.03,-28.0177333817765));
#39797=CARTESIAN_POINT('Origin',(-18.6658347245569,37.03,-28.2937154744401));
#39798=CARTESIAN_POINT('',(-18.6658347245569,37.03,-28.2937154744401));
#39799=CARTESIAN_POINT('Origin',(-18.7335012750361,37.03,-28.5707303109632));
#39800=CARTESIAN_POINT('',(-18.7335012750361,37.03,-28.5707303109632));
#39801=CARTESIAN_POINT('Origin',(-18.3016633687267,37.03,-29.0979679504746));
#39802=CARTESIAN_POINT('',(-18.3016633687267,37.03,-29.0979679504746));
#39803=CARTESIAN_POINT('Origin',(-17.8521891662412,37.03,-29.5842963748526));
#39804=CARTESIAN_POINT('',(-17.8521891662412,37.03,-29.5842963748526));
#39805=CARTESIAN_POINT('Origin',(-17.3868386222561,37.03,-30.0279296716277));
#39806=CARTESIAN_POINT('',(-17.3868386222561,37.03,-30.0279296716277));
#39807=CARTESIAN_POINT('Origin',(-16.9073260095938,37.03,-30.4266610257849));
#39808=CARTESIAN_POINT('',(-16.9073260095938,37.03,-30.4266610257849));
#39809=CARTESIAN_POINT('Origin',(-16.4152802505257,37.03,-30.7775184023227));
#39810=CARTESIAN_POINT('',(-16.4152802505257,37.03,-30.7775184023227));
#39811=CARTESIAN_POINT('Origin',(-15.9121625074333,37.03,-31.0760053785341));
#39812=CARTESIAN_POINT('',(-15.9121625074333,37.03,-31.0760053785341));
#39813=CARTESIAN_POINT('Origin',(-15.3990391648128,37.03,-31.3139390566435));
#39814=CARTESIAN_POINT('Origin',(-13.0625,37.03,-33.));
#39815=CARTESIAN_POINT('',(-13.0625,37.03,-33.));
#39816=CARTESIAN_POINT('Origin',(-12.9936165714376,37.03,-34.3397143891372));
#39817=CARTESIAN_POINT('',(-12.9936165714376,37.03,-34.3397143891372));
#39818=CARTESIAN_POINT('Origin',(-14.8752200595314,37.03,-34.533718210459));
#39819=CARTESIAN_POINT('',(-14.8752200595314,37.03,-34.533718210459));
#39820=CARTESIAN_POINT('Origin',(-15.3990391648128,37.03,-34.6860609433565));
#39821=CARTESIAN_POINT('Origin',(-16.9073260095938,37.03,-35.5733389742151));
#39822=CARTESIAN_POINT('',(-16.9073260095938,37.03,-35.5733389742151));
#39823=CARTESIAN_POINT('Origin',(-17.3868386222561,37.03,-35.9720703283723));
#39824=CARTESIAN_POINT('',(-17.3868386222561,37.03,-35.9720703283723));
#39825=CARTESIAN_POINT('Origin',(-17.8521891662412,37.03,-36.4157036251474));
#39826=CARTESIAN_POINT('',(-17.8521891662412,37.03,-36.4157036251474));
#39827=CARTESIAN_POINT('Origin',(-18.3016633687267,37.03,-36.9020320495254));
#39828=CARTESIAN_POINT('',(-18.3016633687267,37.03,-36.9020320495254));
#39829=CARTESIAN_POINT('Origin',(-18.7335012750361,37.03,-37.4292696890368));
#39830=CARTESIAN_POINT('',(-18.7335012750361,37.03,-37.4292696890368));
#39831=CARTESIAN_POINT('Origin',(-18.6658347245569,37.03,-37.7062845255599));
#39832=CARTESIAN_POINT('',(-18.6658347245569,37.03,-37.7062845255599));
#39833=CARTESIAN_POINT('Origin',(-18.5940721560646,37.03,-37.9822666182235));
#39834=CARTESIAN_POINT('',(-18.5940721560646,37.03,-37.9822666182235));
#39835=CARTESIAN_POINT('Origin',(-18.518229317088,37.03,-38.257155405706));
#39836=CARTESIAN_POINT('',(-18.518229317088,37.03,-38.257155405706));
#39837=CARTESIAN_POINT('Origin',(-18.4383228505279,37.03,-38.5308905665998));
#39838=CARTESIAN_POINT('',(-18.4383228505279,37.03,-38.5308905665998));
#39839=CARTESIAN_POINT('Origin',(-17.8007214335911,37.03,-38.7715728030933));
#39840=CARTESIAN_POINT('',(-17.8007214335911,37.03,-38.7715728030933));
#39841=CARTESIAN_POINT('Origin',(-17.1683011437039,37.03,-38.9680084719444));
#39842=CARTESIAN_POINT('',(-17.1683011437039,37.03,-38.9680084719444));
#39843=CARTESIAN_POINT('Origin',(-16.5434791025604,37.03,-39.1195309049236));
#39844=CARTESIAN_POINT('',(-16.5434791025604,37.03,-39.1195309049236));
#39845=CARTESIAN_POINT('Origin',(-15.9288433214812,37.03,-39.225086080578));
#39846=CARTESIAN_POINT('',(-15.9288433214812,37.03,-39.225086080578));
#39847=CARTESIAN_POINT('Origin',(-15.3272905060348,37.03,-39.2829146022309));
#39848=CARTESIAN_POINT('',(-15.3272905060348,37.03,-39.2829146022309));
#39849=CARTESIAN_POINT('Origin',(-14.7423342713165,37.03,-39.2898530347826));
#39850=CARTESIAN_POINT('',(-14.7423342713165,37.03,-39.2898530347826));
#39851=CARTESIAN_POINT('Origin',(-14.1789895822776,37.03,-39.2393479731309));
#39852=CARTESIAN_POINT('Origin',(-11.3124568369342,37.03,-39.53125));
#39853=CARTESIAN_POINT('',(-11.3124568369342,37.03,-39.53125));
#39854=CARTESIAN_POINT('Origin',(-10.5829448433309,37.03,-40.6570349805272));
#39855=CARTESIAN_POINT('',(-10.5829448433309,37.03,-40.6570349805272));
#39856=CARTESIAN_POINT('Origin',(-12.1154593532086,37.03,-41.76584896227));
#39857=CARTESIAN_POINT('',(-12.1154593532086,37.03,-41.76584896227));
#39858=CARTESIAN_POINT('Origin',(-12.4929286389212,37.03,-42.1596911916819));
#39859=CARTESIAN_POINT('Origin',(-13.3555043472661,37.03,-43.6822399290158));
#39860=CARTESIAN_POINT('',(-13.3555043472661,37.03,-43.6822399290158));
#39861=CARTESIAN_POINT('Origin',(-13.571408774188,37.03,-44.2673077173324));
#39862=CARTESIAN_POINT('',(-13.571408774188,37.03,-44.2673077173324));
#39863=CARTESIAN_POINT('Origin',(-13.7525975185565,37.03,-44.8841806942968));
#39864=CARTESIAN_POINT('',(-13.7525975185565,37.03,-44.8841806942968));
#39865=CARTESIAN_POINT('Origin',(-13.8986893840657,37.03,-45.5300905656334));
#39866=CARTESIAN_POINT('',(-13.8986893840657,37.03,-45.5300905656334));
#39867=CARTESIAN_POINT('Origin',(-14.009053161491,37.03,-46.2026107084363));
#39868=CARTESIAN_POINT('',(-14.009053161491,37.03,-46.2026107084363));
#39869=CARTESIAN_POINT('Origin',(-13.8119447915281,37.03,-46.4086793188509));
#39870=CARTESIAN_POINT('',(-13.8119447915281,37.03,-46.4086793188509));
#39871=CARTESIAN_POINT('Origin',(-13.611805537841,37.03,-46.611805537841));
#39872=CARTESIAN_POINT('',(-13.611805537841,37.03,-46.611805537841));
#39873=CARTESIAN_POINT('Origin',(-13.4086793188509,37.03,-46.8119447915281));
#39874=CARTESIAN_POINT('',(-13.4086793188509,37.03,-46.8119447915281));
#39875=CARTESIAN_POINT('Origin',(-13.2026107084363,37.03,-47.009053161491));
#39876=CARTESIAN_POINT('',(-13.2026107084363,37.03,-47.009053161491));
#39877=CARTESIAN_POINT('Origin',(-12.5300905656334,37.03,-46.8986893840657));
#39878=CARTESIAN_POINT('',(-12.5300905656334,37.03,-46.8986893840657));
#39879=CARTESIAN_POINT('Origin',(-11.8841806942968,37.03,-46.7525975185565));
#39880=CARTESIAN_POINT('',(-11.8841806942968,37.03,-46.7525975185565));
#39881=CARTESIAN_POINT('Origin',(-11.2673077173324,37.03,-46.571408774188));
#39882=CARTESIAN_POINT('',(-11.2673077173324,37.03,-46.571408774188));
#39883=CARTESIAN_POINT('Origin',(-10.6822399290158,37.03,-46.3555043472661));
#39884=CARTESIAN_POINT('',(-10.6822399290158,37.03,-46.3555043472661));
#39885=CARTESIAN_POINT('Origin',(-10.1323656482948,37.03,-46.1048089083576));
#39886=CARTESIAN_POINT('',(-10.1323656482948,37.03,-46.1048089083576));
#39887=CARTESIAN_POINT('Origin',(-9.62230947265071,37.03,-45.8183396498506));
#39888=CARTESIAN_POINT('',(-9.62230947265071,37.03,-45.8183396498506));
#39889=CARTESIAN_POINT('Origin',(-9.15969119168187,37.03,-45.4929286389212));
#39890=CARTESIAN_POINT('Origin',(-6.53125000000001,37.03,-44.3124568369342));
#39891=CARTESIAN_POINT('',(-6.53125000000001,37.03,-44.3124568369342));
#39892=CARTESIAN_POINT('Origin',(-5.33658159091048,37.03,-44.922659232468));
#39893=CARTESIAN_POINT('',(-5.33658159091048,37.03,-44.922659232468));
#39894=CARTESIAN_POINT('Origin',(-6.10937109726139,37.03,-46.6491775636676));
#39895=CARTESIAN_POINT('',(-6.10937109726139,37.03,-46.6491775636676));
#39896=CARTESIAN_POINT('Origin',(-6.23934797313094,37.03,-47.1789895822776));
#39897=CARTESIAN_POINT('Origin',(-6.22508608057804,37.03,-48.9288433214812));
#39898=CARTESIAN_POINT('',(-6.22508608057804,37.03,-48.9288433214812));
#39899=CARTESIAN_POINT('Origin',(-6.11953090492364,37.03,-49.5434791025604));
#39900=CARTESIAN_POINT('',(-6.11953090492364,37.03,-49.5434791025604));
#39901=CARTESIAN_POINT('Origin',(-5.96800847194436,37.03,-50.1683011437039));
#39902=CARTESIAN_POINT('',(-5.96800847194436,37.03,-50.1683011437039));
#39903=CARTESIAN_POINT('Origin',(-5.7715728030933,37.03,-50.8007214335911));
#39904=CARTESIAN_POINT('',(-5.7715728030933,37.03,-50.8007214335911));
#39905=CARTESIAN_POINT('Origin',(-5.53089056659976,37.03,-51.4383228505279));
#39906=CARTESIAN_POINT('',(-5.53089056659976,37.03,-51.4383228505279));
#39907=CARTESIAN_POINT('Origin',(-5.25715540570604,37.03,-51.518229317088));
#39908=CARTESIAN_POINT('',(-5.25715540570604,37.03,-51.518229317088));
#39909=CARTESIAN_POINT('Origin',(-4.98226661822352,37.03,-51.5940721560646));
#39910=CARTESIAN_POINT('',(-4.98226661822352,37.03,-51.5940721560646));
#39911=CARTESIAN_POINT('Origin',(-4.70628452555985,37.03,-51.6658347245569));
#39912=CARTESIAN_POINT('',(-4.70628452555985,37.03,-51.6658347245569));
#39913=CARTESIAN_POINT('Origin',(-4.42926968903682,37.03,-51.7335012750361));
#39914=CARTESIAN_POINT('',(-4.42926968903682,37.03,-51.7335012750361));
#39915=CARTESIAN_POINT('Origin',(-3.90203204952539,37.03,-51.3016633687267));
#39916=CARTESIAN_POINT('',(-3.90203204952539,37.03,-51.3016633687267));
#39917=CARTESIAN_POINT('Origin',(-3.41570362514739,37.03,-50.8521891662412));
#39918=CARTESIAN_POINT('',(-3.41570362514739,37.03,-50.8521891662412));
#39919=CARTESIAN_POINT('Origin',(-2.97207032837234,37.03,-50.3868386222561));
#39920=CARTESIAN_POINT('',(-2.97207032837234,37.03,-50.3868386222561));
#39921=CARTESIAN_POINT('Origin',(-2.57333897421511,37.03,-49.9073260095938));
#39922=CARTESIAN_POINT('',(-2.57333897421511,37.03,-49.9073260095938));
#39923=CARTESIAN_POINT('Origin',(-2.22248159767726,37.03,-49.4152802505257));
#39924=CARTESIAN_POINT('',(-2.22248159767726,37.03,-49.4152802505257));
#39925=CARTESIAN_POINT('Origin',(-1.92399462146589,37.03,-48.9121625074333));
#39926=CARTESIAN_POINT('',(-1.92399462146589,37.03,-48.9121625074333));
#39927=CARTESIAN_POINT('Origin',(-1.68606094335648,37.03,-48.3990391648128));
#39928=CARTESIAN_POINT('Origin',(-2.4980018054066E-15,37.03,-46.0625));
#39929=CARTESIAN_POINT('',(-2.39954232207934E-15,37.03,-46.0625));
#39930=CARTESIAN_POINT('Origin',(1.33971438913717,37.03,-45.9936165714376));
#39931=CARTESIAN_POINT('',(1.33971438913717,37.03,-45.9936165714376));
#39932=CARTESIAN_POINT('Origin',(1.53371821045902,37.03,-47.8752200595314));
#39933=CARTESIAN_POINT('',(1.53371821045902,37.03,-47.8752200595314));
#39934=CARTESIAN_POINT('Origin',(1.68606094335647,37.03,-48.3990391648128));
#39935=CARTESIAN_POINT('Origin',(2.57333897421511,37.03,-49.9073260095938));
#39936=CARTESIAN_POINT('',(2.57333897421511,37.03,-49.9073260095938));
#39937=CARTESIAN_POINT('Origin',(2.97207032837233,37.03,-50.3868386222561));
#39938=CARTESIAN_POINT('',(2.97207032837233,37.03,-50.3868386222561));
#39939=CARTESIAN_POINT('Origin',(3.41570362514738,37.03,-50.8521891662412));
#39940=CARTESIAN_POINT('',(3.41570362514738,37.03,-50.8521891662412));
#39941=CARTESIAN_POINT('Origin',(3.90203204952538,37.03,-51.3016633687267));
#39942=CARTESIAN_POINT('',(3.90203204952538,37.03,-51.3016633687267));
#39943=CARTESIAN_POINT('Origin',(4.42926968903682,37.03,-51.7335012750361));
#39944=CARTESIAN_POINT('',(4.42926968903682,37.03,-51.7335012750361));
#39945=CARTESIAN_POINT('Origin',(4.70628452555985,37.03,-51.6658347245569));
#39946=CARTESIAN_POINT('',(4.70628452555985,37.03,-51.6658347245569));
#39947=CARTESIAN_POINT('Origin',(4.98226661822352,37.03,-51.5940721560646));
#39948=CARTESIAN_POINT('',(4.98226661822352,37.03,-51.5940721560646));
#39949=CARTESIAN_POINT('Origin',(5.25715540570603,37.03,-51.518229317088));
#39950=CARTESIAN_POINT('',(5.25715540570603,37.03,-51.518229317088));
#39951=CARTESIAN_POINT('Origin',(5.53089056659975,37.03,-51.4383228505279));
#39952=CARTESIAN_POINT('',(5.53089056659975,37.03,-51.4383228505279));
#39953=CARTESIAN_POINT('Origin',(5.77157280309329,37.03,-50.8007214335911));
#39954=CARTESIAN_POINT('',(5.77157280309329,37.03,-50.8007214335911));
#39955=CARTESIAN_POINT('Origin',(5.96800847194436,37.03,-50.1683011437039));
#39956=CARTESIAN_POINT('',(5.96800847194436,37.03,-50.1683011437039));
#39957=CARTESIAN_POINT('Origin',(6.11953090492363,37.03,-49.5434791025604));
#39958=CARTESIAN_POINT('',(6.11953090492363,37.03,-49.5434791025604));
#39959=CARTESIAN_POINT('Origin',(6.22508608057804,37.03,-48.9288433214812));
#39960=CARTESIAN_POINT('',(6.22508608057804,37.03,-48.9288433214812));
#39961=CARTESIAN_POINT('Origin',(6.2829146022309,37.03,-48.3272905060348));
#39962=CARTESIAN_POINT('',(6.2829146022309,37.03,-48.3272905060348));
#39963=CARTESIAN_POINT('Origin',(6.28985303478254,37.03,-47.7423342713165));
#39964=CARTESIAN_POINT('',(6.28985303478254,37.03,-47.7423342713165));
#39965=CARTESIAN_POINT('Origin',(6.23934797313093,37.03,-47.1789895822776));
#39966=CARTESIAN_POINT('Origin',(6.53125,37.03,-44.3124568369342));
#39967=CARTESIAN_POINT('',(6.53125,37.03,-44.3124568369342));
#39968=CARTESIAN_POINT('Origin',(7.65703498052716,37.03,-43.5829448433309));
#39969=CARTESIAN_POINT('',(7.65703498052716,37.03,-43.5829448433309));
#39970=CARTESIAN_POINT('Origin',(8.76584896227005,37.03,-45.1154593532086));
#39971=CARTESIAN_POINT('',(8.76584896227005,37.03,-45.1154593532086));
#39972=CARTESIAN_POINT('Origin',(9.15969119168186,37.03,-45.4929286389212));
#39973=CARTESIAN_POINT('Origin',(10.6822399290158,37.03,-46.3555043472661));
#39974=CARTESIAN_POINT('',(10.6822399290158,37.03,-46.3555043472661));
#39975=CARTESIAN_POINT('Origin',(11.2673077173324,37.03,-46.571408774188));
#39976=CARTESIAN_POINT('',(11.2673077173324,37.03,-46.571408774188));
#39977=CARTESIAN_POINT('Origin',(11.8841806942968,37.03,-46.7525975185565));
#39978=CARTESIAN_POINT('',(11.8841806942968,37.03,-46.7525975185565));
#39979=CARTESIAN_POINT('Origin',(12.5300905656334,37.03,-46.8986893840657));
#39980=CARTESIAN_POINT('',(12.5300905656334,37.03,-46.8986893840657));
#39981=CARTESIAN_POINT('Origin',(13.2026107084363,37.03,-47.009053161491));
#39982=CARTESIAN_POINT('',(13.2026107084363,37.03,-47.009053161491));
#39983=CARTESIAN_POINT('Origin',(13.4086793188509,37.03,-46.8119447915281));
#39984=CARTESIAN_POINT('',(13.4086793188509,37.03,-46.8119447915281));
#39985=CARTESIAN_POINT('Origin',(13.611805537841,37.03,-46.6118055378411));
#39986=CARTESIAN_POINT('',(13.611805537841,37.03,-46.6118055378411));
#39987=CARTESIAN_POINT('Origin',(13.8119447915281,37.03,-46.4086793188509));
#39988=CARTESIAN_POINT('',(13.8119447915281,37.03,-46.4086793188509));
#39989=CARTESIAN_POINT('Origin',(14.009053161491,37.03,-46.2026107084364));
#39990=CARTESIAN_POINT('',(14.009053161491,37.03,-46.2026107084364));
#39991=CARTESIAN_POINT('Origin',(13.8986893840657,37.03,-45.5300905656334));
#39992=CARTESIAN_POINT('',(13.8986893840657,37.03,-45.5300905656334));
#39993=CARTESIAN_POINT('Origin',(13.7525975185565,37.03,-44.8841806942968));
#39994=CARTESIAN_POINT('',(13.7525975185565,37.03,-44.8841806942968));
#39995=CARTESIAN_POINT('Origin',(13.571408774188,37.03,-44.2673077173324));
#39996=CARTESIAN_POINT('',(13.571408774188,37.03,-44.2673077173324));
#39997=CARTESIAN_POINT('Origin',(13.3555043472661,37.03,-43.6822399290158));
#39998=CARTESIAN_POINT('',(13.3555043472661,37.03,-43.6822399290158));
#39999=CARTESIAN_POINT('Origin',(13.1048089083576,37.03,-43.1323656482948));
#40000=CARTESIAN_POINT('',(13.1048089083576,37.03,-43.1323656482948));
#40001=CARTESIAN_POINT('Origin',(12.8183396498506,37.03,-42.6223094726507));
#40002=CARTESIAN_POINT('',(12.8183396498506,37.03,-42.6223094726507));
#40003=CARTESIAN_POINT('Origin',(12.4929286389212,37.03,-42.1596911916819));
#40004=CARTESIAN_POINT('Origin',(11.3124568369342,37.03,-39.53125));
#40005=CARTESIAN_POINT('',(11.3124568369342,37.03,-39.53125));
#40006=CARTESIAN_POINT('Origin',(11.922659232468,37.03,-38.3365815909105));
#40007=CARTESIAN_POINT('',(11.922659232468,37.03,-38.3365815909105));
#40008=CARTESIAN_POINT('Origin',(13.6491775636676,37.03,-39.1093710972614));
#40009=CARTESIAN_POINT('',(13.6491775636676,37.03,-39.1093710972614));
#40010=CARTESIAN_POINT('Origin',(14.1789895822776,37.03,-39.2393479731309));
#40011=CARTESIAN_POINT('Origin',(15.9288433214812,37.03,-39.225086080578));
#40012=CARTESIAN_POINT('',(15.9288433214812,37.03,-39.225086080578));
#40013=CARTESIAN_POINT('Origin',(16.5434791025604,37.03,-39.1195309049236));
#40014=CARTESIAN_POINT('',(16.5434791025604,37.03,-39.1195309049236));
#40015=CARTESIAN_POINT('Origin',(17.1683011437039,37.03,-38.9680084719444));
#40016=CARTESIAN_POINT('',(17.1683011437039,37.03,-38.9680084719444));
#40017=CARTESIAN_POINT('Origin',(17.8007214335911,37.03,-38.7715728030933));
#40018=CARTESIAN_POINT('',(17.8007214335911,37.03,-38.7715728030933));
#40019=CARTESIAN_POINT('Origin',(18.4383228505279,37.03,-38.5308905665998));
#40020=CARTESIAN_POINT('',(18.4383228505279,37.03,-38.5308905665998));
#40021=CARTESIAN_POINT('Origin',(18.518229317088,37.03,-38.257155405706));
#40022=CARTESIAN_POINT('',(18.518229317088,37.03,-38.257155405706));
#40023=CARTESIAN_POINT('Origin',(18.5940721560646,37.03,-37.9822666182235));
#40024=CARTESIAN_POINT('',(18.5940721560646,37.03,-37.9822666182235));
#40025=CARTESIAN_POINT('Origin',(18.6658347245569,37.03,-37.7062845255599));
#40026=CARTESIAN_POINT('',(18.6658347245569,37.03,-37.7062845255599));
#40027=CARTESIAN_POINT('Origin',(18.7335012750361,37.03,-37.4292696890368));
#40028=CARTESIAN_POINT('',(18.7335012750361,37.03,-37.4292696890368));
#40029=CARTESIAN_POINT('Origin',(18.3016633687267,37.03,-36.9020320495254));
#40030=CARTESIAN_POINT('',(18.3016633687267,37.03,-36.9020320495254));
#40031=CARTESIAN_POINT('Origin',(17.8521891662412,37.03,-36.4157036251474));
#40032=CARTESIAN_POINT('',(17.8521891662412,37.03,-36.4157036251474));
#40033=CARTESIAN_POINT('Origin',(17.3868386222561,37.03,-35.9720703283723));
#40034=CARTESIAN_POINT('',(17.3868386222561,37.03,-35.9720703283723));
#40035=CARTESIAN_POINT('Origin',(16.9073260095938,37.03,-35.5733389742151));
#40036=CARTESIAN_POINT('',(16.9073260095938,37.03,-35.5733389742151));
#40037=CARTESIAN_POINT('Origin',(16.4152802505257,37.03,-35.2224815976773));
#40038=CARTESIAN_POINT('',(16.4152802505257,37.03,-35.2224815976773));
#40039=CARTESIAN_POINT('Origin',(15.9121625074333,37.03,-34.9239946214659));
#40040=CARTESIAN_POINT('',(15.9121625074333,37.03,-34.9239946214659));
#40041=CARTESIAN_POINT('Origin',(15.3990391648128,37.03,-34.6860609433565));
#40042=CARTESIAN_POINT('Origin',(13.0625,37.03,-33.));
#40043=CARTESIAN_POINT('',(13.0625,37.03,-33.));
#40044=CARTESIAN_POINT('Origin',(12.9936165714376,37.03,-31.6602856108628));
#40045=CARTESIAN_POINT('',(12.9936165714376,37.03,-31.6602856108628));
#40046=CARTESIAN_POINT('Origin',(14.8752200595314,37.03,-31.466281789541));
#40047=CARTESIAN_POINT('',(14.8752200595314,37.03,-31.466281789541));
#40048=CARTESIAN_POINT('Origin',(15.3990391648128,37.03,-31.3139390566435));
#40049=CARTESIAN_POINT('Origin',(16.9073260095938,37.03,-30.4266610257849));
#40050=CARTESIAN_POINT('',(16.9073260095938,37.03,-30.4266610257849));
#40051=CARTESIAN_POINT('Origin',(17.3868386222561,37.03,-30.0279296716277));
#40052=CARTESIAN_POINT('',(17.3868386222561,37.03,-30.0279296716277));
#40053=CARTESIAN_POINT('Origin',(17.8521891662412,37.03,-29.5842963748526));
#40054=CARTESIAN_POINT('',(17.8521891662412,37.03,-29.5842963748526));
#40055=CARTESIAN_POINT('Origin',(18.3016633687267,37.03,-29.0979679504746));
#40056=CARTESIAN_POINT('',(18.3016633687267,37.03,-29.0979679504746));
#40057=CARTESIAN_POINT('Origin',(18.7335012750361,37.03,-28.5707303109632));
#40058=CARTESIAN_POINT('',(18.7335012750361,37.03,-28.5707303109632));
#40059=CARTESIAN_POINT('Origin',(18.6658347245569,37.03,-28.2937154744402));
#40060=CARTESIAN_POINT('',(18.6658347245569,37.03,-28.2937154744402));
#40061=CARTESIAN_POINT('Origin',(18.5940721560646,37.03,-28.0177333817765));
#40062=CARTESIAN_POINT('',(18.5940721560646,37.03,-28.0177333817765));
#40063=CARTESIAN_POINT('Origin',(18.518229317088,37.03,-27.742844594294));
#40064=CARTESIAN_POINT('',(18.518229317088,37.03,-27.742844594294));
#40065=CARTESIAN_POINT('Origin',(18.4383228505279,37.03,-27.4691094334002));
#40066=CARTESIAN_POINT('',(18.4383228505279,37.03,-27.4691094334002));
#40067=CARTESIAN_POINT('Origin',(17.8007214335911,37.03,-27.2284271969067));
#40068=CARTESIAN_POINT('',(17.8007214335911,37.03,-27.2284271969067));
#40069=CARTESIAN_POINT('Origin',(17.1683011437039,37.03,-27.0319915280556));
#40070=CARTESIAN_POINT('',(17.1683011437039,37.03,-27.0319915280556));
#40071=CARTESIAN_POINT('Origin',(16.5434791025604,37.03,-26.8804690950764));
#40072=CARTESIAN_POINT('',(16.5434791025604,37.03,-26.8804690950764));
#40073=CARTESIAN_POINT('Origin',(15.9288433214812,37.03,-26.774913919422));
#40074=CARTESIAN_POINT('',(15.9288433214812,37.03,-26.774913919422));
#40075=CARTESIAN_POINT('Origin',(15.3272905060348,37.03,-26.7170853977691));
#40076=CARTESIAN_POINT('',(15.3272905060348,37.03,-26.7170853977691));
#40077=CARTESIAN_POINT('Origin',(14.7423342713165,37.03,-26.7101469652175));
#40078=CARTESIAN_POINT('',(14.7423342713165,37.03,-26.7101469652175));
#40079=CARTESIAN_POINT('Origin',(14.1789895822776,37.03,-26.7606520268691));
#40080=CARTESIAN_POINT('Origin',(11.3124568369342,37.03,-26.46875));
#40081=CARTESIAN_POINT('',(11.3124568369342,37.03,-26.46875));
#40082=CARTESIAN_POINT('Origin',(10.5829448433309,37.03,-25.3429650194728));
#40083=CARTESIAN_POINT('',(10.5829448433309,37.03,-25.3429650194728));
#40084=CARTESIAN_POINT('Origin',(12.1154593532086,37.03,-24.23415103773));
#40085=CARTESIAN_POINT('',(12.1154593532086,37.03,-24.23415103773));
#40086=CARTESIAN_POINT('Origin',(12.4929286389212,37.03,-23.8403088083181));
#40087=CARTESIAN_POINT('Origin',(13.3555043472661,37.03,-22.3177600709842));
#40088=CARTESIAN_POINT('',(13.3555043472661,37.03,-22.3177600709842));
#40089=CARTESIAN_POINT('Origin',(13.571408774188,37.03,-21.7326922826676));
#40090=CARTESIAN_POINT('',(13.571408774188,37.03,-21.7326922826676));
#40091=CARTESIAN_POINT('Origin',(13.7525975185565,37.03,-21.1158193057032));
#40092=CARTESIAN_POINT('',(13.7525975185565,37.03,-21.1158193057032));
#40093=CARTESIAN_POINT('Origin',(13.8986893840657,37.03,-20.4699094343666));
#40094=CARTESIAN_POINT('',(13.8986893840657,37.03,-20.4699094343666));
#40095=CARTESIAN_POINT('Origin',(14.009053161491,37.03,-19.7973892915637));
#40096=CARTESIAN_POINT('',(14.009053161491,37.03,-19.7973892915637));
#40097=CARTESIAN_POINT('Origin',(13.8119447915281,37.03,-19.5913206811491));
#40098=CARTESIAN_POINT('',(13.8119447915281,37.03,-19.5913206811491));
#40099=CARTESIAN_POINT('Origin',(13.611805537841,37.03,-19.388194462159));
#40100=CARTESIAN_POINT('',(13.611805537841,37.03,-19.388194462159));
#40101=CARTESIAN_POINT('Origin',(13.4086793188509,37.03,-19.1880552084719));
#40102=CARTESIAN_POINT('',(13.4086793188509,37.03,-19.1880552084719));
#40103=CARTESIAN_POINT('Origin',(13.2026107084364,37.03,-18.990946838509));
#40104=CARTESIAN_POINT('',(13.2026107084364,37.03,-18.990946838509));
#40105=CARTESIAN_POINT('Origin',(12.5300905656334,37.03,-19.1013106159343));
#40106=CARTESIAN_POINT('',(12.5300905656334,37.03,-19.1013106159343));
#40107=CARTESIAN_POINT('Origin',(11.8841806942968,37.03,-19.2474024814435));
#40108=CARTESIAN_POINT('',(11.8841806942968,37.03,-19.2474024814435));
#40109=CARTESIAN_POINT('Origin',(11.2673077173324,37.03,-19.428591225812));
#40110=CARTESIAN_POINT('',(11.2673077173324,37.03,-19.428591225812));
#40111=CARTESIAN_POINT('Origin',(10.6822399290158,37.03,-19.6444956527339));
#40112=CARTESIAN_POINT('',(10.6822399290158,37.03,-19.6444956527339));
#40113=CARTESIAN_POINT('Origin',(10.1323656482948,37.03,-19.8951910916424));
#40114=CARTESIAN_POINT('',(10.1323656482948,37.03,-19.8951910916424));
#40115=CARTESIAN_POINT('Origin',(9.62230947265072,37.03,-20.1816603501494));
#40116=CARTESIAN_POINT('',(9.62230947265072,37.03,-20.1816603501494));
#40117=CARTESIAN_POINT('Origin',(9.15969119168187,37.03,-20.5070713610788));
#40118=CARTESIAN_POINT('Origin',(6.53125,37.03,-21.6875431630658));
#40119=CARTESIAN_POINT('Origin',(0.,51.,-33.));
#40120=CARTESIAN_POINT('',(-1.04094977927525E-15,18.05,-41.5));
#40121=CARTESIAN_POINT('',(-1.04094977927525E-15,51.,-41.5));
#40122=CARTESIAN_POINT('Origin',(0.,18.05,-33.));
#40123=CARTESIAN_POINT('Origin',(0.,18.05,-24.5));
#40124=CARTESIAN_POINT('Origin',(0.,51.,-33.));
#40125=CARTESIAN_POINT('',(-1.04094977927525E-15,83.95,-41.5));
#40126=CARTESIAN_POINT('Origin',(0.,83.95,-33.));
#40127=CARTESIAN_POINT('',(-1.04094977927525E-15,51.,-41.5));
#40128=CARTESIAN_POINT('Origin',(0.,83.95,-33.));
#46369=UNCERTAINTY_MEASURE_WITH_UNIT(LENGTH_MEASURE(0.01),#46396,
'DISTANCE_ACCURACY_VALUE',
'Maximum model space distance between geometric entities at asserted c
onnectivities');
#46379=UNCERTAINTY_MEASURE_WITH_UNIT(LENGTH_MEASURE(0.01),#46396,
'DISTANCE_ACCURACY_VALUE',
'Maximum model space distance between geometric entities at asserted c
onnectivities');
#46385=(
GEOMETRIC_REPRESENTATION_CONTEXT(3)
GLOBAL_UNCERTAINTY_ASSIGNED_CONTEXT((#46369))
GLOBAL_UNIT_ASSIGNED_CONTEXT((#46396,#46398,#46399))
REPRESENTATION_CONTEXT('','3D')
);
#46395=(
GEOMETRIC_REPRESENTATION_CONTEXT(3)
GLOBAL_UNCERTAINTY_ASSIGNED_CONTEXT((#46379))
GLOBAL_UNIT_ASSIGNED_CONTEXT((#46396,#46398,#46399))
REPRESENTATION_CONTEXT('','3D')
);
#46396=(
LENGTH_UNIT()
NAMED_UNIT(*)
SI_UNIT(.MILLI.,.METRE.)
);
#46398=(
NAMED_UNIT(*)
PLANE_ANGLE_UNIT()
SI_UNIT($,.RADIAN.)
);
#46399=(
NAMED_UNIT(*)
SI_UNIT($,.STERADIAN.)
SOLID_ANGLE_UNIT()
);
#46405=SHAPE_DEFINITION_REPRESENTATION(#46420,#46460);
#46420=PRODUCT_DEFINITION_SHAPE('',$,#46476);
#46460=SHAPE_REPRESENTATION('',(#26063),#46385);
#46470=PRODUCT_DEFINITION_CONTEXT('part definition',#46517,'design');
#46476=PRODUCT_DEFINITION('2026-10-26-00-50-58-441',
'05_Driven_Gear_Shaft_z12_m2.75',#46491,#46470);
#46491=PRODUCT_DEFINITION_FORMATION('',$,#46524);
#46517=APPLICATION_CONTEXT(
'Core Data for Automotive Mechanical Design Process');
#46518=PRODUCT_CONTEXT('part definition',#46517,'mechanical');
#46524=PRODUCT('2026-10-26-00-50-58-441',
'05_Driven_Gear_Shaft_z12_m2.75',$,(#46518));
#46590=COLOUR_RGB('Grey',0.48,0.52,0.57);
#46591=FILL_AREA_STYLE_COLOUR('',#46590);
#46592=FILL_AREA_STYLE('',(#46591));
#46593=SURFACE_STYLE_FILL_AREA(#46592);
#46594=SURFACE_SIDE_STYLE('',(#46593));
#46595=SURFACE_STYLE_USAGE(.BOTH.,#46594);
#46596=PRESENTATION_STYLE_ASSIGNMENT((#46595));
ENDSEC;
END-ISO-10303-21;
